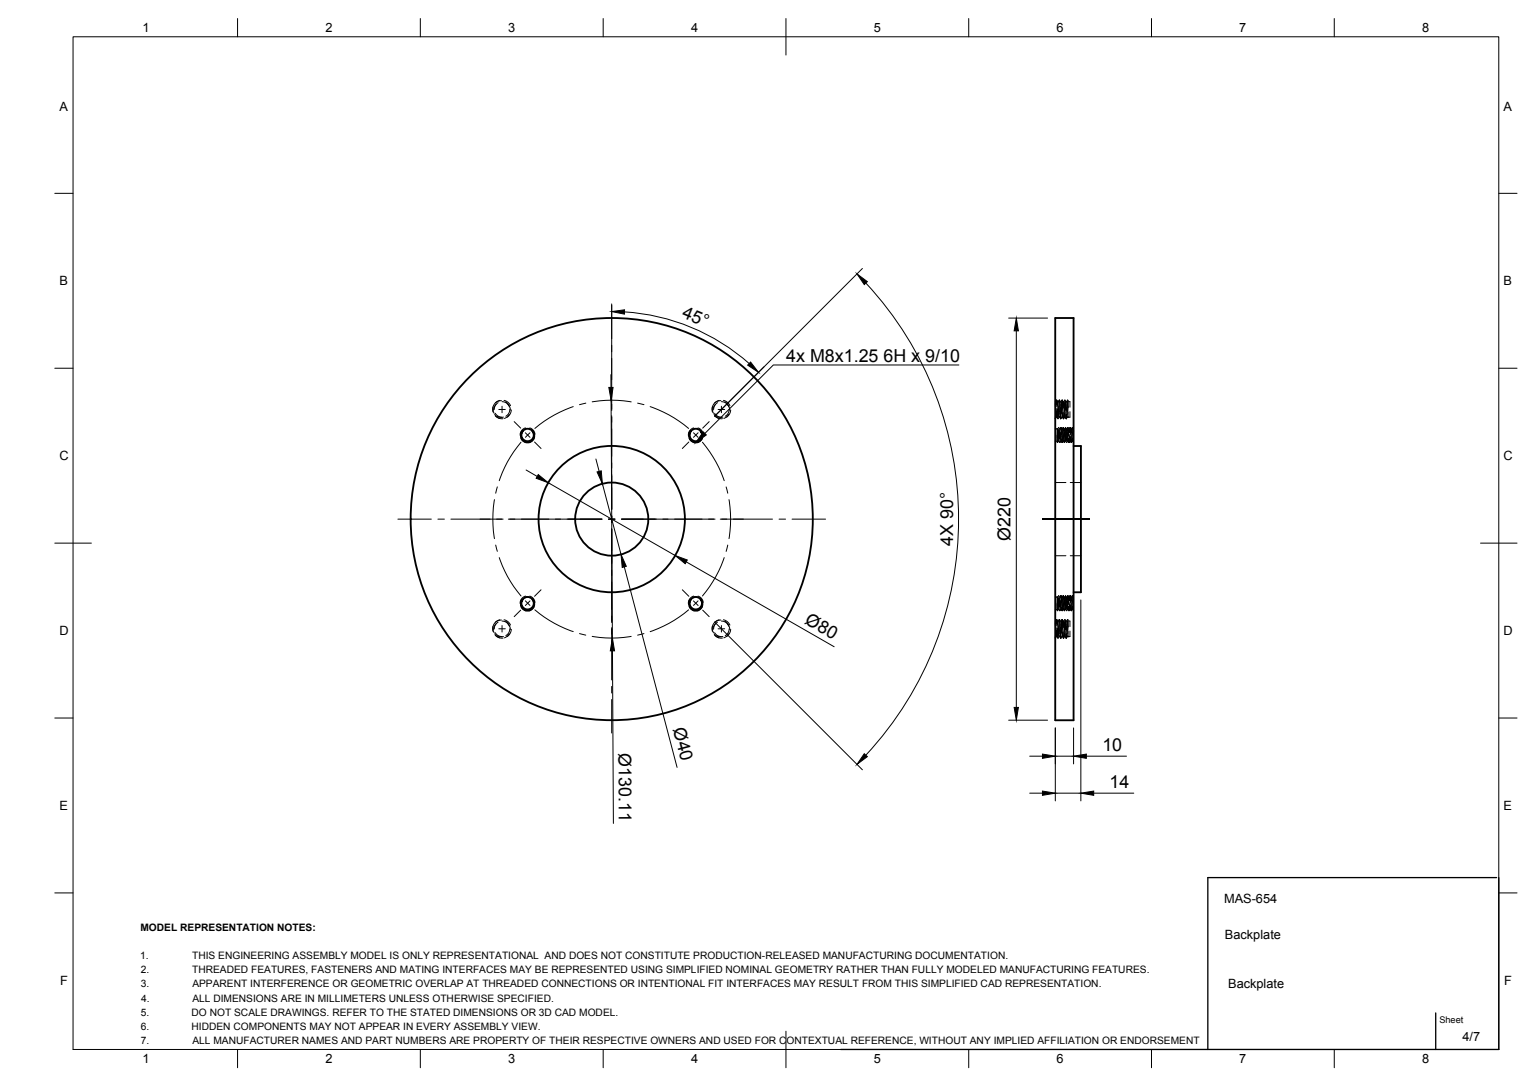
ISO-10303-21;
HEADER;
/* Generated by software containing ST-Developer
 * from STEP Tools, Inc. (www.steptools.com) 
 */

FILE_DESCRIPTION(
/* description */ ('Independent four-jaw lathe chuck,200mm body,40mm bore,36\X2\2013\X0\7
6mm nominal opposed jaw opening. Four shared machined T-jaws and model
ed partial M12x1.75 feed screws, native independent screw/slider links
, removable bolted bronze-bearing cartridges, fully captured ring/wash
er/head thrust stacks and registered bolted backplate. Custom spindle 
interface; no compatibility, speed, grip force or safety rating assign
ed.'),
/* implementation_level */ '2;1');

FILE_NAME(
/* name */ 'Backplate.step',
/* time_stamp */ '2026-11-09T20:24:54-08:00',
/* author */ (''),
/* organization */ (''),
/* preprocessor_version */ 'ST-DEVELOPER v20.2',
/* originating_system */ 'Autodesk Translation Framework v15.17.0.0',
/* authorisation */ '');

FILE_SCHEMA (('AUTOMOTIVE_DESIGN { 1 0 10303 214 3 1 1 }'));
ENDSEC;

DATA;
#10=MECHANICAL_DESIGN_GEOMETRIC_PRESENTATION_REPRESENTATION('',(#237),#69491);
#215=SHAPE_REPRESENTATION_RELATIONSHIP('SRR','None',#69572,#226);
#226=ADVANCED_BREP_SHAPE_REPRESENTATION('',(#248),#69481);
#237=STYLED_ITEM('',(#69636),#248);
#248=MANIFOLD_SOLID_BREP('Body1',#14732);
#274=B_SPLINE_SURFACE_WITH_KNOTS('',3,3,((#35745,#35746,#35747,#35748,#35749,
#35750,#35751,#35752,#35753,#35754,#35755,#35756,#35757,#35758,#35759,#35760,
#35761,#35762,#35763,#35764,#35765,#35766,#35767,#35768,#35769,#35770,#35771,
#35772,#35773,#35774,#35775,#35776,#35777,#35778,#35779,#35780,#35781,#35782,
#35783,#35784,#35785,#35786,#35787,#35788,#35789,#35790,#35791,#35792,#35793,
#35794,#35795,#35796,#35797,#35798,#35799,#35800,#35801,#35802,#35803,#35804,
#35805,#35806,#35807,#35808),(#35809,#35810,#35811,#35812,#35813,#35814,
#35815,#35816,#35817,#35818,#35819,#35820,#35821,#35822,#35823,#35824,#35825,
#35826,#35827,#35828,#35829,#35830,#35831,#35832,#35833,#35834,#35835,#35836,
#35837,#35838,#35839,#35840,#35841,#35842,#35843,#35844,#35845,#35846,#35847,
#35848,#35849,#35850,#35851,#35852,#35853,#35854,#35855,#35856,#35857,#35858,
#35859,#35860,#35861,#35862,#35863,#35864,#35865,#35866,#35867,#35868,#35869,
#35870,#35871,#35872),(#35873,#35874,#35875,#35876,#35877,#35878,#35879,
#35880,#35881,#35882,#35883,#35884,#35885,#35886,#35887,#35888,#35889,#35890,
#35891,#35892,#35893,#35894,#35895,#35896,#35897,#35898,#35899,#35900,#35901,
#35902,#35903,#35904,#35905,#35906,#35907,#35908,#35909,#35910,#35911,#35912,
#35913,#35914,#35915,#35916,#35917,#35918,#35919,#35920,#35921,#35922,#35923,
#35924,#35925,#35926,#35927,#35928,#35929,#35930,#35931,#35932,#35933,#35934,
#35935,#35936),(#35937,#35938,#35939,#35940,#35941,#35942,#35943,#35944,
#35945,#35946,#35947,#35948,#35949,#35950,#35951,#35952,#35953,#35954,#35955,
#35956,#35957,#35958,#35959,#35960,#35961,#35962,#35963,#35964,#35965,#35966,
#35967,#35968,#35969,#35970,#35971,#35972,#35973,#35974,#35975,#35976,#35977,
#35978,#35979,#35980,#35981,#35982,#35983,#35984,#35985,#35986,#35987,#35988,
#35989,#35990,#35991,#35992,#35993,#35994,#35995,#35996,#35997,#35998,#35999,
#36000)),.UNSPECIFIED.,.F.,.F.,.F.,(4,4),(4,1,1,1,1,1,1,1,1,1,1,1,1,1,1,
1,1,1,1,1,1,1,1,1,1,1,1,1,1,1,1,1,1,1,1,1,1,1,1,1,1,1,1,1,1,1,1,1,1,1,1,
1,1,1,1,1,1,1,1,1,1,4),(0.,0.0965329650085053),(11.8529428644271,12.3426821320026,
12.8324213995782,13.3221606671538,13.8118999347294,14.301639202305,14.7913784698806,
15.2811177374562,15.7708570050318,16.2605962726074,16.750335540183,17.2400748077586,
17.7298140753341,18.2195533429097,18.7092926104853,19.1990318780609,19.6887711456365,
20.1785104132121,20.6682496807877,21.1579889483633,21.6477282159389,22.1374674835145,
22.6272067510901,23.1169460186656,23.6066852862412,24.0964245538168,24.5861638213924,
25.075903088968,25.5656423565436,26.0553816241192,26.5451208916948,27.524599426846,
28.5040779619971,29.4835564971483,29.9732957647239,30.4630350322995,30.9527742998751,
31.4425135674507,31.9322528350263,32.4219921026019,32.9117313701775,33.4014706377531,
33.8912099053287,34.3809491729042,34.8706884404798,35.3604277080554,35.850166975631,
36.3399062432066,36.8296455107822,37.3193847783578,37.8091240459334,38.298863313509,
38.7886025810846,39.2783418486601,39.7680811162357,40.2578203838113,40.7475596513869,
41.2372989189625,41.7270381865381,42.2167774541137,42.7065167216893,43.1962559892649),
 .UNSPECIFIED.);
#275=B_SPLINE_SURFACE_WITH_KNOTS('',3,3,((#36150,#36151,#36152,#36153,#36154,
#36155,#36156,#36157,#36158,#36159,#36160,#36161,#36162,#36163,#36164,#36165,
#36166,#36167,#36168,#36169,#36170,#36171,#36172,#36173,#36174,#36175,#36176,
#36177,#36178,#36179,#36180,#36181,#36182,#36183,#36184,#36185,#36186,#36187,
#36188,#36189,#36190,#36191,#36192,#36193,#36194,#36195,#36196,#36197,#36198,
#36199,#36200,#36201,#36202,#36203,#36204,#36205,#36206,#36207,#36208,#36209,
#36210,#36211,#36212,#36213),(#36214,#36215,#36216,#36217,#36218,#36219,
#36220,#36221,#36222,#36223,#36224,#36225,#36226,#36227,#36228,#36229,#36230,
#36231,#36232,#36233,#36234,#36235,#36236,#36237,#36238,#36239,#36240,#36241,
#36242,#36243,#36244,#36245,#36246,#36247,#36248,#36249,#36250,#36251,#36252,
#36253,#36254,#36255,#36256,#36257,#36258,#36259,#36260,#36261,#36262,#36263,
#36264,#36265,#36266,#36267,#36268,#36269,#36270,#36271,#36272,#36273,#36274,
#36275,#36276,#36277),(#36278,#36279,#36280,#36281,#36282,#36283,#36284,
#36285,#36286,#36287,#36288,#36289,#36290,#36291,#36292,#36293,#36294,#36295,
#36296,#36297,#36298,#36299,#36300,#36301,#36302,#36303,#36304,#36305,#36306,
#36307,#36308,#36309,#36310,#36311,#36312,#36313,#36314,#36315,#36316,#36317,
#36318,#36319,#36320,#36321,#36322,#36323,#36324,#36325,#36326,#36327,#36328,
#36329,#36330,#36331,#36332,#36333,#36334,#36335,#36336,#36337,#36338,#36339,
#36340,#36341),(#36342,#36343,#36344,#36345,#36346,#36347,#36348,#36349,
#36350,#36351,#36352,#36353,#36354,#36355,#36356,#36357,#36358,#36359,#36360,
#36361,#36362,#36363,#36364,#36365,#36366,#36367,#36368,#36369,#36370,#36371,
#36372,#36373,#36374,#36375,#36376,#36377,#36378,#36379,#36380,#36381,#36382,
#36383,#36384,#36385,#36386,#36387,#36388,#36389,#36390,#36391,#36392,#36393,
#36394,#36395,#36396,#36397,#36398,#36399,#36400,#36401,#36402,#36403,#36404,
#36405)),.UNSPECIFIED.,.F.,.F.,.F.,(4,4),(4,1,1,1,1,1,1,1,1,1,1,1,1,1,1,
1,1,1,1,1,1,1,1,1,1,1,1,1,1,1,1,1,1,1,1,1,1,1,1,1,1,1,1,1,1,1,1,1,1,1,1,
1,1,1,1,1,1,1,1,1,1,4),(0.,0.0965329650085053),(14.399609326548,14.8893485941236,
15.3790878616992,15.8688271292748,16.3585663968504,16.848305664426,17.3380449320016,
17.8277841995772,18.3175234671527,18.8072627347283,19.2970020023039,19.7867412698795,
20.2764805374551,20.7662198050307,21.2559590726063,21.7456983401819,22.2354376077575,
22.7251768753331,23.2149161429087,23.7046554104842,24.1943946780598,24.6841339456354,
25.173873213211,25.6636124807866,26.1533517483622,26.6430910159378,27.1328302835134,
27.622569551089,28.1123088186646,28.6020480862402,29.0917873538157,30.0712658889669,
31.0507444241181,32.0302229592693,32.5199622268449,33.0097014944205,33.4994407619961,
33.9891800295717,34.4789192971472,34.9686585647228,35.4583978322984,35.948137099874,
36.4378763674496,36.9276156350252,37.4173549026008,37.9070941701764,38.396833437752,
38.8865727053276,39.3763119729032,39.8660512404787,40.3557905080543,40.8455297756299,
41.3352690432055,41.8250083107811,42.3147475783567,42.8044868459323,43.2942261135079,
43.7839653810835,44.2737046486591,44.7634439162347,45.2531831838103,45.7429224513858),
 .UNSPECIFIED.);
#276=B_SPLINE_SURFACE_WITH_KNOTS('',3,3,((#36810,#36811,#36812,#36813,#36814,
#36815,#36816,#36817,#36818,#36819,#36820,#36821,#36822,#36823,#36824,#36825,
#36826,#36827,#36828,#36829,#36830,#36831,#36832,#36833,#36834,#36835,#36836,
#36837,#36838,#36839,#36840,#36841,#36842,#36843,#36844,#36845,#36846,#36847,
#36848,#36849,#36850,#36851,#36852,#36853,#36854,#36855,#36856,#36857,#36858,
#36859,#36860,#36861,#36862,#36863,#36864,#36865,#36866,#36867,#36868,#36869,
#36870,#36871,#36872,#36873),(#36874,#36875,#36876,#36877,#36878,#36879,
#36880,#36881,#36882,#36883,#36884,#36885,#36886,#36887,#36888,#36889,#36890,
#36891,#36892,#36893,#36894,#36895,#36896,#36897,#36898,#36899,#36900,#36901,
#36902,#36903,#36904,#36905,#36906,#36907,#36908,#36909,#36910,#36911,#36912,
#36913,#36914,#36915,#36916,#36917,#36918,#36919,#36920,#36921,#36922,#36923,
#36924,#36925,#36926,#36927,#36928,#36929,#36930,#36931,#36932,#36933,#36934,
#36935,#36936,#36937),(#36938,#36939,#36940,#36941,#36942,#36943,#36944,
#36945,#36946,#36947,#36948,#36949,#36950,#36951,#36952,#36953,#36954,#36955,
#36956,#36957,#36958,#36959,#36960,#36961,#36962,#36963,#36964,#36965,#36966,
#36967,#36968,#36969,#36970,#36971,#36972,#36973,#36974,#36975,#36976,#36977,
#36978,#36979,#36980,#36981,#36982,#36983,#36984,#36985,#36986,#36987,#36988,
#36989,#36990,#36991,#36992,#36993,#36994,#36995,#36996,#36997,#36998,#36999,
#37000,#37001),(#37002,#37003,#37004,#37005,#37006,#37007,#37008,#37009,
#37010,#37011,#37012,#37013,#37014,#37015,#37016,#37017,#37018,#37019,#37020,
#37021,#37022,#37023,#37024,#37025,#37026,#37027,#37028,#37029,#37030,#37031,
#37032,#37033,#37034,#37035,#37036,#37037,#37038,#37039,#37040,#37041,#37042,
#37043,#37044,#37045,#37046,#37047,#37048,#37049,#37050,#37051,#37052,#37053,
#37054,#37055,#37056,#37057,#37058,#37059,#37060,#37061,#37062,#37063,#37064,
#37065)),.UNSPECIFIED.,.F.,.F.,.F.,(4,4),(4,1,1,1,1,1,1,1,1,1,1,1,1,1,1,
1,1,1,1,1,1,1,1,1,1,1,1,1,1,1,1,1,1,1,1,1,1,1,1,1,1,1,1,1,1,1,1,1,1,1,1,
1,1,1,1,1,1,1,1,1,1,4),(0.,0.0965329650085053),(11.8529428644271,12.3426821320026,
12.8324213995782,13.3221606671538,13.8118999347294,14.301639202305,14.7913784698806,
15.2811177374562,15.7708570050318,16.2605962726074,16.750335540183,17.2400748077586,
17.7298140753341,18.2195533429097,18.7092926104853,19.1990318780609,19.6887711456365,
20.1785104132121,20.6682496807877,21.1579889483633,21.6477282159389,22.1374674835145,
22.6272067510901,23.1169460186656,23.6066852862412,24.0964245538168,24.5861638213924,
25.075903088968,25.5656423565436,26.0553816241192,26.5451208916948,27.524599426846,
28.5040779619971,29.4835564971483,29.9732957647239,30.4630350322995,30.9527742998751,
31.4425135674507,31.9322528350263,32.4219921026019,32.9117313701775,33.4014706377531,
33.8912099053287,34.3809491729042,34.8706884404798,35.3604277080554,35.850166975631,
36.3399062432066,36.8296455107822,37.3193847783578,37.8091240459334,38.298863313509,
38.7886025810846,39.2783418486601,39.7680811162357,40.2578203838113,40.7475596513869,
41.2372989189625,41.7270381865381,42.2167774541137,42.7065167216893,43.1962559892649),
 .UNSPECIFIED.);
#277=B_SPLINE_SURFACE_WITH_KNOTS('',3,3,((#37215,#37216,#37217,#37218,#37219,
#37220,#37221,#37222,#37223,#37224,#37225,#37226,#37227,#37228,#37229,#37230,
#37231,#37232,#37233,#37234,#37235,#37236,#37237,#37238,#37239,#37240,#37241,
#37242,#37243,#37244,#37245,#37246,#37247,#37248,#37249,#37250,#37251,#37252,
#37253,#37254,#37255,#37256,#37257,#37258,#37259,#37260,#37261,#37262,#37263,
#37264,#37265,#37266,#37267,#37268,#37269,#37270,#37271,#37272,#37273,#37274,
#37275,#37276,#37277,#37278),(#37279,#37280,#37281,#37282,#37283,#37284,
#37285,#37286,#37287,#37288,#37289,#37290,#37291,#37292,#37293,#37294,#37295,
#37296,#37297,#37298,#37299,#37300,#37301,#37302,#37303,#37304,#37305,#37306,
#37307,#37308,#37309,#37310,#37311,#37312,#37313,#37314,#37315,#37316,#37317,
#37318,#37319,#37320,#37321,#37322,#37323,#37324,#37325,#37326,#37327,#37328,
#37329,#37330,#37331,#37332,#37333,#37334,#37335,#37336,#37337,#37338,#37339,
#37340,#37341,#37342),(#37343,#37344,#37345,#37346,#37347,#37348,#37349,
#37350,#37351,#37352,#37353,#37354,#37355,#37356,#37357,#37358,#37359,#37360,
#37361,#37362,#37363,#37364,#37365,#37366,#37367,#37368,#37369,#37370,#37371,
#37372,#37373,#37374,#37375,#37376,#37377,#37378,#37379,#37380,#37381,#37382,
#37383,#37384,#37385,#37386,#37387,#37388,#37389,#37390,#37391,#37392,#37393,
#37394,#37395,#37396,#37397,#37398,#37399,#37400,#37401,#37402,#37403,#37404,
#37405,#37406),(#37407,#37408,#37409,#37410,#37411,#37412,#37413,#37414,
#37415,#37416,#37417,#37418,#37419,#37420,#37421,#37422,#37423,#37424,#37425,
#37426,#37427,#37428,#37429,#37430,#37431,#37432,#37433,#37434,#37435,#37436,
#37437,#37438,#37439,#37440,#37441,#37442,#37443,#37444,#37445,#37446,#37447,
#37448,#37449,#37450,#37451,#37452,#37453,#37454,#37455,#37456,#37457,#37458,
#37459,#37460,#37461,#37462,#37463,#37464,#37465,#37466,#37467,#37468,#37469,
#37470)),.UNSPECIFIED.,.F.,.F.,.F.,(4,4),(4,1,1,1,1,1,1,1,1,1,1,1,1,1,1,
1,1,1,1,1,1,1,1,1,1,1,1,1,1,1,1,1,1,1,1,1,1,1,1,1,1,1,1,1,1,1,1,1,1,1,1,
1,1,1,1,1,1,1,1,1,1,4),(0.,0.0965329650085053),(14.399609326548,14.8893485941236,
15.3790878616992,15.8688271292748,16.3585663968504,16.848305664426,17.3380449320016,
17.8277841995772,18.3175234671527,18.8072627347283,19.2970020023039,19.7867412698795,
20.2764805374551,20.7662198050307,21.2559590726063,21.7456983401819,22.2354376077575,
22.7251768753331,23.2149161429087,23.7046554104842,24.1943946780598,24.6841339456354,
25.173873213211,25.6636124807866,26.1533517483622,26.6430910159378,27.1328302835134,
27.622569551089,28.1123088186646,28.6020480862402,29.0917873538157,30.0712658889669,
31.0507444241181,32.0302229592693,32.5199622268449,33.0097014944205,33.4994407619961,
33.9891800295717,34.4789192971472,34.9686585647228,35.4583978322984,35.948137099874,
36.4378763674496,36.9276156350252,37.4173549026008,37.9070941701764,38.396833437752,
38.8865727053276,39.3763119729032,39.8660512404787,40.3557905080543,40.8455297756299,
41.3352690432055,41.8250083107811,42.3147475783567,42.8044868459323,43.2942261135079,
43.7839653810835,44.2737046486591,44.7634439162347,45.2531831838103,45.7429224513858),
 .UNSPECIFIED.);
#278=B_SPLINE_SURFACE_WITH_KNOTS('',3,3,((#37875,#37876,#37877,#37878,#37879,
#37880,#37881,#37882,#37883,#37884,#37885,#37886,#37887,#37888,#37889,#37890,
#37891,#37892,#37893,#37894,#37895,#37896,#37897,#37898,#37899,#37900,#37901,
#37902,#37903,#37904,#37905,#37906,#37907,#37908,#37909,#37910,#37911,#37912,
#37913,#37914,#37915,#37916,#37917,#37918,#37919,#37920,#37921,#37922,#37923,
#37924,#37925,#37926,#37927,#37928,#37929,#37930,#37931,#37932,#37933,#37934,
#37935,#37936,#37937,#37938),(#37939,#37940,#37941,#37942,#37943,#37944,
#37945,#37946,#37947,#37948,#37949,#37950,#37951,#37952,#37953,#37954,#37955,
#37956,#37957,#37958,#37959,#37960,#37961,#37962,#37963,#37964,#37965,#37966,
#37967,#37968,#37969,#37970,#37971,#37972,#37973,#37974,#37975,#37976,#37977,
#37978,#37979,#37980,#37981,#37982,#37983,#37984,#37985,#37986,#37987,#37988,
#37989,#37990,#37991,#37992,#37993,#37994,#37995,#37996,#37997,#37998,#37999,
#38000,#38001,#38002),(#38003,#38004,#38005,#38006,#38007,#38008,#38009,
#38010,#38011,#38012,#38013,#38014,#38015,#38016,#38017,#38018,#38019,#38020,
#38021,#38022,#38023,#38024,#38025,#38026,#38027,#38028,#38029,#38030,#38031,
#38032,#38033,#38034,#38035,#38036,#38037,#38038,#38039,#38040,#38041,#38042,
#38043,#38044,#38045,#38046,#38047,#38048,#38049,#38050,#38051,#38052,#38053,
#38054,#38055,#38056,#38057,#38058,#38059,#38060,#38061,#38062,#38063,#38064,
#38065,#38066),(#38067,#38068,#38069,#38070,#38071,#38072,#38073,#38074,
#38075,#38076,#38077,#38078,#38079,#38080,#38081,#38082,#38083,#38084,#38085,
#38086,#38087,#38088,#38089,#38090,#38091,#38092,#38093,#38094,#38095,#38096,
#38097,#38098,#38099,#38100,#38101,#38102,#38103,#38104,#38105,#38106,#38107,
#38108,#38109,#38110,#38111,#38112,#38113,#38114,#38115,#38116,#38117,#38118,
#38119,#38120,#38121,#38122,#38123,#38124,#38125,#38126,#38127,#38128,#38129,
#38130)),.UNSPECIFIED.,.F.,.F.,.F.,(4,4),(4,1,1,1,1,1,1,1,1,1,1,1,1,1,1,
1,1,1,1,1,1,1,1,1,1,1,1,1,1,1,1,1,1,1,1,1,1,1,1,1,1,1,1,1,1,1,1,1,1,1,1,
1,1,1,1,1,1,1,1,1,1,4),(0.,0.0965329650085053),(11.8529428644271,12.3426821320026,
12.8324213995782,13.3221606671538,13.8118999347294,14.301639202305,14.7913784698806,
15.2811177374562,15.7708570050318,16.2605962726074,16.750335540183,17.2400748077586,
17.7298140753341,18.2195533429097,18.7092926104853,19.1990318780609,19.6887711456365,
20.1785104132121,20.6682496807877,21.1579889483633,21.6477282159389,22.1374674835145,
22.6272067510901,23.1169460186656,23.6066852862412,24.0964245538168,24.5861638213924,
25.075903088968,25.5656423565436,26.0553816241192,26.5451208916948,27.524599426846,
28.5040779619971,29.4835564971483,29.9732957647239,30.4630350322995,30.9527742998751,
31.4425135674507,31.9322528350263,32.4219921026019,32.9117313701775,33.4014706377531,
33.8912099053287,34.3809491729042,34.8706884404798,35.3604277080554,35.850166975631,
36.3399062432066,36.8296455107822,37.3193847783578,37.8091240459334,38.298863313509,
38.7886025810846,39.2783418486601,39.7680811162357,40.2578203838113,40.7475596513869,
41.2372989189625,41.7270381865381,42.2167774541137,42.7065167216893,43.1962559892649),
 .UNSPECIFIED.);
#279=B_SPLINE_SURFACE_WITH_KNOTS('',3,3,((#38280,#38281,#38282,#38283,#38284,
#38285,#38286,#38287,#38288,#38289,#38290,#38291,#38292,#38293,#38294,#38295,
#38296,#38297,#38298,#38299,#38300,#38301,#38302,#38303,#38304,#38305,#38306,
#38307,#38308,#38309,#38310,#38311,#38312,#38313,#38314,#38315,#38316,#38317,
#38318,#38319,#38320,#38321,#38322,#38323,#38324,#38325,#38326,#38327,#38328,
#38329,#38330,#38331,#38332,#38333,#38334,#38335,#38336,#38337,#38338,#38339,
#38340,#38341,#38342,#38343),(#38344,#38345,#38346,#38347,#38348,#38349,
#38350,#38351,#38352,#38353,#38354,#38355,#38356,#38357,#38358,#38359,#38360,
#38361,#38362,#38363,#38364,#38365,#38366,#38367,#38368,#38369,#38370,#38371,
#38372,#38373,#38374,#38375,#38376,#38377,#38378,#38379,#38380,#38381,#38382,
#38383,#38384,#38385,#38386,#38387,#38388,#38389,#38390,#38391,#38392,#38393,
#38394,#38395,#38396,#38397,#38398,#38399,#38400,#38401,#38402,#38403,#38404,
#38405,#38406,#38407),(#38408,#38409,#38410,#38411,#38412,#38413,#38414,
#38415,#38416,#38417,#38418,#38419,#38420,#38421,#38422,#38423,#38424,#38425,
#38426,#38427,#38428,#38429,#38430,#38431,#38432,#38433,#38434,#38435,#38436,
#38437,#38438,#38439,#38440,#38441,#38442,#38443,#38444,#38445,#38446,#38447,
#38448,#38449,#38450,#38451,#38452,#38453,#38454,#38455,#38456,#38457,#38458,
#38459,#38460,#38461,#38462,#38463,#38464,#38465,#38466,#38467,#38468,#38469,
#38470,#38471),(#38472,#38473,#38474,#38475,#38476,#38477,#38478,#38479,
#38480,#38481,#38482,#38483,#38484,#38485,#38486,#38487,#38488,#38489,#38490,
#38491,#38492,#38493,#38494,#38495,#38496,#38497,#38498,#38499,#38500,#38501,
#38502,#38503,#38504,#38505,#38506,#38507,#38508,#38509,#38510,#38511,#38512,
#38513,#38514,#38515,#38516,#38517,#38518,#38519,#38520,#38521,#38522,#38523,
#38524,#38525,#38526,#38527,#38528,#38529,#38530,#38531,#38532,#38533,#38534,
#38535)),.UNSPECIFIED.,.F.,.F.,.F.,(4,4),(4,1,1,1,1,1,1,1,1,1,1,1,1,1,1,
1,1,1,1,1,1,1,1,1,1,1,1,1,1,1,1,1,1,1,1,1,1,1,1,1,1,1,1,1,1,1,1,1,1,1,1,
1,1,1,1,1,1,1,1,1,1,4),(0.,0.0965329650085053),(14.399609326548,14.8893485941236,
15.3790878616992,15.8688271292748,16.3585663968504,16.848305664426,17.3380449320016,
17.8277841995772,18.3175234671527,18.8072627347283,19.2970020023039,19.7867412698795,
20.2764805374551,20.7662198050307,21.2559590726063,21.7456983401819,22.2354376077575,
22.7251768753331,23.2149161429087,23.7046554104842,24.1943946780598,24.6841339456354,
25.173873213211,25.6636124807866,26.1533517483622,26.6430910159378,27.1328302835134,
27.622569551089,28.1123088186646,28.6020480862402,29.0917873538157,30.0712658889669,
31.0507444241181,32.0302229592693,32.5199622268449,33.0097014944205,33.4994407619961,
33.9891800295717,34.4789192971472,34.9686585647228,35.4583978322984,35.948137099874,
36.4378763674496,36.9276156350252,37.4173549026008,37.9070941701764,38.396833437752,
38.8865727053276,39.3763119729032,39.8660512404787,40.3557905080543,40.8455297756299,
41.3352690432055,41.8250083107811,42.3147475783567,42.8044868459323,43.2942261135079,
43.7839653810835,44.2737046486591,44.7634439162347,45.2531831838103,45.7429224513858),
 .UNSPECIFIED.);
#280=B_SPLINE_SURFACE_WITH_KNOTS('',3,3,((#38940,#38941,#38942,#38943,#38944,
#38945,#38946,#38947,#38948,#38949,#38950,#38951,#38952,#38953,#38954,#38955,
#38956,#38957,#38958,#38959,#38960,#38961,#38962,#38963,#38964,#38965,#38966,
#38967,#38968,#38969,#38970,#38971,#38972,#38973,#38974,#38975,#38976,#38977,
#38978,#38979,#38980,#38981,#38982,#38983,#38984,#38985,#38986,#38987,#38988,
#38989,#38990,#38991,#38992,#38993,#38994,#38995,#38996,#38997,#38998,#38999,
#39000,#39001,#39002,#39003),(#39004,#39005,#39006,#39007,#39008,#39009,
#39010,#39011,#39012,#39013,#39014,#39015,#39016,#39017,#39018,#39019,#39020,
#39021,#39022,#39023,#39024,#39025,#39026,#39027,#39028,#39029,#39030,#39031,
#39032,#39033,#39034,#39035,#39036,#39037,#39038,#39039,#39040,#39041,#39042,
#39043,#39044,#39045,#39046,#39047,#39048,#39049,#39050,#39051,#39052,#39053,
#39054,#39055,#39056,#39057,#39058,#39059,#39060,#39061,#39062,#39063,#39064,
#39065,#39066,#39067),(#39068,#39069,#39070,#39071,#39072,#39073,#39074,
#39075,#39076,#39077,#39078,#39079,#39080,#39081,#39082,#39083,#39084,#39085,
#39086,#39087,#39088,#39089,#39090,#39091,#39092,#39093,#39094,#39095,#39096,
#39097,#39098,#39099,#39100,#39101,#39102,#39103,#39104,#39105,#39106,#39107,
#39108,#39109,#39110,#39111,#39112,#39113,#39114,#39115,#39116,#39117,#39118,
#39119,#39120,#39121,#39122,#39123,#39124,#39125,#39126,#39127,#39128,#39129,
#39130,#39131),(#39132,#39133,#39134,#39135,#39136,#39137,#39138,#39139,
#39140,#39141,#39142,#39143,#39144,#39145,#39146,#39147,#39148,#39149,#39150,
#39151,#39152,#39153,#39154,#39155,#39156,#39157,#39158,#39159,#39160,#39161,
#39162,#39163,#39164,#39165,#39166,#39167,#39168,#39169,#39170,#39171,#39172,
#39173,#39174,#39175,#39176,#39177,#39178,#39179,#39180,#39181,#39182,#39183,
#39184,#39185,#39186,#39187,#39188,#39189,#39190,#39191,#39192,#39193,#39194,
#39195)),.UNSPECIFIED.,.F.,.F.,.F.,(4,4),(4,1,1,1,1,1,1,1,1,1,1,1,1,1,1,
1,1,1,1,1,1,1,1,1,1,1,1,1,1,1,1,1,1,1,1,1,1,1,1,1,1,1,1,1,1,1,1,1,1,1,1,
1,1,1,1,1,1,1,1,1,1,4),(0.,0.0965329650085053),(11.8529428644271,12.3426821320026,
12.8324213995782,13.3221606671538,13.8118999347294,14.301639202305,14.7913784698806,
15.2811177374562,15.7708570050318,16.2605962726074,16.750335540183,17.2400748077586,
17.7298140753341,18.2195533429097,18.7092926104853,19.1990318780609,19.6887711456365,
20.1785104132121,20.6682496807877,21.1579889483633,21.6477282159389,22.1374674835145,
22.6272067510901,23.1169460186656,23.6066852862412,24.0964245538168,24.5861638213924,
25.075903088968,25.5656423565436,26.0553816241192,26.5451208916948,27.524599426846,
28.5040779619972,29.4835564971483,29.9732957647239,30.4630350322995,30.9527742998751,
31.4425135674507,31.9322528350263,32.4219921026019,32.9117313701775,33.4014706377531,
33.8912099053287,34.3809491729042,34.8706884404798,35.3604277080554,35.850166975631,
36.3399062432066,36.8296455107822,37.3193847783578,37.8091240459334,38.298863313509,
38.7886025810846,39.2783418486602,39.7680811162357,40.2578203838113,40.7475596513869,
41.2372989189625,41.7270381865381,42.2167774541137,42.7065167216893,43.1962559892649),
 .UNSPECIFIED.);
#281=B_SPLINE_SURFACE_WITH_KNOTS('',3,3,((#39345,#39346,#39347,#39348,#39349,
#39350,#39351,#39352,#39353,#39354,#39355,#39356,#39357,#39358,#39359,#39360,
#39361,#39362,#39363,#39364,#39365,#39366,#39367,#39368,#39369,#39370,#39371,
#39372,#39373,#39374,#39375,#39376,#39377,#39378,#39379,#39380,#39381,#39382,
#39383,#39384,#39385,#39386,#39387,#39388,#39389,#39390,#39391,#39392,#39393,
#39394,#39395,#39396,#39397,#39398,#39399,#39400,#39401,#39402,#39403,#39404,
#39405,#39406,#39407,#39408),(#39409,#39410,#39411,#39412,#39413,#39414,
#39415,#39416,#39417,#39418,#39419,#39420,#39421,#39422,#39423,#39424,#39425,
#39426,#39427,#39428,#39429,#39430,#39431,#39432,#39433,#39434,#39435,#39436,
#39437,#39438,#39439,#39440,#39441,#39442,#39443,#39444,#39445,#39446,#39447,
#39448,#39449,#39450,#39451,#39452,#39453,#39454,#39455,#39456,#39457,#39458,
#39459,#39460,#39461,#39462,#39463,#39464,#39465,#39466,#39467,#39468,#39469,
#39470,#39471,#39472),(#39473,#39474,#39475,#39476,#39477,#39478,#39479,
#39480,#39481,#39482,#39483,#39484,#39485,#39486,#39487,#39488,#39489,#39490,
#39491,#39492,#39493,#39494,#39495,#39496,#39497,#39498,#39499,#39500,#39501,
#39502,#39503,#39504,#39505,#39506,#39507,#39508,#39509,#39510,#39511,#39512,
#39513,#39514,#39515,#39516,#39517,#39518,#39519,#39520,#39521,#39522,#39523,
#39524,#39525,#39526,#39527,#39528,#39529,#39530,#39531,#39532,#39533,#39534,
#39535,#39536),(#39537,#39538,#39539,#39540,#39541,#39542,#39543,#39544,
#39545,#39546,#39547,#39548,#39549,#39550,#39551,#39552,#39553,#39554,#39555,
#39556,#39557,#39558,#39559,#39560,#39561,#39562,#39563,#39564,#39565,#39566,
#39567,#39568,#39569,#39570,#39571,#39572,#39573,#39574,#39575,#39576,#39577,
#39578,#39579,#39580,#39581,#39582,#39583,#39584,#39585,#39586,#39587,#39588,
#39589,#39590,#39591,#39592,#39593,#39594,#39595,#39596,#39597,#39598,#39599,
#39600)),.UNSPECIFIED.,.F.,.F.,.F.,(4,4),(4,1,1,1,1,1,1,1,1,1,1,1,1,1,1,
1,1,1,1,1,1,1,1,1,1,1,1,1,1,1,1,1,1,1,1,1,1,1,1,1,1,1,1,1,1,1,1,1,1,1,1,
1,1,1,1,1,1,1,1,1,1,4),(0.,0.0965329650085053),(14.399609326548,14.8893485941236,
15.3790878616992,15.8688271292748,16.3585663968504,16.848305664426,17.3380449320016,
17.8277841995772,18.3175234671527,18.8072627347283,19.2970020023039,19.7867412698795,
20.2764805374551,20.7662198050307,21.2559590726063,21.7456983401819,22.2354376077575,
22.7251768753331,23.2149161429087,23.7046554104842,24.1943946780598,24.6841339456354,
25.173873213211,25.6636124807866,26.1533517483622,26.6430910159378,27.1328302835134,
27.622569551089,28.1123088186646,28.6020480862402,29.0917873538157,30.0712658889669,
31.0507444241181,32.0302229592693,32.5199622268449,33.0097014944205,33.4994407619961,
33.9891800295717,34.4789192971472,34.9686585647228,35.4583978322984,35.948137099874,
36.4378763674496,36.9276156350252,37.4173549026008,37.9070941701764,38.396833437752,
38.8865727053276,39.3763119729032,39.8660512404787,40.3557905080543,40.8455297756299,
41.3352690432055,41.8250083107811,42.3147475783567,42.8044868459323,43.2942261135079,
43.7839653810835,44.2737046486591,44.7634439162347,45.2531831838103,45.7429224513858),
 .UNSPECIFIED.);
#282=B_SPLINE_SURFACE_WITH_KNOTS('',3,3,((#39975,#39976,#39977,#39978,#39979,
#39980,#39981,#39982,#39983,#39984,#39985,#39986,#39987,#39988,#39989,#39990,
#39991,#39992,#39993,#39994,#39995,#39996,#39997,#39998,#39999,#40000,#40001,
#40002,#40003,#40004,#40005,#40006,#40007,#40008,#40009,#40010,#40011,#40012,
#40013,#40014,#40015,#40016,#40017,#40018,#40019,#40020,#40021,#40022,#40023,
#40024,#40025),(#40026,#40027,#40028,#40029,#40030,#40031,#40032,#40033,
#40034,#40035,#40036,#40037,#40038,#40039,#40040,#40041,#40042,#40043,#40044,
#40045,#40046,#40047,#40048,#40049,#40050,#40051,#40052,#40053,#40054,#40055,
#40056,#40057,#40058,#40059,#40060,#40061,#40062,#40063,#40064,#40065,#40066,
#40067,#40068,#40069,#40070,#40071,#40072,#40073,#40074,#40075,#40076),
(#40077,#40078,#40079,#40080,#40081,#40082,#40083,#40084,#40085,#40086,
#40087,#40088,#40089,#40090,#40091,#40092,#40093,#40094,#40095,#40096,#40097,
#40098,#40099,#40100,#40101,#40102,#40103,#40104,#40105,#40106,#40107,#40108,
#40109,#40110,#40111,#40112,#40113,#40114,#40115,#40116,#40117,#40118,#40119,
#40120,#40121,#40122,#40123,#40124,#40125,#40126,#40127),(#40128,#40129,
#40130,#40131,#40132,#40133,#40134,#40135,#40136,#40137,#40138,#40139,#40140,
#40141,#40142,#40143,#40144,#40145,#40146,#40147,#40148,#40149,#40150,#40151,
#40152,#40153,#40154,#40155,#40156,#40157,#40158,#40159,#40160,#40161,#40162,
#40163,#40164,#40165,#40166,#40167,#40168,#40169,#40170,#40171,#40172,#40173,
#40174,#40175,#40176,#40177,#40178)),.UNSPECIFIED.,.F.,.F.,.F.,(4,4),(4,
1,1,1,1,1,1,1,1,1,1,1,1,1,1,1,1,1,1,1,1,1,1,1,1,1,1,1,1,1,1,1,1,1,1,1,1,
1,1,1,1,1,1,1,1,1,1,1,4),(0.,0.0802805549308171),(11.8575378228164,12.8420504191595,
13.8265630155026,14.8110756118456,15.7955882081887,16.7801008045318,17.7646134008748,
18.7491259972179,19.733638593561,20.718151189904,21.7026637862471,22.6871763825902,
23.6716889789332,24.6562015752763,25.6407141716194,26.6252267679624,27.6097393643055,
28.5942519606485,29.5787645569916,30.5632771533347,31.5477897496777,32.5323023460208,
33.5168149423639,34.5013275387069,35.48584013505,36.4703527313931,37.4548653277361,
38.4393779240792,39.4238905204223,40.4084031167653,41.3929157131084,42.3774283094515,
43.3619409057945,44.3464535021376,45.3309660984807,46.3154786948237,47.2999912911668,
48.2845038875099,49.2690164838529,50.253529080196,51.2380416765391,52.2225542728821,
53.2070668692252,54.1915794655683,55.1760920619113,56.1606046582544,57.1451172545975,
58.1296298509405,59.1141424472836),.UNSPECIFIED.);
#283=B_SPLINE_SURFACE_WITH_KNOTS('',3,3,((#40298,#40299,#40300,#40301,#40302,
#40303,#40304,#40305,#40306,#40307,#40308,#40309,#40310,#40311,#40312,#40313,
#40314,#40315,#40316,#40317,#40318,#40319,#40320,#40321,#40322,#40323,#40324,
#40325,#40326,#40327,#40328,#40329,#40330,#40331,#40332,#40333,#40334,#40335,
#40336,#40337,#40338,#40339,#40340,#40341,#40342,#40343,#40344,#40345,#40346,
#40347,#40348),(#40349,#40350,#40351,#40352,#40353,#40354,#40355,#40356,
#40357,#40358,#40359,#40360,#40361,#40362,#40363,#40364,#40365,#40366,#40367,
#40368,#40369,#40370,#40371,#40372,#40373,#40374,#40375,#40376,#40377,#40378,
#40379,#40380,#40381,#40382,#40383,#40384,#40385,#40386,#40387,#40388,#40389,
#40390,#40391,#40392,#40393,#40394,#40395,#40396,#40397,#40398,#40399),
(#40400,#40401,#40402,#40403,#40404,#40405,#40406,#40407,#40408,#40409,
#40410,#40411,#40412,#40413,#40414,#40415,#40416,#40417,#40418,#40419,#40420,
#40421,#40422,#40423,#40424,#40425,#40426,#40427,#40428,#40429,#40430,#40431,
#40432,#40433,#40434,#40435,#40436,#40437,#40438,#40439,#40440,#40441,#40442,
#40443,#40444,#40445,#40446,#40447,#40448,#40449,#40450),(#40451,#40452,
#40453,#40454,#40455,#40456,#40457,#40458,#40459,#40460,#40461,#40462,#40463,
#40464,#40465,#40466,#40467,#40468,#40469,#40470,#40471,#40472,#40473,#40474,
#40475,#40476,#40477,#40478,#40479,#40480,#40481,#40482,#40483,#40484,#40485,
#40486,#40487,#40488,#40489,#40490,#40491,#40492,#40493,#40494,#40495,#40496,
#40497,#40498,#40499,#40500,#40501)),.UNSPECIFIED.,.F.,.F.,.F.,(4,4),(4,
1,1,1,1,1,1,1,1,1,1,1,1,1,1,1,1,1,1,1,1,1,1,1,1,1,1,1,1,1,1,1,1,1,1,1,1,
1,1,1,1,1,1,1,1,1,1,1,4),(0.,0.0802805549308171),(14.3991256467175,15.3836382430606,
16.3681508394037,17.3526634357467,18.3371760320898,19.3216886284329,20.3062012247759,
21.290713821119,22.2752264174621,23.2597390138051,24.2442516101482,25.2287642064913,
26.2132768028343,27.1977893991774,28.1823019955205,29.1668145918635,30.1513271882066,
31.1358397845497,32.1203523808927,33.1048649772358,34.0893775735789,35.0738901699219,
36.058402766265,37.0429153626081,38.0274279589511,39.0119405552942,39.9964531516373,
40.9809657479803,41.9654783443234,42.9499909406665,43.9345035370095,44.9190161333526,
45.9035287296957,46.8880413260387,47.8725539223818,48.8570665187248,49.8415791150679,
50.826091711411,51.810604307754,52.7951169040971,53.7796295004402,54.7641420967832,
55.7486546931263,56.7331672894694,57.7176798858124,58.7021924821555,59.6867050784986,
60.6712176748416,61.6557302711847),.UNSPECIFIED.);
#284=B_SPLINE_SURFACE_WITH_KNOTS('',3,3,((#40848,#40849,#40850,#40851,#40852,
#40853,#40854,#40855,#40856,#40857,#40858,#40859,#40860,#40861,#40862,#40863,
#40864,#40865,#40866,#40867,#40868,#40869,#40870,#40871,#40872,#40873,#40874,
#40875,#40876,#40877,#40878,#40879,#40880,#40881,#40882,#40883,#40884,#40885,
#40886,#40887,#40888,#40889,#40890,#40891,#40892,#40893,#40894,#40895,#40896,
#40897,#40898),(#40899,#40900,#40901,#40902,#40903,#40904,#40905,#40906,
#40907,#40908,#40909,#40910,#40911,#40912,#40913,#40914,#40915,#40916,#40917,
#40918,#40919,#40920,#40921,#40922,#40923,#40924,#40925,#40926,#40927,#40928,
#40929,#40930,#40931,#40932,#40933,#40934,#40935,#40936,#40937,#40938,#40939,
#40940,#40941,#40942,#40943,#40944,#40945,#40946,#40947,#40948,#40949),
(#40950,#40951,#40952,#40953,#40954,#40955,#40956,#40957,#40958,#40959,
#40960,#40961,#40962,#40963,#40964,#40965,#40966,#40967,#40968,#40969,#40970,
#40971,#40972,#40973,#40974,#40975,#40976,#40977,#40978,#40979,#40980,#40981,
#40982,#40983,#40984,#40985,#40986,#40987,#40988,#40989,#40990,#40991,#40992,
#40993,#40994,#40995,#40996,#40997,#40998,#40999,#41000),(#41001,#41002,
#41003,#41004,#41005,#41006,#41007,#41008,#41009,#41010,#41011,#41012,#41013,
#41014,#41015,#41016,#41017,#41018,#41019,#41020,#41021,#41022,#41023,#41024,
#41025,#41026,#41027,#41028,#41029,#41030,#41031,#41032,#41033,#41034,#41035,
#41036,#41037,#41038,#41039,#41040,#41041,#41042,#41043,#41044,#41045,#41046,
#41047,#41048,#41049,#41050,#41051)),.UNSPECIFIED.,.F.,.F.,.F.,(4,4),(4,
1,1,1,1,1,1,1,1,1,1,1,1,1,1,1,1,1,1,1,1,1,1,1,1,1,1,1,1,1,1,1,1,1,1,1,1,
1,1,1,1,1,1,1,1,1,1,1,4),(0.,0.0802805549308171),(11.8575378228164,12.8420504191595,
13.8265630155026,14.8110756118456,15.7955882081887,16.7801008045318,17.7646134008748,
18.7491259972179,19.733638593561,20.718151189904,21.7026637862471,22.6871763825901,
23.6716889789332,24.6562015752763,25.6407141716193,26.6252267679624,27.6097393643055,
28.5942519606485,29.5787645569916,30.5632771533347,31.5477897496777,32.5323023460208,
33.5168149423639,34.5013275387069,35.48584013505,36.4703527313931,37.4548653277361,
38.4393779240792,39.4238905204223,40.4084031167653,41.3929157131084,42.3774283094515,
43.3619409057945,44.3464535021376,45.3309660984807,46.3154786948237,47.2999912911668,
48.2845038875099,49.2690164838529,50.253529080196,51.2380416765391,52.2225542728821,
53.2070668692252,54.1915794655683,55.1760920619113,56.1606046582544,57.1451172545975,
58.1296298509405,59.1141424472836),.UNSPECIFIED.);
#285=B_SPLINE_SURFACE_WITH_KNOTS('',3,3,((#41171,#41172,#41173,#41174,#41175,
#41176,#41177,#41178,#41179,#41180,#41181,#41182,#41183,#41184,#41185,#41186,
#41187,#41188,#41189,#41190,#41191,#41192,#41193,#41194,#41195,#41196,#41197,
#41198,#41199,#41200,#41201,#41202,#41203,#41204,#41205,#41206,#41207,#41208,
#41209,#41210,#41211,#41212,#41213,#41214,#41215,#41216,#41217,#41218,#41219,
#41220,#41221),(#41222,#41223,#41224,#41225,#41226,#41227,#41228,#41229,
#41230,#41231,#41232,#41233,#41234,#41235,#41236,#41237,#41238,#41239,#41240,
#41241,#41242,#41243,#41244,#41245,#41246,#41247,#41248,#41249,#41250,#41251,
#41252,#41253,#41254,#41255,#41256,#41257,#41258,#41259,#41260,#41261,#41262,
#41263,#41264,#41265,#41266,#41267,#41268,#41269,#41270,#41271,#41272),
(#41273,#41274,#41275,#41276,#41277,#41278,#41279,#41280,#41281,#41282,
#41283,#41284,#41285,#41286,#41287,#41288,#41289,#41290,#41291,#41292,#41293,
#41294,#41295,#41296,#41297,#41298,#41299,#41300,#41301,#41302,#41303,#41304,
#41305,#41306,#41307,#41308,#41309,#41310,#41311,#41312,#41313,#41314,#41315,
#41316,#41317,#41318,#41319,#41320,#41321,#41322,#41323),(#41324,#41325,
#41326,#41327,#41328,#41329,#41330,#41331,#41332,#41333,#41334,#41335,#41336,
#41337,#41338,#41339,#41340,#41341,#41342,#41343,#41344,#41345,#41346,#41347,
#41348,#41349,#41350,#41351,#41352,#41353,#41354,#41355,#41356,#41357,#41358,
#41359,#41360,#41361,#41362,#41363,#41364,#41365,#41366,#41367,#41368,#41369,
#41370,#41371,#41372,#41373,#41374)),.UNSPECIFIED.,.F.,.F.,.F.,(4,4),(4,
1,1,1,1,1,1,1,1,1,1,1,1,1,1,1,1,1,1,1,1,1,1,1,1,1,1,1,1,1,1,1,1,1,1,1,1,
1,1,1,1,1,1,1,1,1,1,1,4),(0.,0.0802805549308171),(14.3991256467175,15.3836382430606,
16.3681508394037,17.3526634357467,18.3371760320898,19.3216886284329,20.3062012247759,
21.290713821119,22.2752264174621,23.2597390138051,24.2442516101482,25.2287642064913,
26.2132768028343,27.1977893991774,28.1823019955205,29.1668145918635,30.1513271882066,
31.1358397845497,32.1203523808927,33.1048649772358,34.0893775735789,35.0738901699219,
36.058402766265,37.0429153626081,38.0274279589511,39.0119405552942,39.9964531516373,
40.9809657479803,41.9654783443234,42.9499909406665,43.9345035370095,44.9190161333526,
45.9035287296957,46.8880413260387,47.8725539223818,48.8570665187248,49.8415791150679,
50.826091711411,51.810604307754,52.7951169040971,53.7796295004402,54.7641420967832,
55.7486546931263,56.7331672894694,57.7176798858124,58.7021924821555,59.6867050784986,
60.6712176748416,61.6557302711847),.UNSPECIFIED.);
#286=B_SPLINE_SURFACE_WITH_KNOTS('',3,3,((#41721,#41722,#41723,#41724,#41725,
#41726,#41727,#41728,#41729,#41730,#41731,#41732,#41733,#41734,#41735,#41736,
#41737,#41738,#41739,#41740,#41741,#41742,#41743,#41744,#41745,#41746,#41747,
#41748,#41749,#41750,#41751,#41752,#41753,#41754,#41755,#41756,#41757,#41758,
#41759,#41760,#41761,#41762,#41763,#41764,#41765,#41766,#41767,#41768,#41769,
#41770,#41771),(#41772,#41773,#41774,#41775,#41776,#41777,#41778,#41779,
#41780,#41781,#41782,#41783,#41784,#41785,#41786,#41787,#41788,#41789,#41790,
#41791,#41792,#41793,#41794,#41795,#41796,#41797,#41798,#41799,#41800,#41801,
#41802,#41803,#41804,#41805,#41806,#41807,#41808,#41809,#41810,#41811,#41812,
#41813,#41814,#41815,#41816,#41817,#41818,#41819,#41820,#41821,#41822),
(#41823,#41824,#41825,#41826,#41827,#41828,#41829,#41830,#41831,#41832,
#41833,#41834,#41835,#41836,#41837,#41838,#41839,#41840,#41841,#41842,#41843,
#41844,#41845,#41846,#41847,#41848,#41849,#41850,#41851,#41852,#41853,#41854,
#41855,#41856,#41857,#41858,#41859,#41860,#41861,#41862,#41863,#41864,#41865,
#41866,#41867,#41868,#41869,#41870,#41871,#41872,#41873),(#41874,#41875,
#41876,#41877,#41878,#41879,#41880,#41881,#41882,#41883,#41884,#41885,#41886,
#41887,#41888,#41889,#41890,#41891,#41892,#41893,#41894,#41895,#41896,#41897,
#41898,#41899,#41900,#41901,#41902,#41903,#41904,#41905,#41906,#41907,#41908,
#41909,#41910,#41911,#41912,#41913,#41914,#41915,#41916,#41917,#41918,#41919,
#41920,#41921,#41922,#41923,#41924)),.UNSPECIFIED.,.F.,.F.,.F.,(4,4),(4,
1,1,1,1,1,1,1,1,1,1,1,1,1,1,1,1,1,1,1,1,1,1,1,1,1,1,1,1,1,1,1,1,1,1,1,1,
1,1,1,1,1,1,1,1,1,1,1,4),(0.,0.0802805549308171),(11.8575378228164,12.8420504191595,
13.8265630155026,14.8110756118456,15.7955882081887,16.7801008045318,17.7646134008748,
18.7491259972179,19.733638593561,20.718151189904,21.7026637862471,22.6871763825901,
23.6716889789332,24.6562015752763,25.6407141716193,26.6252267679624,27.6097393643055,
28.5942519606485,29.5787645569916,30.5632771533347,31.5477897496777,32.5323023460208,
33.5168149423639,34.5013275387069,35.48584013505,36.4703527313931,37.4548653277361,
38.4393779240792,39.4238905204223,40.4084031167653,41.3929157131084,42.3774283094515,
43.3619409057945,44.3464535021376,45.3309660984807,46.3154786948237,47.2999912911668,
48.2845038875099,49.2690164838529,50.253529080196,51.2380416765391,52.2225542728821,
53.2070668692252,54.1915794655683,55.1760920619113,56.1606046582544,57.1451172545975,
58.1296298509405,59.1141424472836),.UNSPECIFIED.);
#287=B_SPLINE_SURFACE_WITH_KNOTS('',3,3,((#42044,#42045,#42046,#42047,#42048,
#42049,#42050,#42051,#42052,#42053,#42054,#42055,#42056,#42057,#42058,#42059,
#42060,#42061,#42062,#42063,#42064,#42065,#42066,#42067,#42068,#42069,#42070,
#42071,#42072,#42073,#42074,#42075,#42076,#42077,#42078,#42079,#42080,#42081,
#42082,#42083,#42084,#42085,#42086,#42087,#42088,#42089,#42090,#42091,#42092,
#42093,#42094),(#42095,#42096,#42097,#42098,#42099,#42100,#42101,#42102,
#42103,#42104,#42105,#42106,#42107,#42108,#42109,#42110,#42111,#42112,#42113,
#42114,#42115,#42116,#42117,#42118,#42119,#42120,#42121,#42122,#42123,#42124,
#42125,#42126,#42127,#42128,#42129,#42130,#42131,#42132,#42133,#42134,#42135,
#42136,#42137,#42138,#42139,#42140,#42141,#42142,#42143,#42144,#42145),
(#42146,#42147,#42148,#42149,#42150,#42151,#42152,#42153,#42154,#42155,
#42156,#42157,#42158,#42159,#42160,#42161,#42162,#42163,#42164,#42165,#42166,
#42167,#42168,#42169,#42170,#42171,#42172,#42173,#42174,#42175,#42176,#42177,
#42178,#42179,#42180,#42181,#42182,#42183,#42184,#42185,#42186,#42187,#42188,
#42189,#42190,#42191,#42192,#42193,#42194,#42195,#42196),(#42197,#42198,
#42199,#42200,#42201,#42202,#42203,#42204,#42205,#42206,#42207,#42208,#42209,
#42210,#42211,#42212,#42213,#42214,#42215,#42216,#42217,#42218,#42219,#42220,
#42221,#42222,#42223,#42224,#42225,#42226,#42227,#42228,#42229,#42230,#42231,
#42232,#42233,#42234,#42235,#42236,#42237,#42238,#42239,#42240,#42241,#42242,
#42243,#42244,#42245,#42246,#42247)),.UNSPECIFIED.,.F.,.F.,.F.,(4,4),(4,
1,1,1,1,1,1,1,1,1,1,1,1,1,1,1,1,1,1,1,1,1,1,1,1,1,1,1,1,1,1,1,1,1,1,1,1,
1,1,1,1,1,1,1,1,1,1,1,4),(0.,0.0802805549308171),(14.3991256467175,15.3836382430606,
16.3681508394037,17.3526634357467,18.3371760320898,19.3216886284329,20.3062012247759,
21.290713821119,22.2752264174621,23.2597390138051,24.2442516101482,25.2287642064913,
26.2132768028343,27.1977893991774,28.1823019955205,29.1668145918635,30.1513271882066,
31.1358397845496,32.1203523808927,33.1048649772358,34.0893775735788,35.0738901699219,
36.058402766265,37.042915362608,38.0274279589511,39.0119405552942,39.9964531516372,
40.9809657479803,41.9654783443234,42.9499909406664,43.9345035370095,44.9190161333526,
45.9035287296956,46.8880413260387,47.8725539223818,48.8570665187248,49.8415791150679,
50.826091711411,51.810604307754,52.7951169040971,53.7796295004402,54.7641420967832,
55.7486546931263,56.7331672894694,57.7176798858124,58.7021924821555,59.6867050784986,
60.6712176748416,61.6557302711847),.UNSPECIFIED.);
#288=B_SPLINE_SURFACE_WITH_KNOTS('',3,3,((#42594,#42595,#42596,#42597,#42598,
#42599,#42600,#42601,#42602,#42603,#42604,#42605,#42606,#42607,#42608,#42609,
#42610,#42611,#42612,#42613,#42614,#42615,#42616,#42617,#42618,#42619,#42620,
#42621,#42622,#42623,#42624,#42625,#42626,#42627,#42628,#42629,#42630,#42631,
#42632,#42633,#42634,#42635,#42636,#42637,#42638,#42639,#42640,#42641,#42642,
#42643,#42644),(#42645,#42646,#42647,#42648,#42649,#42650,#42651,#42652,
#42653,#42654,#42655,#42656,#42657,#42658,#42659,#42660,#42661,#42662,#42663,
#42664,#42665,#42666,#42667,#42668,#42669,#42670,#42671,#42672,#42673,#42674,
#42675,#42676,#42677,#42678,#42679,#42680,#42681,#42682,#42683,#42684,#42685,
#42686,#42687,#42688,#42689,#42690,#42691,#42692,#42693,#42694,#42695),
(#42696,#42697,#42698,#42699,#42700,#42701,#42702,#42703,#42704,#42705,
#42706,#42707,#42708,#42709,#42710,#42711,#42712,#42713,#42714,#42715,#42716,
#42717,#42718,#42719,#42720,#42721,#42722,#42723,#42724,#42725,#42726,#42727,
#42728,#42729,#42730,#42731,#42732,#42733,#42734,#42735,#42736,#42737,#42738,
#42739,#42740,#42741,#42742,#42743,#42744,#42745,#42746),(#42747,#42748,
#42749,#42750,#42751,#42752,#42753,#42754,#42755,#42756,#42757,#42758,#42759,
#42760,#42761,#42762,#42763,#42764,#42765,#42766,#42767,#42768,#42769,#42770,
#42771,#42772,#42773,#42774,#42775,#42776,#42777,#42778,#42779,#42780,#42781,
#42782,#42783,#42784,#42785,#42786,#42787,#42788,#42789,#42790,#42791,#42792,
#42793,#42794,#42795,#42796,#42797)),.UNSPECIFIED.,.F.,.F.,.F.,(4,4),(4,
1,1,1,1,1,1,1,1,1,1,1,1,1,1,1,1,1,1,1,1,1,1,1,1,1,1,1,1,1,1,1,1,1,1,1,1,
1,1,1,1,1,1,1,1,1,1,1,4),(0.,0.0802805549308171),(11.8575378228164,12.8420504191595,
13.8265630155026,14.8110756118456,15.7955882081887,16.7801008045318,17.7646134008748,
18.7491259972179,19.733638593561,20.718151189904,21.7026637862471,22.6871763825901,
23.6716889789332,24.6562015752763,25.6407141716193,26.6252267679624,27.6097393643055,
28.5942519606485,29.5787645569916,30.5632771533347,31.5477897496777,32.5323023460208,
33.5168149423639,34.5013275387069,35.48584013505,36.4703527313931,37.4548653277361,
38.4393779240792,39.4238905204223,40.4084031167653,41.3929157131084,42.3774283094515,
43.3619409057945,44.3464535021376,45.3309660984807,46.3154786948237,47.2999912911668,
48.2845038875099,49.2690164838529,50.253529080196,51.2380416765391,52.2225542728821,
53.2070668692252,54.1915794655683,55.1760920619113,56.1606046582544,57.1451172545975,
58.1296298509405,59.1141424472836),.UNSPECIFIED.);
#289=B_SPLINE_SURFACE_WITH_KNOTS('',3,3,((#42917,#42918,#42919,#42920,#42921,
#42922,#42923,#42924,#42925,#42926,#42927,#42928,#42929,#42930,#42931,#42932,
#42933,#42934,#42935,#42936,#42937,#42938,#42939,#42940,#42941,#42942,#42943,
#42944,#42945,#42946,#42947,#42948,#42949,#42950,#42951,#42952,#42953,#42954,
#42955,#42956,#42957,#42958,#42959,#42960,#42961,#42962,#42963,#42964,#42965,
#42966,#42967),(#42968,#42969,#42970,#42971,#42972,#42973,#42974,#42975,
#42976,#42977,#42978,#42979,#42980,#42981,#42982,#42983,#42984,#42985,#42986,
#42987,#42988,#42989,#42990,#42991,#42992,#42993,#42994,#42995,#42996,#42997,
#42998,#42999,#43000,#43001,#43002,#43003,#43004,#43005,#43006,#43007,#43008,
#43009,#43010,#43011,#43012,#43013,#43014,#43015,#43016,#43017,#43018),
(#43019,#43020,#43021,#43022,#43023,#43024,#43025,#43026,#43027,#43028,
#43029,#43030,#43031,#43032,#43033,#43034,#43035,#43036,#43037,#43038,#43039,
#43040,#43041,#43042,#43043,#43044,#43045,#43046,#43047,#43048,#43049,#43050,
#43051,#43052,#43053,#43054,#43055,#43056,#43057,#43058,#43059,#43060,#43061,
#43062,#43063,#43064,#43065,#43066,#43067,#43068,#43069),(#43070,#43071,
#43072,#43073,#43074,#43075,#43076,#43077,#43078,#43079,#43080,#43081,#43082,
#43083,#43084,#43085,#43086,#43087,#43088,#43089,#43090,#43091,#43092,#43093,
#43094,#43095,#43096,#43097,#43098,#43099,#43100,#43101,#43102,#43103,#43104,
#43105,#43106,#43107,#43108,#43109,#43110,#43111,#43112,#43113,#43114,#43115,
#43116,#43117,#43118,#43119,#43120)),.UNSPECIFIED.,.F.,.F.,.F.,(4,4),(4,
1,1,1,1,1,1,1,1,1,1,1,1,1,1,1,1,1,1,1,1,1,1,1,1,1,1,1,1,1,1,1,1,1,1,1,1,
1,1,1,1,1,1,1,1,1,1,1,4),(0.,0.0802805549308171),(14.3991256467175,15.3836382430606,
16.3681508394037,17.3526634357467,18.3371760320898,19.3216886284329,20.3062012247759,
21.290713821119,22.2752264174621,23.2597390138051,24.2442516101482,25.2287642064913,
26.2132768028343,27.1977893991774,28.1823019955205,29.1668145918635,30.1513271882066,
31.1358397845497,32.1203523808927,33.1048649772358,34.0893775735789,35.0738901699219,
36.058402766265,37.0429153626081,38.0274279589511,39.0119405552942,39.9964531516373,
40.9809657479803,41.9654783443234,42.9499909406665,43.9345035370095,44.9190161333526,
45.9035287296957,46.8880413260387,47.8725539223818,48.8570665187248,49.8415791150679,
50.826091711411,51.810604307754,52.7951169040971,53.7796295004402,54.7641420967832,
55.7486546931263,56.7331672894694,57.7176798858124,58.7021924821555,59.6867050784986,
60.6712176748416,61.6557302711847),.UNSPECIFIED.);
#328=FACE_BOUND('',#1728,.T.);
#329=FACE_BOUND('',#1732,.T.);
#330=FACE_BOUND('',#1733,.T.);
#331=FACE_BOUND('',#1734,.T.);
#332=FACE_BOUND('',#1735,.T.);
#333=FACE_BOUND('',#1736,.T.);
#334=FACE_BOUND('',#1738,.T.);
#335=FACE_BOUND('',#1739,.T.);
#336=FACE_BOUND('',#1740,.T.);
#337=FACE_BOUND('',#1741,.T.);
#338=FACE_BOUND('',#1742,.T.);
#339=FACE_BOUND('',#1743,.T.);
#340=FACE_BOUND('',#1744,.T.);
#341=FACE_BOUND('',#1745,.T.);
#342=FACE_BOUND('',#1746,.T.);
#435=PLANE('',#15330);
#436=PLANE('',#15333);
#437=PLANE('',#15336);
#438=PLANE('',#15339);
#439=PLANE('',#15342);
#440=PLANE('',#15343);
#441=PLANE('',#15344);
#442=PLANE('',#15345);
#443=PLANE('',#15346);
#444=PLANE('',#15349);
#445=PLANE('',#15352);
#446=PLANE('',#15355);
#447=PLANE('',#15361);
#448=PLANE('',#15368);
#449=PLANE('',#15369);
#779=FACE_OUTER_BOUND('',#1590,.T.);
#780=FACE_OUTER_BOUND('',#1591,.T.);
#781=FACE_OUTER_BOUND('',#1592,.T.);
#782=FACE_OUTER_BOUND('',#1593,.T.);
#783=FACE_OUTER_BOUND('',#1594,.T.);
#784=FACE_OUTER_BOUND('',#1595,.T.);
#785=FACE_OUTER_BOUND('',#1596,.T.);
#786=FACE_OUTER_BOUND('',#1597,.T.);
#787=FACE_OUTER_BOUND('',#1598,.T.);
#788=FACE_OUTER_BOUND('',#1599,.T.);
#789=FACE_OUTER_BOUND('',#1600,.T.);
#790=FACE_OUTER_BOUND('',#1601,.T.);
#791=FACE_OUTER_BOUND('',#1602,.T.);
#792=FACE_OUTER_BOUND('',#1603,.T.);
#793=FACE_OUTER_BOUND('',#1604,.T.);
#794=FACE_OUTER_BOUND('',#1605,.T.);
#795=FACE_OUTER_BOUND('',#1606,.T.);
#796=FACE_OUTER_BOUND('',#1607,.T.);
#797=FACE_OUTER_BOUND('',#1608,.T.);
#798=FACE_OUTER_BOUND('',#1609,.T.);
#799=FACE_OUTER_BOUND('',#1610,.T.);
#800=FACE_OUTER_BOUND('',#1611,.T.);
#801=FACE_OUTER_BOUND('',#1612,.T.);
#802=FACE_OUTER_BOUND('',#1613,.T.);
#803=FACE_OUTER_BOUND('',#1614,.T.);
#804=FACE_OUTER_BOUND('',#1615,.T.);
#805=FACE_OUTER_BOUND('',#1616,.T.);
#806=FACE_OUTER_BOUND('',#1617,.T.);
#807=FACE_OUTER_BOUND('',#1618,.T.);
#808=FACE_OUTER_BOUND('',#1619,.T.);
#809=FACE_OUTER_BOUND('',#1620,.T.);
#810=FACE_OUTER_BOUND('',#1621,.T.);
#811=FACE_OUTER_BOUND('',#1622,.T.);
#812=FACE_OUTER_BOUND('',#1623,.T.);
#813=FACE_OUTER_BOUND('',#1624,.T.);
#814=FACE_OUTER_BOUND('',#1625,.T.);
#815=FACE_OUTER_BOUND('',#1626,.T.);
#816=FACE_OUTER_BOUND('',#1627,.T.);
#817=FACE_OUTER_BOUND('',#1628,.T.);
#818=FACE_OUTER_BOUND('',#1629,.T.);
#819=FACE_OUTER_BOUND('',#1630,.T.);
#820=FACE_OUTER_BOUND('',#1631,.T.);
#821=FACE_OUTER_BOUND('',#1632,.T.);
#822=FACE_OUTER_BOUND('',#1633,.T.);
#823=FACE_OUTER_BOUND('',#1634,.T.);
#824=FACE_OUTER_BOUND('',#1635,.T.);
#825=FACE_OUTER_BOUND('',#1636,.T.);
#826=FACE_OUTER_BOUND('',#1637,.T.);
#827=FACE_OUTER_BOUND('',#1638,.T.);
#828=FACE_OUTER_BOUND('',#1639,.T.);
#829=FACE_OUTER_BOUND('',#1640,.T.);
#830=FACE_OUTER_BOUND('',#1641,.T.);
#831=FACE_OUTER_BOUND('',#1642,.T.);
#832=FACE_OUTER_BOUND('',#1643,.T.);
#833=FACE_OUTER_BOUND('',#1644,.T.);
#834=FACE_OUTER_BOUND('',#1645,.T.);
#835=FACE_OUTER_BOUND('',#1646,.T.);
#836=FACE_OUTER_BOUND('',#1647,.T.);
#837=FACE_OUTER_BOUND('',#1648,.T.);
#838=FACE_OUTER_BOUND('',#1649,.T.);
#839=FACE_OUTER_BOUND('',#1650,.T.);
#840=FACE_OUTER_BOUND('',#1651,.T.);
#841=FACE_OUTER_BOUND('',#1652,.T.);
#842=FACE_OUTER_BOUND('',#1653,.T.);
#843=FACE_OUTER_BOUND('',#1654,.T.);
#844=FACE_OUTER_BOUND('',#1655,.T.);
#845=FACE_OUTER_BOUND('',#1656,.T.);
#846=FACE_OUTER_BOUND('',#1657,.T.);
#847=FACE_OUTER_BOUND('',#1658,.T.);
#848=FACE_OUTER_BOUND('',#1659,.T.);
#849=FACE_OUTER_BOUND('',#1660,.T.);
#850=FACE_OUTER_BOUND('',#1661,.T.);
#851=FACE_OUTER_BOUND('',#1662,.T.);
#852=FACE_OUTER_BOUND('',#1663,.T.);
#853=FACE_OUTER_BOUND('',#1664,.T.);
#854=FACE_OUTER_BOUND('',#1665,.T.);
#855=FACE_OUTER_BOUND('',#1666,.T.);
#856=FACE_OUTER_BOUND('',#1667,.T.);
#857=FACE_OUTER_BOUND('',#1668,.T.);
#858=FACE_OUTER_BOUND('',#1669,.T.);
#859=FACE_OUTER_BOUND('',#1670,.T.);
#860=FACE_OUTER_BOUND('',#1671,.T.);
#861=FACE_OUTER_BOUND('',#1672,.T.);
#862=FACE_OUTER_BOUND('',#1673,.T.);
#863=FACE_OUTER_BOUND('',#1674,.T.);
#864=FACE_OUTER_BOUND('',#1675,.T.);
#865=FACE_OUTER_BOUND('',#1676,.T.);
#866=FACE_OUTER_BOUND('',#1677,.T.);
#867=FACE_OUTER_BOUND('',#1678,.T.);
#868=FACE_OUTER_BOUND('',#1679,.T.);
#869=FACE_OUTER_BOUND('',#1680,.T.);
#870=FACE_OUTER_BOUND('',#1681,.T.);
#871=FACE_OUTER_BOUND('',#1682,.T.);
#872=FACE_OUTER_BOUND('',#1683,.T.);
#873=FACE_OUTER_BOUND('',#1684,.T.);
#874=FACE_OUTER_BOUND('',#1685,.T.);
#875=FACE_OUTER_BOUND('',#1686,.T.);
#876=FACE_OUTER_BOUND('',#1687,.T.);
#877=FACE_OUTER_BOUND('',#1688,.T.);
#878=FACE_OUTER_BOUND('',#1689,.T.);
#879=FACE_OUTER_BOUND('',#1690,.T.);
#880=FACE_OUTER_BOUND('',#1691,.T.);
#881=FACE_OUTER_BOUND('',#1692,.T.);
#882=FACE_OUTER_BOUND('',#1693,.T.);
#883=FACE_OUTER_BOUND('',#1694,.T.);
#884=FACE_OUTER_BOUND('',#1695,.T.);
#885=FACE_OUTER_BOUND('',#1696,.T.);
#886=FACE_OUTER_BOUND('',#1697,.T.);
#887=FACE_OUTER_BOUND('',#1698,.T.);
#888=FACE_OUTER_BOUND('',#1699,.T.);
#889=FACE_OUTER_BOUND('',#1700,.T.);
#890=FACE_OUTER_BOUND('',#1701,.T.);
#891=FACE_OUTER_BOUND('',#1702,.T.);
#892=FACE_OUTER_BOUND('',#1703,.T.);
#893=FACE_OUTER_BOUND('',#1704,.T.);
#894=FACE_OUTER_BOUND('',#1705,.T.);
#895=FACE_OUTER_BOUND('',#1706,.T.);
#896=FACE_OUTER_BOUND('',#1707,.T.);
#897=FACE_OUTER_BOUND('',#1708,.T.);
#898=FACE_OUTER_BOUND('',#1709,.T.);
#899=FACE_OUTER_BOUND('',#1710,.T.);
#900=FACE_OUTER_BOUND('',#1711,.T.);
#901=FACE_OUTER_BOUND('',#1712,.T.);
#902=FACE_OUTER_BOUND('',#1713,.T.);
#903=FACE_OUTER_BOUND('',#1714,.T.);
#904=FACE_OUTER_BOUND('',#1715,.T.);
#905=FACE_OUTER_BOUND('',#1716,.T.);
#906=FACE_OUTER_BOUND('',#1717,.T.);
#907=FACE_OUTER_BOUND('',#1718,.T.);
#908=FACE_OUTER_BOUND('',#1719,.T.);
#909=FACE_OUTER_BOUND('',#1720,.T.);
#910=FACE_OUTER_BOUND('',#1721,.T.);
#911=FACE_OUTER_BOUND('',#1722,.T.);
#912=FACE_OUTER_BOUND('',#1723,.T.);
#913=FACE_OUTER_BOUND('',#1724,.T.);
#914=FACE_OUTER_BOUND('',#1725,.T.);
#915=FACE_OUTER_BOUND('',#1726,.T.);
#916=FACE_OUTER_BOUND('',#1727,.T.);
#917=FACE_OUTER_BOUND('',#1729,.T.);
#918=FACE_OUTER_BOUND('',#1730,.T.);
#919=FACE_OUTER_BOUND('',#1731,.T.);
#920=FACE_OUTER_BOUND('',#1737,.T.);
#1590=EDGE_LOOP('',(#10427,#10428,#10429,#10430,#10431,#10432,#10433,#10434));
#1591=EDGE_LOOP('',(#10435,#10436,#10437,#10438));
#1592=EDGE_LOOP('',(#10439,#10440,#10441,#10442));
#1593=EDGE_LOOP('',(#10443,#10444,#10445,#10446));
#1594=EDGE_LOOP('',(#10447,#10448,#10449,#10450));
#1595=EDGE_LOOP('',(#10451,#10452,#10453,#10454));
#1596=EDGE_LOOP('',(#10455,#10456,#10457,#10458));
#1597=EDGE_LOOP('',(#10459,#10460,#10461,#10462));
#1598=EDGE_LOOP('',(#10463,#10464,#10465,#10466));
#1599=EDGE_LOOP('',(#10467,#10468,#10469,#10470));
#1600=EDGE_LOOP('',(#10471,#10472,#10473,#10474));
#1601=EDGE_LOOP('',(#10475,#10476,#10477,#10478));
#1602=EDGE_LOOP('',(#10479,#10480,#10481,#10482));
#1603=EDGE_LOOP('',(#10483,#10484,#10485,#10486));
#1604=EDGE_LOOP('',(#10487,#10488,#10489,#10490,#10491,#10492,#10493,#10494));
#1605=EDGE_LOOP('',(#10495,#10496,#10497,#10498));
#1606=EDGE_LOOP('',(#10499,#10500,#10501,#10502));
#1607=EDGE_LOOP('',(#10503,#10504,#10505,#10506));
#1608=EDGE_LOOP('',(#10507,#10508,#10509,#10510));
#1609=EDGE_LOOP('',(#10511,#10512,#10513,#10514));
#1610=EDGE_LOOP('',(#10515,#10516,#10517,#10518));
#1611=EDGE_LOOP('',(#10519,#10520,#10521,#10522));
#1612=EDGE_LOOP('',(#10523,#10524,#10525,#10526));
#1613=EDGE_LOOP('',(#10527,#10528,#10529,#10530));
#1614=EDGE_LOOP('',(#10531,#10532,#10533,#10534));
#1615=EDGE_LOOP('',(#10535,#10536,#10537,#10538));
#1616=EDGE_LOOP('',(#10539,#10540,#10541,#10542));
#1617=EDGE_LOOP('',(#10543,#10544,#10545,#10546));
#1618=EDGE_LOOP('',(#10547,#10548,#10549,#10550,#10551,#10552,#10553,#10554));
#1619=EDGE_LOOP('',(#10555,#10556,#10557,#10558));
#1620=EDGE_LOOP('',(#10559,#10560,#10561,#10562));
#1621=EDGE_LOOP('',(#10563,#10564,#10565,#10566));
#1622=EDGE_LOOP('',(#10567,#10568,#10569,#10570));
#1623=EDGE_LOOP('',(#10571,#10572,#10573,#10574));
#1624=EDGE_LOOP('',(#10575,#10576,#10577,#10578));
#1625=EDGE_LOOP('',(#10579,#10580,#10581,#10582));
#1626=EDGE_LOOP('',(#10583,#10584,#10585,#10586));
#1627=EDGE_LOOP('',(#10587,#10588,#10589,#10590));
#1628=EDGE_LOOP('',(#10591,#10592,#10593,#10594));
#1629=EDGE_LOOP('',(#10595,#10596,#10597,#10598));
#1630=EDGE_LOOP('',(#10599,#10600,#10601,#10602));
#1631=EDGE_LOOP('',(#10603,#10604,#10605,#10606));
#1632=EDGE_LOOP('',(#10607,#10608,#10609,#10610,#10611,#10612,#10613,#10614));
#1633=EDGE_LOOP('',(#10615,#10616,#10617,#10618));
#1634=EDGE_LOOP('',(#10619,#10620,#10621,#10622));
#1635=EDGE_LOOP('',(#10623,#10624,#10625,#10626));
#1636=EDGE_LOOP('',(#10627,#10628,#10629,#10630));
#1637=EDGE_LOOP('',(#10631,#10632,#10633,#10634));
#1638=EDGE_LOOP('',(#10635,#10636,#10637,#10638));
#1639=EDGE_LOOP('',(#10639,#10640,#10641,#10642));
#1640=EDGE_LOOP('',(#10643,#10644,#10645,#10646));
#1641=EDGE_LOOP('',(#10647,#10648,#10649,#10650));
#1642=EDGE_LOOP('',(#10651,#10652,#10653,#10654));
#1643=EDGE_LOOP('',(#10655,#10656,#10657,#10658));
#1644=EDGE_LOOP('',(#10659,#10660,#10661,#10662));
#1645=EDGE_LOOP('',(#10663,#10664,#10665,#10666));
#1646=EDGE_LOOP('',(#10667,#10668,#10669,#10670,#10671,#10672,#10673,#10674));
#1647=EDGE_LOOP('',(#10675,#10676,#10677,#10678));
#1648=EDGE_LOOP('',(#10679,#10680,#10681,#10682));
#1649=EDGE_LOOP('',(#10683,#10684,#10685,#10686));
#1650=EDGE_LOOP('',(#10687,#10688,#10689,#10690));
#1651=EDGE_LOOP('',(#10691,#10692,#10693,#10694));
#1652=EDGE_LOOP('',(#10695,#10696,#10697,#10698));
#1653=EDGE_LOOP('',(#10699,#10700,#10701,#10702));
#1654=EDGE_LOOP('',(#10703,#10704,#10705,#10706));
#1655=EDGE_LOOP('',(#10707,#10708,#10709,#10710,#10711,#10712,#10713,#10714));
#1656=EDGE_LOOP('',(#10715,#10716,#10717,#10718));
#1657=EDGE_LOOP('',(#10719,#10720,#10721,#10722));
#1658=EDGE_LOOP('',(#10723,#10724,#10725,#10726));
#1659=EDGE_LOOP('',(#10727,#10728,#10729,#10730));
#1660=EDGE_LOOP('',(#10731,#10732,#10733,#10734));
#1661=EDGE_LOOP('',(#10735,#10736,#10737,#10738));
#1662=EDGE_LOOP('',(#10739,#10740,#10741,#10742));
#1663=EDGE_LOOP('',(#10743,#10744,#10745,#10746));
#1664=EDGE_LOOP('',(#10747,#10748,#10749,#10750,#10751,#10752,#10753,#10754));
#1665=EDGE_LOOP('',(#10755,#10756,#10757,#10758));
#1666=EDGE_LOOP('',(#10759,#10760,#10761,#10762));
#1667=EDGE_LOOP('',(#10763,#10764,#10765,#10766));
#1668=EDGE_LOOP('',(#10767,#10768,#10769,#10770));
#1669=EDGE_LOOP('',(#10771,#10772,#10773,#10774));
#1670=EDGE_LOOP('',(#10775,#10776,#10777,#10778));
#1671=EDGE_LOOP('',(#10779,#10780,#10781,#10782));
#1672=EDGE_LOOP('',(#10783,#10784,#10785,#10786));
#1673=EDGE_LOOP('',(#10787,#10788,#10789,#10790,#10791,#10792,#10793,#10794));
#1674=EDGE_LOOP('',(#10795,#10796,#10797,#10798));
#1675=EDGE_LOOP('',(#10799,#10800,#10801,#10802));
#1676=EDGE_LOOP('',(#10803,#10804,#10805,#10806));
#1677=EDGE_LOOP('',(#10807,#10808,#10809,#10810));
#1678=EDGE_LOOP('',(#10811,#10812,#10813,#10814));
#1679=EDGE_LOOP('',(#10815,#10816,#10817,#10818));
#1680=EDGE_LOOP('',(#10819,#10820,#10821,#10822));
#1681=EDGE_LOOP('',(#10823,#10824,#10825,#10826));
#1682=EDGE_LOOP('',(#10827,#10828,#10829,#10830));
#1683=EDGE_LOOP('',(#10831,#10832,#10833,#10834));
#1684=EDGE_LOOP('',(#10835,#10836,#10837,#10838,#10839,#10840,#10841,#10842,
#10843,#10844,#10845,#10846,#10847,#10848));
#1685=EDGE_LOOP('',(#10849,#10850,#10851,#10852,#10853,#10854,#10855,#10856,
#10857,#10858,#10859,#10860,#10861));
#1686=EDGE_LOOP('',(#10862,#10863,#10864,#10865));
#1687=EDGE_LOOP('',(#10866,#10867,#10868,#10869));
#1688=EDGE_LOOP('',(#10870,#10871,#10872,#10873));
#1689=EDGE_LOOP('',(#10874,#10875,#10876,#10877,#10878,#10879,#10880,#10881,
#10882,#10883,#10884,#10885,#10886,#10887));
#1690=EDGE_LOOP('',(#10888,#10889,#10890,#10891,#10892,#10893,#10894,#10895,
#10896,#10897,#10898,#10899,#10900));
#1691=EDGE_LOOP('',(#10901,#10902,#10903,#10904));
#1692=EDGE_LOOP('',(#10905,#10906,#10907,#10908));
#1693=EDGE_LOOP('',(#10909,#10910,#10911,#10912));
#1694=EDGE_LOOP('',(#10913,#10914,#10915,#10916,#10917,#10918,#10919,#10920,
#10921,#10922,#10923,#10924,#10925,#10926));
#1695=EDGE_LOOP('',(#10927,#10928,#10929,#10930,#10931,#10932,#10933,#10934,
#10935,#10936,#10937,#10938,#10939));
#1696=EDGE_LOOP('',(#10940,#10941,#10942,#10943));
#1697=EDGE_LOOP('',(#10944,#10945,#10946,#10947));
#1698=EDGE_LOOP('',(#10948,#10949,#10950,#10951));
#1699=EDGE_LOOP('',(#10952,#10953,#10954,#10955,#10956,#10957,#10958,#10959,
#10960,#10961,#10962,#10963,#10964,#10965));
#1700=EDGE_LOOP('',(#10966,#10967,#10968,#10969,#10970,#10971,#10972,#10973,
#10974,#10975,#10976,#10977,#10978));
#1701=EDGE_LOOP('',(#10979,#10980,#10981,#10982));
#1702=EDGE_LOOP('',(#10983));
#1703=EDGE_LOOP('',(#10984));
#1704=EDGE_LOOP('',(#10985));
#1705=EDGE_LOOP('',(#10986));
#1706=EDGE_LOOP('',(#10987,#10988,#10989,#10990,#10991));
#1707=EDGE_LOOP('',(#10992,#10993,#10994,#10995));
#1708=EDGE_LOOP('',(#10996,#10997,#10998,#10999,#11000,#11001,#11002,#11003,
#11004,#11005,#11006,#11007,#11008,#11009,#11010,#11011,#11012,#11013));
#1709=EDGE_LOOP('',(#11014,#11015,#11016,#11017,#11018,#11019,#11020,#11021,
#11022,#11023,#11024,#11025,#11026,#11027,#11028,#11029,#11030,#11031));
#1710=EDGE_LOOP('',(#11032,#11033,#11034,#11035));
#1711=EDGE_LOOP('',(#11036,#11037,#11038,#11039,#11040));
#1712=EDGE_LOOP('',(#11041,#11042,#11043,#11044));
#1713=EDGE_LOOP('',(#11045,#11046,#11047,#11048,#11049,#11050,#11051,#11052,
#11053,#11054,#11055,#11056,#11057,#11058,#11059,#11060,#11061,#11062));
#1714=EDGE_LOOP('',(#11063,#11064,#11065,#11066,#11067,#11068,#11069,#11070,
#11071,#11072,#11073,#11074,#11075,#11076,#11077,#11078,#11079,#11080));
#1715=EDGE_LOOP('',(#11081,#11082,#11083,#11084));
#1716=EDGE_LOOP('',(#11085,#11086,#11087,#11088,#11089));
#1717=EDGE_LOOP('',(#11090,#11091,#11092,#11093));
#1718=EDGE_LOOP('',(#11094,#11095,#11096,#11097,#11098,#11099,#11100,#11101,
#11102,#11103,#11104,#11105,#11106,#11107,#11108,#11109,#11110,#11111));
#1719=EDGE_LOOP('',(#11112,#11113,#11114,#11115,#11116,#11117,#11118,#11119,
#11120,#11121,#11122,#11123,#11124,#11125,#11126,#11127,#11128,#11129));
#1720=EDGE_LOOP('',(#11130,#11131,#11132,#11133));
#1721=EDGE_LOOP('',(#11134,#11135,#11136,#11137,#11138));
#1722=EDGE_LOOP('',(#11139,#11140,#11141,#11142));
#1723=EDGE_LOOP('',(#11143,#11144,#11145,#11146,#11147,#11148,#11149,#11150,
#11151,#11152,#11153,#11154,#11155,#11156,#11157,#11158,#11159,#11160));
#1724=EDGE_LOOP('',(#11161,#11162,#11163,#11164,#11165,#11166,#11167,#11168,
#11169,#11170,#11171,#11172,#11173,#11174,#11175,#11176,#11177,#11178));
#1725=EDGE_LOOP('',(#11179,#11180,#11181,#11182));
#1726=EDGE_LOOP('',(#11183,#11184,#11185,#11186));
#1727=EDGE_LOOP('',(#11187));
#1728=EDGE_LOOP('',(#11188));
#1729=EDGE_LOOP('',(#11189,#11190,#11191,#11192));
#1730=EDGE_LOOP('',(#11193,#11194,#11195,#11196));
#1731=EDGE_LOOP('',(#11197));
#1732=EDGE_LOOP('',(#11198,#11199,#11200,#11201));
#1733=EDGE_LOOP('',(#11202,#11203,#11204,#11205));
#1734=EDGE_LOOP('',(#11206,#11207,#11208,#11209));
#1735=EDGE_LOOP('',(#11210,#11211,#11212,#11213));
#1736=EDGE_LOOP('',(#11214));
#1737=EDGE_LOOP('',(#11215));
#1738=EDGE_LOOP('',(#11216,#11217,#11218,#11219));
#1739=EDGE_LOOP('',(#11220,#11221,#11222,#11223));
#1740=EDGE_LOOP('',(#11224));
#1741=EDGE_LOOP('',(#11225));
#1742=EDGE_LOOP('',(#11226));
#1743=EDGE_LOOP('',(#11227));
#1744=EDGE_LOOP('',(#11228));
#1745=EDGE_LOOP('',(#11229,#11230,#11231,#11232));
#1746=EDGE_LOOP('',(#11233,#11234,#11235,#11236));
#2237=CIRCLE('',#15195,3.38975);
#2238=CIRCLE('',#15196,3.38975);
#2239=CIRCLE('',#15197,3.38975);
#2240=CIRCLE('',#15204,3.38975);
#2241=CIRCLE('',#15206,4.085);
#2242=CIRCLE('',#15213,4.085);
#2243=CIRCLE('',#15215,3.38975);
#2244=CIRCLE('',#15216,3.38975);
#2245=CIRCLE('',#15217,3.38975);
#2246=CIRCLE('',#15224,3.38975);
#2247=CIRCLE('',#15226,4.085);
#2248=CIRCLE('',#15233,4.085);
#2249=CIRCLE('',#15235,3.38975);
#2250=CIRCLE('',#15236,3.38975);
#2251=CIRCLE('',#15237,3.38975);
#2252=CIRCLE('',#15244,3.38975);
#2253=CIRCLE('',#15246,4.085);
#2254=CIRCLE('',#15253,4.085);
#2255=CIRCLE('',#15255,3.38975);
#2256=CIRCLE('',#15256,3.38975);
#2257=CIRCLE('',#15257,3.38975);
#2258=CIRCLE('',#15264,3.38975);
#2259=CIRCLE('',#15266,4.085);
#2260=CIRCLE('',#15273,4.085);
#2261=CIRCLE('',#15275,4.263);
#2262=CIRCLE('',#15276,4.263);
#2263=CIRCLE('',#15280,4.263);
#2264=CIRCLE('',#15282,5.099);
#2265=CIRCLE('',#15287,5.099);
#2266=CIRCLE('',#15289,4.263);
#2267=CIRCLE('',#15290,4.263);
#2268=CIRCLE('',#15294,4.263);
#2269=CIRCLE('',#15296,5.099);
#2270=CIRCLE('',#15301,5.099);
#2271=CIRCLE('',#15303,4.263);
#2272=CIRCLE('',#15304,4.263);
#2273=CIRCLE('',#15308,4.263);
#2274=CIRCLE('',#15310,5.099);
#2275=CIRCLE('',#15315,5.099);
#2276=CIRCLE('',#15317,4.263);
#2277=CIRCLE('',#15318,4.263);
#2278=CIRCLE('',#15322,4.263);
#2279=CIRCLE('',#15324,5.099);
#2280=CIRCLE('',#15329,5.099);
#2281=CIRCLE('',#15359,40.);
#2282=CIRCLE('',#15360,40.);
#2283=CIRCLE('',#15362,20.);
#2284=CIRCLE('',#15364,20.);
#2285=CIRCLE('',#15366,110.);
#2286=CIRCLE('',#15367,110.);
#2699=B_SPLINE_CURVE_WITH_KNOTS('',3,(#31645,#31646,#31647,#31648,#31649,
#31650,#31651),.UNSPECIFIED.,.F.,.F.,(4,3,4),(45.2911347714885,46.2720920281241,
47.2566046244672),.UNSPECIFIED.);
#2700=B_SPLINE_CURVE_WITH_KNOTS('',3,(#31659,#31660,#31661,#31662,#31663,
#31664,#31665,#31666,#31667,#31668,#31669,#31670,#31671),.UNSPECIFIED.,
 .F.,.F.,(4,3,3,3,4),(-45.238934211693,-44.303066835438,-43.3185542390949,
-42.3340416427518,-41.5495372882101),.UNSPECIFIED.);
#2701=B_SPLINE_CURVE_WITH_KNOTS('',3,(#31676,#31677,#31678,#31679,#31680,
#31681,#31682,#31683,#31684,#31685,#31686,#31687,#31688,#31689,#31690,#31691,
#31692,#31693,#31694,#31695,#31696,#31697,#31698,#31699,#31700),
 .UNSPECIFIED.,.F.,.F.,(4,3,3,3,3,3,3,3,4),(39.0079494643089,39.3805038537227,
40.3650164500657,41.3495290464088,42.3340416427518,43.3185542390949,44.303066835438,
45.287579431781,45.2911347714885),.UNSPECIFIED.);
#2702=B_SPLINE_CURVE_WITH_KNOTS('',3,(#31701,#31702,#31703,#31704,#31705,
#31706,#31707,#31708,#31709,#31710,#31711,#31712,#31713,#31714,#31715,#31716,
#31717,#31718,#31719,#31720,#31721,#31722,#31723,#31724,#31725),
 .UNSPECIFIED.,.F.,.F.,(4,3,3,3,3,3,3,3,4),(-41.5495372882101,-41.3495290464088,
-40.3650164500657,-39.3805038537227,-38.3959912573796,-37.4114786610365,
-36.4269660646935,-35.4424534683504,-35.2663519810305),.UNSPECIFIED.);
#2703=B_SPLINE_CURVE_WITH_KNOTS('',3,(#31730,#31731,#31732,#31733,#31734,
#31735,#31736,#31737,#31738,#31739,#31740,#31741,#31742,#31743,#31744,#31745,
#31746,#31747,#31748,#31749,#31750,#31751),.UNSPECIFIED.,.F.,.F.,(4,3,3,
3,3,3,3,4),(32.7247641571293,33.4734282756643,34.4579408720073,35.4424534683504,
36.4269660646935,37.4114786610365,38.3959912573796,39.0079494643089),
 .UNSPECIFIED.);
#2704=B_SPLINE_CURVE_WITH_KNOTS('',3,(#31752,#31753,#31754,#31755,#31756,
#31757,#31758,#31759,#31760,#31761,#31762,#31763,#31764,#31765,#31766,#31767,
#31768,#31769,#31770,#31771,#31772,#31773),.UNSPECIFIED.,.F.,.F.,(4,3,3,
3,3,3,3,4),(-35.2663519810305,-34.4579408720073,-33.4734282756643,-32.4889156793212,
-31.5044030829781,-30.5198904866351,-29.535377890292,-28.9831666738509),
 .UNSPECIFIED.);
#2705=B_SPLINE_CURVE_WITH_KNOTS('',3,(#31778,#31779,#31780,#31781,#31782,
#31783,#31784,#31785,#31786,#31787,#31788,#31789,#31790,#31791,#31792,#31793,
#31794,#31795,#31796,#31797,#31798,#31799,#31800,#31801,#31802),
 .UNSPECIFIED.,.F.,.F.,(4,3,3,3,3,3,3,3,4),(26.4415788499498,26.5818401012628,
27.5663526976059,28.5508652939489,29.535377890292,30.5198904866351,31.5044030829781,
32.4889156793212,32.7247641571293),.UNSPECIFIED.);
#2706=B_SPLINE_CURVE_WITH_KNOTS('',3,(#31803,#31804,#31805,#31806,#31807,
#31808,#31809,#31810,#31811,#31812,#31813,#31814,#31815,#31816,#31817,#31818,
#31819,#31820,#31821,#31822,#31823,#31824),.UNSPECIFIED.,.F.,.F.,(4,3,3,
3,3,3,3,4),(-28.9831666738509,-28.5508652939489,-27.5663526976059,-26.5818401012628,
-25.5973275049197,-24.6128149085767,-23.6283023122336,-22.6999813666713),
 .UNSPECIFIED.);
#2707=B_SPLINE_CURVE_WITH_KNOTS('',3,(#31829,#31830,#31831,#31832,#31833,
#31834,#31835,#31836,#31837,#31838,#31839,#31840,#31841,#31842,#31843,#31844,
#31845,#31846,#31847,#31848,#31849,#31850),.UNSPECIFIED.,.F.,.F.,(4,3,3,
3,3,3,3,4),(20.1583935427702,20.6747645232044,21.6592771195475,22.6437897158905,
23.6283023122336,24.6128149085767,25.5973275049197,26.4415788499498),
 .UNSPECIFIED.);
#2708=B_SPLINE_CURVE_WITH_KNOTS('',3,(#31851,#31852,#31853,#31854,#31855,
#31856,#31857,#31858,#31859,#31860,#31861,#31862,#31863,#31864,#31865,#31866,
#31867,#31868,#31869,#31870,#31871,#31872,#31873,#31874,#31875),
 .UNSPECIFIED.,.F.,.F.,(4,3,3,3,3,3,3,3,4),(-22.6999813666713,-22.6437897158905,
-21.6592771195475,-20.6747645232044,-19.6902519268613,-18.7057393305183,
-17.7212267341752,-16.7367141378321,-16.4167960594917),.UNSPECIFIED.);
#2709=B_SPLINE_CURVE_WITH_KNOTS('',3,(#31880,#31881,#31882,#31883,#31884,
#31885,#31886,#31887,#31888,#31889,#31890,#31891,#31892,#31893,#31894,#31895,
#31896,#31897,#31898,#31899,#31900,#31901),.UNSPECIFIED.,.F.,.F.,(4,3,3,
3,3,3,3,4),(13.8752082355906,14.767688945146,15.7522015414891,16.7367141378321,
17.7212267341752,18.7057393305183,19.6902519268613,20.1583935427702),
 .UNSPECIFIED.);
#2710=B_SPLINE_CURVE_WITH_KNOTS('',3,(#31902,#31903,#31904,#31905,#31906,
#31907,#31908,#31909,#31910,#31911,#31912,#31913,#31914,#31915,#31916,#31917,
#31918,#31919,#31920,#31921,#31922,#31923),.UNSPECIFIED.,.F.,.F.,(4,3,3,
3,3,3,3,4),(-16.4167960594917,-15.7522015414891,-14.767688945146,-13.7831763488029,
-12.7986637524599,-11.8141511561168,-10.8296385597737,-10.1336107523121),
 .UNSPECIFIED.);
#2711=B_SPLINE_CURVE_WITH_KNOTS('',3,(#31929,#31930,#31931,#31932,#31933,
#31934,#31935,#31936,#31937,#31938,#31939,#31940,#31941),.UNSPECIFIED.,
 .F.,.F.,(4,3,3,3,4),(-3.85042544513253,-2.9535377890292,-1.96902519268613,
-0.984512596343067,0.),.UNSPECIFIED.);
#2712=B_SPLINE_CURVE_WITH_KNOTS('',3,(#31944,#31945,#31946,#31947,#31948,
#31949,#31950,#31951,#31952,#31953,#31954,#31955,#31956,#31957,#31958,#31959,
#31960,#31961,#31962),.UNSPECIFIED.,.F.,.F.,(4,3,3,3,3,3,4),(2.01767041277416,
2.9535377890292,3.93805038537227,4.92256298171533,5.9070755780584,6.89158817440147,
7.592022928411),.UNSPECIFIED.);
#2713=B_SPLINE_CURVE_WITH_KNOTS('',3,(#31968,#31969,#31970,#31971,#31972,
#31973,#31974,#31975,#31976),.UNSPECIFIED.,.F.,.F.,(4,1,1,1,1,1,4),(53.4070751110265,
54.1915794655683,55.1760920619113,56.1606046582544,57.1451172545975,58.1296298509405,
59.1141424472836),.UNSPECIFIED.);
#2714=B_SPLINE_CURVE_WITH_KNOTS('',3,(#31979,#31980,#31981,#31982,#31983,
#31984,#31985,#31986,#31987,#31988),.UNSPECIFIED.,.F.,.F.,(4,1,1,1,1,1,
1,4),(53.4070751110265,53.7796295004402,54.7641420967832,55.7486546931263,
56.7331672894694,57.7176798858124,58.7021924821555,59.6380598584106),
 .UNSPECIFIED.);
#2715=B_SPLINE_CURVE_WITH_KNOTS('',3,(#31993,#31994,#31995,#31996,#31997,
#31998,#31999,#32000,#32001,#32002,#32003),.UNSPECIFIED.,.F.,.F.,(4,1,1,
1,1,1,1,1,4),(47.1238898038469,47.2999912911668,48.2845038875099,49.2690164838529,
50.253529080196,51.2380416765391,52.2225542728821,53.2070668692252,53.4070751110265),
 .UNSPECIFIED.);
#2716=B_SPLINE_CURVE_WITH_KNOTS('',3,(#32004,#32005,#32006,#32007,#32008,
#32009,#32010,#32011,#32012,#32013),.UNSPECIFIED.,.F.,.F.,(4,1,1,1,1,1,
1,4),(47.1238898038469,47.8725539223818,48.8570665187248,49.8415791150679,
50.826091711411,51.810604307754,52.7951169040971,53.4070751110265),
 .UNSPECIFIED.);
#2717=B_SPLINE_CURVE_WITH_KNOTS('',3,(#32018,#32019,#32020,#32021,#32022,
#32023,#32024,#32025,#32026,#32027),.UNSPECIFIED.,.F.,.F.,(4,1,1,1,1,1,
1,4),(40.8407044966673,41.3929157131084,42.3774283094515,43.3619409057945,
44.3464535021376,45.3309660984807,46.3154786948237,47.1238898038469),
 .UNSPECIFIED.);
#2718=B_SPLINE_CURVE_WITH_KNOTS('',3,(#32028,#32029,#32030,#32031,#32032,
#32033,#32034,#32035,#32036,#32037,#32038),.UNSPECIFIED.,.F.,.F.,(4,1,1,
1,1,1,1,1,4),(40.8407044966673,40.9809657479803,41.9654783443234,42.9499909406665,
43.9345035370095,44.9190161333526,45.9035287296957,46.8880413260387,47.1238898038469),
 .UNSPECIFIED.);
#2719=B_SPLINE_CURVE_WITH_KNOTS('',3,(#32043,#32044,#32045,#32046,#32047,
#32048,#32049,#32050,#32051,#32052),.UNSPECIFIED.,.F.,.F.,(4,1,1,1,1,1,
1,4),(34.5575191894877,35.48584013505,36.4703527313931,37.4548653277361,
38.4393779240792,39.4238905204223,40.4084031167653,40.8407044966673),
 .UNSPECIFIED.);
#2720=B_SPLINE_CURVE_WITH_KNOTS('',3,(#32053,#32054,#32055,#32056,#32057,
#32058,#32059,#32060,#32061,#32062),.UNSPECIFIED.,.F.,.F.,(4,1,1,1,1,1,
1,4),(34.5575191894877,35.0738901699219,36.058402766265,37.0429153626081,
38.0274279589511,39.0119405552942,39.9964531516373,40.8407044966673),
 .UNSPECIFIED.);
#2721=B_SPLINE_CURVE_WITH_KNOTS('',3,(#32067,#32068,#32069,#32070,#32071,
#32072,#32073,#32074,#32075,#32076,#32077),.UNSPECIFIED.,.F.,.F.,(4,1,1,
1,1,1,1,1,4),(28.2743338823081,28.5942519606485,29.5787645569916,30.5632771533347,
31.5477897496777,32.5323023460208,33.5168149423639,34.5013275387069,34.5575191894877),
 .UNSPECIFIED.);
#2722=B_SPLINE_CURVE_WITH_KNOTS('',3,(#32078,#32079,#32080,#32081,#32082,
#32083,#32084,#32085,#32086,#32087),.UNSPECIFIED.,.F.,.F.,(4,1,1,1,1,1,
1,4),(28.2743338823081,29.1668145918635,30.1513271882066,31.1358397845497,
32.1203523808927,33.1048649772358,34.0893775735789,34.5575191894877),
 .UNSPECIFIED.);
#2723=B_SPLINE_CURVE_WITH_KNOTS('',3,(#32092,#32093,#32094,#32095,#32096,
#32097,#32098,#32099,#32100,#32101),.UNSPECIFIED.,.F.,.F.,(4,1,1,1,1,1,
1,4),(21.9911485751285,22.6871763825901,23.6716889789332,24.6562015752763,
25.6407141716193,26.6252267679624,27.6097393643055,28.2743338823081),
 .UNSPECIFIED.);
#2724=B_SPLINE_CURVE_WITH_KNOTS('',3,(#32102,#32103,#32104,#32105,#32106,
#32107,#32108,#32109,#32110,#32111,#32112),.UNSPECIFIED.,.F.,.F.,(4,1,1,
1,1,1,1,1,4),(21.9911485751285,22.2752264174621,23.2597390138051,24.2442516101482,
25.2287642064913,26.2132768028343,27.1977893991774,28.1823019955205,28.2743338823081),
 .UNSPECIFIED.);
#2725=B_SPLINE_CURVE_WITH_KNOTS('',3,(#32118,#32119,#32120,#32121,#32122),
 .UNSPECIFIED.,.F.,.F.,(4,1,4),(14.3991256467175,15.3836382430606,15.7079632679489),
 .UNSPECIFIED.);
#2726=B_SPLINE_CURVE_WITH_KNOTS('',3,(#32125,#32126,#32127,#32128,#32129),
 .UNSPECIFIED.,.F.,.F.,(4,1,4),(13.8752082355906,14.8110756118456,15.7079632679489),
 .UNSPECIFIED.);
#2727=B_SPLINE_CURVE_WITH_KNOTS('',3,(#32135,#32136,#32137,#32138,#32139,
#32140,#32141),.UNSPECIFIED.,.F.,.F.,(4,3,4),(45.2911347714885,46.2720920281241,
47.2566046244672),.UNSPECIFIED.);
#2728=B_SPLINE_CURVE_WITH_KNOTS('',3,(#32149,#32150,#32151,#32152,#32153,
#32154,#32155,#32156,#32157,#32158,#32159,#32160,#32161),.UNSPECIFIED.,
 .F.,.F.,(4,3,3,3,4),(-45.238934211693,-44.303066835438,-43.3185542390949,
-42.3340416427519,-41.54953728821),.UNSPECIFIED.);
#2729=B_SPLINE_CURVE_WITH_KNOTS('',3,(#32166,#32167,#32168,#32169,#32170,
#32171,#32172,#32173,#32174,#32175,#32176,#32177,#32178,#32179,#32180,#32181,
#32182,#32183,#32184,#32185,#32186,#32187,#32188,#32189,#32190),
 .UNSPECIFIED.,.F.,.F.,(4,3,3,3,3,3,3,3,4),(39.0079494643089,39.3805038537226,
40.3650164500657,41.3495290464088,42.3340416427518,43.3185542390949,44.303066835438,
45.287579431781,45.2911347714885),.UNSPECIFIED.);
#2730=B_SPLINE_CURVE_WITH_KNOTS('',3,(#32191,#32192,#32193,#32194,#32195,
#32196,#32197,#32198,#32199,#32200,#32201,#32202,#32203,#32204,#32205,#32206,
#32207,#32208,#32209,#32210,#32211,#32212,#32213,#32214,#32215),
 .UNSPECIFIED.,.F.,.F.,(4,3,3,3,3,3,3,3,4),(-41.54953728821,-41.3495290464088,
-40.3650164500657,-39.3805038537227,-38.3959912573796,-37.4114786610365,
-36.4269660646935,-35.4424534683504,-35.2663519810305),.UNSPECIFIED.);
#2731=B_SPLINE_CURVE_WITH_KNOTS('',3,(#32220,#32221,#32222,#32223,#32224,
#32225,#32226,#32227,#32228,#32229,#32230,#32231,#32232,#32233,#32234,#32235,
#32236,#32237,#32238,#32239,#32240,#32241),.UNSPECIFIED.,.F.,.F.,(4,3,3,
3,3,3,3,4),(32.7247641571293,33.4734282756642,34.4579408720073,35.4424534683504,
36.4269660646934,37.4114786610365,38.3959912573796,39.0079494643089),
 .UNSPECIFIED.);
#2732=B_SPLINE_CURVE_WITH_KNOTS('',3,(#32242,#32243,#32244,#32245,#32246,
#32247,#32248,#32249,#32250,#32251,#32252,#32253,#32254,#32255,#32256,#32257,
#32258,#32259,#32260,#32261,#32262,#32263),.UNSPECIFIED.,.F.,.F.,(4,3,3,
3,3,3,3,4),(-35.2663519810305,-34.4579408720073,-33.4734282756642,-32.4889156793212,
-31.5044030829781,-30.5198904866351,-29.535377890292,-28.9831666738509),
 .UNSPECIFIED.);
#2733=B_SPLINE_CURVE_WITH_KNOTS('',3,(#32268,#32269,#32270,#32271,#32272,
#32273,#32274,#32275,#32276,#32277,#32278,#32279,#32280,#32281,#32282,#32283,
#32284,#32285,#32286,#32287,#32288,#32289,#32290,#32291,#32292),
 .UNSPECIFIED.,.F.,.F.,(4,3,3,3,3,3,3,3,4),(26.4415788499498,26.5818401012628,
27.5663526976058,28.5508652939489,29.535377890292,30.519890486635,31.5044030829781,
32.4889156793212,32.7247641571293),.UNSPECIFIED.);
#2734=B_SPLINE_CURVE_WITH_KNOTS('',3,(#32293,#32294,#32295,#32296,#32297,
#32298,#32299,#32300,#32301,#32302,#32303,#32304,#32305,#32306,#32307,#32308,
#32309,#32310,#32311,#32312,#32313,#32314),.UNSPECIFIED.,.F.,.F.,(4,3,3,
3,3,3,3,4),(-28.9831666738509,-28.5508652939489,-27.5663526976059,-26.5818401012628,
-25.5973275049197,-24.6128149085767,-23.6283023122336,-22.6999813666713),
 .UNSPECIFIED.);
#2735=B_SPLINE_CURVE_WITH_KNOTS('',3,(#32319,#32320,#32321,#32322,#32323,
#32324,#32325,#32326,#32327,#32328,#32329,#32330,#32331,#32332,#32333,#32334,
#32335,#32336,#32337,#32338,#32339,#32340),.UNSPECIFIED.,.F.,.F.,(4,3,3,
3,3,3,3,4),(20.1583935427702,20.6747645232044,21.6592771195474,22.6437897158905,
23.6283023122336,24.6128149085766,25.5973275049197,26.4415788499498),
 .UNSPECIFIED.);
#2736=B_SPLINE_CURVE_WITH_KNOTS('',3,(#32341,#32342,#32343,#32344,#32345,
#32346,#32347,#32348,#32349,#32350,#32351,#32352,#32353,#32354,#32355,#32356,
#32357,#32358,#32359,#32360,#32361,#32362,#32363,#32364,#32365),
 .UNSPECIFIED.,.F.,.F.,(4,3,3,3,3,3,3,3,4),(-22.6999813666713,-22.6437897158905,
-21.6592771195475,-20.6747645232044,-19.6902519268613,-18.7057393305183,
-17.7212267341752,-16.7367141378321,-16.4167960594917),.UNSPECIFIED.);
#2737=B_SPLINE_CURVE_WITH_KNOTS('',3,(#32370,#32371,#32372,#32373,#32374,
#32375,#32376,#32377,#32378,#32379,#32380,#32381,#32382,#32383,#32384,#32385,
#32386,#32387,#32388,#32389,#32390,#32391),.UNSPECIFIED.,.F.,.F.,(4,3,3,
3,3,3,3,4),(13.8752082355906,14.767688945146,15.7522015414891,16.7367141378321,
17.7212267341752,18.7057393305182,19.6902519268613,20.1583935427702),
 .UNSPECIFIED.);
#2738=B_SPLINE_CURVE_WITH_KNOTS('',3,(#32392,#32393,#32394,#32395,#32396,
#32397,#32398,#32399,#32400,#32401,#32402,#32403,#32404,#32405,#32406,#32407,
#32408,#32409,#32410,#32411,#32412,#32413),.UNSPECIFIED.,.F.,.F.,(4,3,3,
3,3,3,3,4),(-16.4167960594917,-15.7522015414891,-14.767688945146,-13.7831763488029,
-12.7986637524599,-11.8141511561168,-10.8296385597737,-10.1336107523121),
 .UNSPECIFIED.);
#2739=B_SPLINE_CURVE_WITH_KNOTS('',3,(#32419,#32420,#32421,#32422,#32423,
#32424,#32425,#32426,#32427,#32428,#32429,#32430,#32431),.UNSPECIFIED.,
 .F.,.F.,(4,3,3,3,4),(-3.85042544513253,-2.9535377890292,-1.96902519268613,
-0.984512596343066,0.),.UNSPECIFIED.);
#2740=B_SPLINE_CURVE_WITH_KNOTS('',3,(#32434,#32435,#32436,#32437,#32438,
#32439,#32440,#32441,#32442,#32443,#32444,#32445,#32446,#32447,#32448,#32449,
#32450,#32451,#32452),.UNSPECIFIED.,.F.,.F.,(4,3,3,3,3,3,4),(2.01767041277416,
2.9535377890292,3.93805038537227,4.92256298171533,5.9070755780584,6.89158817440146,
7.592022928411),.UNSPECIFIED.);
#2741=B_SPLINE_CURVE_WITH_KNOTS('',3,(#32458,#32459,#32460,#32461,#32462,
#32463,#32464,#32465,#32466),.UNSPECIFIED.,.F.,.F.,(4,1,1,1,1,1,4),(53.4070751110265,
54.1915794655683,55.1760920619113,56.1606046582544,57.1451172545975,58.1296298509405,
59.1141424472836),.UNSPECIFIED.);
#2742=B_SPLINE_CURVE_WITH_KNOTS('',3,(#32469,#32470,#32471,#32472,#32473,
#32474,#32475,#32476,#32477,#32478),.UNSPECIFIED.,.F.,.F.,(4,1,1,1,1,1,
1,4),(53.4070751110265,53.7796295004402,54.7641420967832,55.7486546931263,
56.7331672894694,57.7176798858124,58.7021924821555,59.6380598584105),
 .UNSPECIFIED.);
#2743=B_SPLINE_CURVE_WITH_KNOTS('',3,(#32483,#32484,#32485,#32486,#32487,
#32488,#32489,#32490,#32491,#32492,#32493),.UNSPECIFIED.,.F.,.F.,(4,1,1,
1,1,1,1,1,4),(47.1238898038469,47.2999912911668,48.2845038875099,49.2690164838529,
50.253529080196,51.2380416765391,52.2225542728821,53.2070668692252,53.4070751110265),
 .UNSPECIFIED.);
#2744=B_SPLINE_CURVE_WITH_KNOTS('',3,(#32494,#32495,#32496,#32497,#32498,
#32499,#32500,#32501,#32502,#32503),.UNSPECIFIED.,.F.,.F.,(4,1,1,1,1,1,
1,4),(47.1238898038469,47.8725539223818,48.8570665187248,49.8415791150679,
50.826091711411,51.810604307754,52.7951169040971,53.4070751110265),
 .UNSPECIFIED.);
#2745=B_SPLINE_CURVE_WITH_KNOTS('',3,(#32508,#32509,#32510,#32511,#32512,
#32513,#32514,#32515,#32516,#32517),.UNSPECIFIED.,.F.,.F.,(4,1,1,1,1,1,
1,4),(40.8407044966673,41.3929157131084,42.3774283094515,43.3619409057945,
44.3464535021376,45.3309660984807,46.3154786948237,47.1238898038469),
 .UNSPECIFIED.);
#2746=B_SPLINE_CURVE_WITH_KNOTS('',3,(#32518,#32519,#32520,#32521,#32522,
#32523,#32524,#32525,#32526,#32527,#32528),.UNSPECIFIED.,.F.,.F.,(4,1,1,
1,1,1,1,1,4),(40.8407044966673,40.9809657479803,41.9654783443234,42.9499909406664,
43.9345035370095,44.9190161333526,45.9035287296956,46.8880413260387,47.1238898038469),
 .UNSPECIFIED.);
#2747=B_SPLINE_CURVE_WITH_KNOTS('',3,(#32533,#32534,#32535,#32536,#32537,
#32538,#32539,#32540,#32541,#32542),.UNSPECIFIED.,.F.,.F.,(4,1,1,1,1,1,
1,4),(34.5575191894877,35.48584013505,36.4703527313931,37.4548653277361,
38.4393779240792,39.4238905204223,40.4084031167653,40.8407044966673),
 .UNSPECIFIED.);
#2748=B_SPLINE_CURVE_WITH_KNOTS('',3,(#32543,#32544,#32545,#32546,#32547,
#32548,#32549,#32550,#32551,#32552),.UNSPECIFIED.,.F.,.F.,(4,1,1,1,1,1,
1,4),(34.5575191894877,35.0738901699219,36.058402766265,37.042915362608,
38.0274279589511,39.0119405552942,39.9964531516372,40.8407044966673),
 .UNSPECIFIED.);
#2749=B_SPLINE_CURVE_WITH_KNOTS('',3,(#32557,#32558,#32559,#32560,#32561,
#32562,#32563,#32564,#32565,#32566,#32567),.UNSPECIFIED.,.F.,.F.,(4,1,1,
1,1,1,1,1,4),(28.2743338823081,28.5942519606485,29.5787645569916,30.5632771533347,
31.5477897496777,32.5323023460208,33.5168149423639,34.5013275387069,34.5575191894877),
 .UNSPECIFIED.);
#2750=B_SPLINE_CURVE_WITH_KNOTS('',3,(#32568,#32569,#32570,#32571,#32572,
#32573,#32574,#32575,#32576,#32577),.UNSPECIFIED.,.F.,.F.,(4,1,1,1,1,1,
1,4),(28.2743338823081,29.1668145918635,30.1513271882066,31.1358397845496,
32.1203523808927,33.1048649772358,34.0893775735788,34.5575191894877),
 .UNSPECIFIED.);
#2751=B_SPLINE_CURVE_WITH_KNOTS('',3,(#32582,#32583,#32584,#32585,#32586,
#32587,#32588,#32589,#32590,#32591),.UNSPECIFIED.,.F.,.F.,(4,1,1,1,1,1,
1,4),(21.9911485751285,22.6871763825901,23.6716889789332,24.6562015752763,
25.6407141716193,26.6252267679624,27.6097393643055,28.2743338823081),
 .UNSPECIFIED.);
#2752=B_SPLINE_CURVE_WITH_KNOTS('',3,(#32592,#32593,#32594,#32595,#32596,
#32597,#32598,#32599,#32600,#32601,#32602),.UNSPECIFIED.,.F.,.F.,(4,1,1,
1,1,1,1,1,4),(21.9911485751285,22.2752264174621,23.2597390138051,24.2442516101482,
25.2287642064913,26.2132768028343,27.1977893991774,28.1823019955205,28.2743338823081),
 .UNSPECIFIED.);
#2753=B_SPLINE_CURVE_WITH_KNOTS('',3,(#32608,#32609,#32610,#32611,#32612),
 .UNSPECIFIED.,.F.,.F.,(4,1,4),(14.3991256467175,15.3836382430606,15.7079632679489),
 .UNSPECIFIED.);
#2754=B_SPLINE_CURVE_WITH_KNOTS('',3,(#32615,#32616,#32617,#32618,#32619),
 .UNSPECIFIED.,.F.,.F.,(4,1,4),(13.8752082355906,14.8110756118456,15.7079632679489),
 .UNSPECIFIED.);
#2755=B_SPLINE_CURVE_WITH_KNOTS('',3,(#32625,#32626,#32627,#32628,#32629,
#32630,#32631),.UNSPECIFIED.,.F.,.F.,(4,3,4),(45.2911347714885,46.2720920281241,
47.2566046244672),.UNSPECIFIED.);
#2756=B_SPLINE_CURVE_WITH_KNOTS('',3,(#32639,#32640,#32641,#32642,#32643,
#32644,#32645,#32646,#32647,#32648,#32649,#32650,#32651),.UNSPECIFIED.,
 .F.,.F.,(4,3,3,3,4),(-45.238934211693,-44.303066835438,-43.3185542390949,
-42.3340416427518,-41.5495372882101),.UNSPECIFIED.);
#2757=B_SPLINE_CURVE_WITH_KNOTS('',3,(#32656,#32657,#32658,#32659,#32660,
#32661,#32662,#32663,#32664,#32665,#32666,#32667,#32668,#32669,#32670,#32671,
#32672,#32673,#32674,#32675,#32676,#32677,#32678,#32679,#32680),
 .UNSPECIFIED.,.F.,.F.,(4,3,3,3,3,3,3,3,4),(39.0079494643089,39.3805038537227,
40.3650164500657,41.3495290464088,42.3340416427518,43.3185542390949,44.303066835438,
45.287579431781,45.2911347714885),.UNSPECIFIED.);
#2758=B_SPLINE_CURVE_WITH_KNOTS('',3,(#32681,#32682,#32683,#32684,#32685,
#32686,#32687,#32688,#32689,#32690,#32691,#32692,#32693,#32694,#32695,#32696,
#32697,#32698,#32699,#32700,#32701,#32702,#32703,#32704,#32705),
 .UNSPECIFIED.,.F.,.F.,(4,3,3,3,3,3,3,3,4),(-41.5495372882101,-41.3495290464088,
-40.3650164500657,-39.3805038537227,-38.3959912573796,-37.4114786610365,
-36.4269660646935,-35.4424534683504,-35.2663519810305),.UNSPECIFIED.);
#2759=B_SPLINE_CURVE_WITH_KNOTS('',3,(#32710,#32711,#32712,#32713,#32714,
#32715,#32716,#32717,#32718,#32719,#32720,#32721,#32722,#32723,#32724,#32725,
#32726,#32727,#32728,#32729,#32730,#32731),.UNSPECIFIED.,.F.,.F.,(4,3,3,
3,3,3,3,4),(32.7247641571293,33.4734282756643,34.4579408720073,35.4424534683504,
36.4269660646935,37.4114786610365,38.3959912573796,39.0079494643089),
 .UNSPECIFIED.);
#2760=B_SPLINE_CURVE_WITH_KNOTS('',3,(#32732,#32733,#32734,#32735,#32736,
#32737,#32738,#32739,#32740,#32741,#32742,#32743,#32744,#32745,#32746,#32747,
#32748,#32749,#32750,#32751,#32752,#32753),.UNSPECIFIED.,.F.,.F.,(4,3,3,
3,3,3,3,4),(-35.2663519810305,-34.4579408720073,-33.4734282756643,-32.4889156793212,
-31.5044030829781,-30.5198904866351,-29.535377890292,-28.9831666738509),
 .UNSPECIFIED.);
#2761=B_SPLINE_CURVE_WITH_KNOTS('',3,(#32758,#32759,#32760,#32761,#32762,
#32763,#32764,#32765,#32766,#32767,#32768,#32769,#32770,#32771,#32772,#32773,
#32774,#32775,#32776,#32777,#32778,#32779,#32780,#32781,#32782),
 .UNSPECIFIED.,.F.,.F.,(4,3,3,3,3,3,3,3,4),(26.4415788499498,26.5818401012628,
27.5663526976059,28.5508652939489,29.535377890292,30.5198904866351,31.5044030829781,
32.4889156793212,32.7247641571293),.UNSPECIFIED.);
#2762=B_SPLINE_CURVE_WITH_KNOTS('',3,(#32783,#32784,#32785,#32786,#32787,
#32788,#32789,#32790,#32791,#32792,#32793,#32794,#32795,#32796,#32797,#32798,
#32799,#32800,#32801,#32802,#32803,#32804),.UNSPECIFIED.,.F.,.F.,(4,3,3,
3,3,3,3,4),(-28.9831666738509,-28.5508652939489,-27.5663526976059,-26.5818401012628,
-25.5973275049197,-24.6128149085767,-23.6283023122336,-22.6999813666713),
 .UNSPECIFIED.);
#2763=B_SPLINE_CURVE_WITH_KNOTS('',3,(#32809,#32810,#32811,#32812,#32813,
#32814,#32815,#32816,#32817,#32818,#32819,#32820,#32821,#32822,#32823,#32824,
#32825,#32826,#32827,#32828,#32829,#32830),.UNSPECIFIED.,.F.,.F.,(4,3,3,
3,3,3,3,4),(20.1583935427702,20.6747645232044,21.6592771195475,22.6437897158905,
23.6283023122336,24.6128149085767,25.5973275049197,26.4415788499498),
 .UNSPECIFIED.);
#2764=B_SPLINE_CURVE_WITH_KNOTS('',3,(#32831,#32832,#32833,#32834,#32835,
#32836,#32837,#32838,#32839,#32840,#32841,#32842,#32843,#32844,#32845,#32846,
#32847,#32848,#32849,#32850,#32851,#32852,#32853,#32854,#32855),
 .UNSPECIFIED.,.F.,.F.,(4,3,3,3,3,3,3,3,4),(-22.6999813666713,-22.6437897158905,
-21.6592771195475,-20.6747645232044,-19.6902519268613,-18.7057393305183,
-17.7212267341752,-16.7367141378321,-16.4167960594917),.UNSPECIFIED.);
#2765=B_SPLINE_CURVE_WITH_KNOTS('',3,(#32860,#32861,#32862,#32863,#32864,
#32865,#32866,#32867,#32868,#32869,#32870,#32871,#32872,#32873,#32874,#32875,
#32876,#32877,#32878,#32879,#32880,#32881),.UNSPECIFIED.,.F.,.F.,(4,3,3,
3,3,3,3,4),(13.8752082355906,14.767688945146,15.7522015414891,16.7367141378321,
17.7212267341752,18.7057393305183,19.6902519268613,20.1583935427702),
 .UNSPECIFIED.);
#2766=B_SPLINE_CURVE_WITH_KNOTS('',3,(#32882,#32883,#32884,#32885,#32886,
#32887,#32888,#32889,#32890,#32891,#32892,#32893,#32894,#32895,#32896,#32897,
#32898,#32899,#32900,#32901,#32902,#32903),.UNSPECIFIED.,.F.,.F.,(4,3,3,
3,3,3,3,4),(-16.4167960594917,-15.7522015414891,-14.767688945146,-13.7831763488029,
-12.7986637524599,-11.8141511561168,-10.8296385597737,-10.1336107523121),
 .UNSPECIFIED.);
#2767=B_SPLINE_CURVE_WITH_KNOTS('',3,(#32909,#32910,#32911,#32912,#32913,
#32914,#32915,#32916,#32917,#32918,#32919,#32920,#32921),.UNSPECIFIED.,
 .F.,.F.,(4,3,3,3,4),(-3.85042544513253,-2.9535377890292,-1.96902519268613,
-0.984512596343067,0.),.UNSPECIFIED.);
#2768=B_SPLINE_CURVE_WITH_KNOTS('',3,(#32924,#32925,#32926,#32927,#32928,
#32929,#32930,#32931,#32932,#32933,#32934,#32935,#32936,#32937,#32938,#32939,
#32940,#32941,#32942),.UNSPECIFIED.,.F.,.F.,(4,3,3,3,3,3,4),(2.01767041277416,
2.9535377890292,3.93805038537227,4.92256298171533,5.9070755780584,6.89158817440147,
7.592022928411),.UNSPECIFIED.);
#2769=B_SPLINE_CURVE_WITH_KNOTS('',3,(#32948,#32949,#32950,#32951,#32952,
#32953,#32954,#32955,#32956),.UNSPECIFIED.,.F.,.F.,(4,1,1,1,1,1,4),(53.4070751110265,
54.1915794655683,55.1760920619113,56.1606046582544,57.1451172545975,58.1296298509405,
59.1141424472836),.UNSPECIFIED.);
#2770=B_SPLINE_CURVE_WITH_KNOTS('',3,(#32959,#32960,#32961,#32962,#32963,
#32964,#32965,#32966,#32967,#32968),.UNSPECIFIED.,.F.,.F.,(4,1,1,1,1,1,
1,4),(53.4070751110265,53.7796295004402,54.7641420967832,55.7486546931263,
56.7331672894694,57.7176798858124,58.7021924821555,59.6380598584106),
 .UNSPECIFIED.);
#2771=B_SPLINE_CURVE_WITH_KNOTS('',3,(#32973,#32974,#32975,#32976,#32977,
#32978,#32979,#32980,#32981,#32982,#32983),.UNSPECIFIED.,.F.,.F.,(4,1,1,
1,1,1,1,1,4),(47.1238898038469,47.2999912911668,48.2845038875099,49.2690164838529,
50.253529080196,51.2380416765391,52.2225542728821,53.2070668692252,53.4070751110265),
 .UNSPECIFIED.);
#2772=B_SPLINE_CURVE_WITH_KNOTS('',3,(#32984,#32985,#32986,#32987,#32988,
#32989,#32990,#32991,#32992,#32993),.UNSPECIFIED.,.F.,.F.,(4,1,1,1,1,1,
1,4),(47.1238898038469,47.8725539223818,48.8570665187248,49.8415791150679,
50.826091711411,51.810604307754,52.7951169040971,53.4070751110265),
 .UNSPECIFIED.);
#2773=B_SPLINE_CURVE_WITH_KNOTS('',3,(#32998,#32999,#33000,#33001,#33002,
#33003,#33004,#33005,#33006,#33007),.UNSPECIFIED.,.F.,.F.,(4,1,1,1,1,1,
1,4),(40.8407044966673,41.3929157131084,42.3774283094515,43.3619409057945,
44.3464535021376,45.3309660984807,46.3154786948237,47.1238898038469),
 .UNSPECIFIED.);
#2774=B_SPLINE_CURVE_WITH_KNOTS('',3,(#33008,#33009,#33010,#33011,#33012,
#33013,#33014,#33015,#33016,#33017,#33018),.UNSPECIFIED.,.F.,.F.,(4,1,1,
1,1,1,1,1,4),(40.8407044966673,40.9809657479803,41.9654783443234,42.9499909406665,
43.9345035370095,44.9190161333526,45.9035287296957,46.8880413260387,47.1238898038469),
 .UNSPECIFIED.);
#2775=B_SPLINE_CURVE_WITH_KNOTS('',3,(#33023,#33024,#33025,#33026,#33027,
#33028,#33029,#33030,#33031,#33032),.UNSPECIFIED.,.F.,.F.,(4,1,1,1,1,1,
1,4),(34.5575191894877,35.48584013505,36.4703527313931,37.4548653277361,
38.4393779240792,39.4238905204223,40.4084031167653,40.8407044966673),
 .UNSPECIFIED.);
#2776=B_SPLINE_CURVE_WITH_KNOTS('',3,(#33033,#33034,#33035,#33036,#33037,
#33038,#33039,#33040,#33041,#33042),.UNSPECIFIED.,.F.,.F.,(4,1,1,1,1,1,
1,4),(34.5575191894877,35.0738901699219,36.058402766265,37.0429153626081,
38.0274279589511,39.0119405552942,39.9964531516373,40.8407044966673),
 .UNSPECIFIED.);
#2777=B_SPLINE_CURVE_WITH_KNOTS('',3,(#33047,#33048,#33049,#33050,#33051,
#33052,#33053,#33054,#33055,#33056,#33057),.UNSPECIFIED.,.F.,.F.,(4,1,1,
1,1,1,1,1,4),(28.2743338823081,28.5942519606485,29.5787645569916,30.5632771533347,
31.5477897496777,32.5323023460208,33.5168149423639,34.5013275387069,34.5575191894877),
 .UNSPECIFIED.);
#2778=B_SPLINE_CURVE_WITH_KNOTS('',3,(#33058,#33059,#33060,#33061,#33062,
#33063,#33064,#33065,#33066,#33067),.UNSPECIFIED.,.F.,.F.,(4,1,1,1,1,1,
1,4),(28.2743338823081,29.1668145918635,30.1513271882066,31.1358397845497,
32.1203523808927,33.1048649772358,34.0893775735789,34.5575191894877),
 .UNSPECIFIED.);
#2779=B_SPLINE_CURVE_WITH_KNOTS('',3,(#33072,#33073,#33074,#33075,#33076,
#33077,#33078,#33079,#33080,#33081),.UNSPECIFIED.,.F.,.F.,(4,1,1,1,1,1,
1,4),(21.9911485751285,22.6871763825901,23.6716889789332,24.6562015752763,
25.6407141716193,26.6252267679624,27.6097393643055,28.2743338823081),
 .UNSPECIFIED.);
#2780=B_SPLINE_CURVE_WITH_KNOTS('',3,(#33082,#33083,#33084,#33085,#33086,
#33087,#33088,#33089,#33090,#33091,#33092),.UNSPECIFIED.,.F.,.F.,(4,1,1,
1,1,1,1,1,4),(21.9911485751285,22.2752264174621,23.2597390138051,24.2442516101482,
25.2287642064913,26.2132768028343,27.1977893991774,28.1823019955205,28.2743338823081),
 .UNSPECIFIED.);
#2781=B_SPLINE_CURVE_WITH_KNOTS('',3,(#33098,#33099,#33100,#33101,#33102),
 .UNSPECIFIED.,.F.,.F.,(4,1,4),(14.3991256467175,15.3836382430606,15.7079632679489),
 .UNSPECIFIED.);
#2782=B_SPLINE_CURVE_WITH_KNOTS('',3,(#33105,#33106,#33107,#33108,#33109),
 .UNSPECIFIED.,.F.,.F.,(4,1,4),(13.8752082355906,14.8110756118456,15.7079632679489),
 .UNSPECIFIED.);
#2783=B_SPLINE_CURVE_WITH_KNOTS('',3,(#33115,#33116,#33117,#33118,#33119,
#33120,#33121),.UNSPECIFIED.,.F.,.F.,(4,3,4),(45.2911347714885,46.2720920281241,
47.2566046244672),.UNSPECIFIED.);
#2784=B_SPLINE_CURVE_WITH_KNOTS('',3,(#33129,#33130,#33131,#33132,#33133,
#33134,#33135,#33136,#33137,#33138,#33139,#33140,#33141),.UNSPECIFIED.,
 .F.,.F.,(4,3,3,3,4),(-45.238934211693,-44.303066835438,-43.3185542390949,
-42.3340416427518,-41.54953728821),.UNSPECIFIED.);
#2785=B_SPLINE_CURVE_WITH_KNOTS('',3,(#33146,#33147,#33148,#33149,#33150,
#33151,#33152,#33153,#33154,#33155,#33156,#33157,#33158,#33159,#33160,#33161,
#33162,#33163,#33164,#33165,#33166,#33167,#33168,#33169,#33170),
 .UNSPECIFIED.,.F.,.F.,(4,3,3,3,3,3,3,3,4),(39.0079494643089,39.3805038537226,
40.3650164500657,41.3495290464088,42.3340416427518,43.3185542390949,44.303066835438,
45.287579431781,45.2911347714885),.UNSPECIFIED.);
#2786=B_SPLINE_CURVE_WITH_KNOTS('',3,(#33171,#33172,#33173,#33174,#33175,
#33176,#33177,#33178,#33179,#33180,#33181,#33182,#33183,#33184,#33185,#33186,
#33187,#33188,#33189,#33190,#33191,#33192,#33193,#33194,#33195),
 .UNSPECIFIED.,.F.,.F.,(4,3,3,3,3,3,3,3,4),(-41.54953728821,-41.3495290464088,
-40.3650164500657,-39.3805038537226,-38.3959912573796,-37.4114786610365,
-36.4269660646934,-35.4424534683504,-35.2663519810305),.UNSPECIFIED.);
#2787=B_SPLINE_CURVE_WITH_KNOTS('',3,(#33200,#33201,#33202,#33203,#33204,
#33205,#33206,#33207,#33208,#33209,#33210,#33211,#33212,#33213,#33214,#33215,
#33216,#33217,#33218,#33219,#33220,#33221),.UNSPECIFIED.,.F.,.F.,(4,3,3,
3,3,3,3,4),(32.7247641571293,33.4734282756642,34.4579408720073,35.4424534683504,
36.4269660646934,37.4114786610365,38.3959912573796,39.0079494643089),
 .UNSPECIFIED.);
#2788=B_SPLINE_CURVE_WITH_KNOTS('',3,(#33222,#33223,#33224,#33225,#33226,
#33227,#33228,#33229,#33230,#33231,#33232,#33233,#33234,#33235,#33236,#33237,
#33238,#33239,#33240,#33241,#33242,#33243),.UNSPECIFIED.,.F.,.F.,(4,3,3,
3,3,3,3,4),(-35.2663519810305,-34.4579408720073,-33.4734282756642,-32.4889156793212,
-31.5044030829781,-30.519890486635,-29.535377890292,-28.9831666738509),
 .UNSPECIFIED.);
#2789=B_SPLINE_CURVE_WITH_KNOTS('',3,(#33248,#33249,#33250,#33251,#33252,
#33253,#33254,#33255,#33256,#33257,#33258,#33259,#33260,#33261,#33262,#33263,
#33264,#33265,#33266,#33267,#33268,#33269,#33270,#33271,#33272),
 .UNSPECIFIED.,.F.,.F.,(4,3,3,3,3,3,3,3,4),(26.4415788499497,26.5818401012628,
27.5663526976059,28.5508652939489,29.535377890292,30.519890486635,31.5044030829781,
32.4889156793212,32.7247641571293),.UNSPECIFIED.);
#2790=B_SPLINE_CURVE_WITH_KNOTS('',3,(#33273,#33274,#33275,#33276,#33277,
#33278,#33279,#33280,#33281,#33282,#33283,#33284,#33285,#33286,#33287,#33288,
#33289,#33290,#33291,#33292,#33293,#33294),.UNSPECIFIED.,.F.,.F.,(4,3,3,
3,3,3,3,4),(-28.9831666738509,-28.5508652939489,-27.5663526976059,-26.5818401012628,
-25.5973275049197,-24.6128149085767,-23.6283023122336,-22.6999813666713),
 .UNSPECIFIED.);
#2791=B_SPLINE_CURVE_WITH_KNOTS('',3,(#33299,#33300,#33301,#33302,#33303,
#33304,#33305,#33306,#33307,#33308,#33309,#33310,#33311,#33312,#33313,#33314,
#33315,#33316,#33317,#33318,#33319,#33320),.UNSPECIFIED.,.F.,.F.,(4,3,3,
3,3,3,3,4),(20.1583935427702,20.6747645232044,21.6592771195474,22.6437897158905,
23.6283023122336,24.6128149085766,25.5973275049197,26.4415788499497),
 .UNSPECIFIED.);
#2792=B_SPLINE_CURVE_WITH_KNOTS('',3,(#33321,#33322,#33323,#33324,#33325,
#33326,#33327,#33328,#33329,#33330,#33331,#33332,#33333,#33334,#33335,#33336,
#33337,#33338,#33339,#33340,#33341,#33342,#33343,#33344,#33345),
 .UNSPECIFIED.,.F.,.F.,(4,3,3,3,3,3,3,3,4),(-22.6999813666713,-22.6437897158905,
-21.6592771195475,-20.6747645232044,-19.6902519268613,-18.7057393305183,
-17.7212267341752,-16.7367141378321,-16.4167960594917),.UNSPECIFIED.);
#2793=B_SPLINE_CURVE_WITH_KNOTS('',3,(#33350,#33351,#33352,#33353,#33354,
#33355,#33356,#33357,#33358,#33359,#33360,#33361,#33362,#33363,#33364,#33365,
#33366,#33367,#33368,#33369,#33370,#33371),.UNSPECIFIED.,.F.,.F.,(4,3,3,
3,3,3,3,4),(13.8752082355906,14.767688945146,15.7522015414891,16.7367141378321,
17.7212267341752,18.7057393305182,19.6902519268613,20.1583935427702),
 .UNSPECIFIED.);
#2794=B_SPLINE_CURVE_WITH_KNOTS('',3,(#33372,#33373,#33374,#33375,#33376,
#33377,#33378,#33379,#33380,#33381,#33382,#33383,#33384,#33385,#33386,#33387,
#33388,#33389,#33390,#33391,#33392,#33393),.UNSPECIFIED.,.F.,.F.,(4,3,3,
3,3,3,3,4),(-16.4167960594917,-15.7522015414891,-14.767688945146,-13.7831763488029,
-12.7986637524599,-11.8141511561168,-10.8296385597737,-10.1336107523121),
 .UNSPECIFIED.);
#2795=B_SPLINE_CURVE_WITH_KNOTS('',3,(#33399,#33400,#33401,#33402,#33403,
#33404,#33405,#33406,#33407,#33408,#33409,#33410,#33411),.UNSPECIFIED.,
 .F.,.F.,(4,3,3,3,4),(-3.85042544513252,-2.9535377890292,-1.96902519268613,
-0.984512596343066,0.),.UNSPECIFIED.);
#2796=B_SPLINE_CURVE_WITH_KNOTS('',3,(#33414,#33415,#33416,#33417,#33418,
#33419,#33420,#33421,#33422,#33423,#33424,#33425,#33426,#33427,#33428,#33429,
#33430,#33431,#33432),.UNSPECIFIED.,.F.,.F.,(4,3,3,3,3,3,4),(2.01767041277416,
2.9535377890292,3.93805038537226,4.92256298171533,5.90707557805839,6.89158817440146,
7.59202292841098),.UNSPECIFIED.);
#2797=B_SPLINE_CURVE_WITH_KNOTS('',3,(#33438,#33439,#33440,#33441,#33442,
#33443,#33444,#33445,#33446),.UNSPECIFIED.,.F.,.F.,(4,1,1,1,1,1,4),(53.4070751110265,
54.1915794655683,55.1760920619113,56.1606046582544,57.1451172545975,58.1296298509405,
59.1141424472836),.UNSPECIFIED.);
#2798=B_SPLINE_CURVE_WITH_KNOTS('',3,(#33449,#33450,#33451,#33452,#33453,
#33454,#33455,#33456,#33457,#33458),.UNSPECIFIED.,.F.,.F.,(4,1,1,1,1,1,
1,4),(53.4070751110265,53.7796295004402,54.7641420967832,55.7486546931263,
56.7331672894694,57.7176798858124,58.7021924821555,59.6380598584106),
 .UNSPECIFIED.);
#2799=B_SPLINE_CURVE_WITH_KNOTS('',3,(#33463,#33464,#33465,#33466,#33467,
#33468,#33469,#33470,#33471,#33472,#33473),.UNSPECIFIED.,.F.,.F.,(4,1,1,
1,1,1,1,1,4),(47.1238898038469,47.2999912911668,48.2845038875099,49.2690164838529,
50.253529080196,51.2380416765391,52.2225542728821,53.2070668692252,53.4070751110265),
 .UNSPECIFIED.);
#2800=B_SPLINE_CURVE_WITH_KNOTS('',3,(#33474,#33475,#33476,#33477,#33478,
#33479,#33480,#33481,#33482,#33483),.UNSPECIFIED.,.F.,.F.,(4,1,1,1,1,1,
1,4),(47.1238898038469,47.8725539223818,48.8570665187248,49.8415791150679,
50.826091711411,51.810604307754,52.7951169040971,53.4070751110265),
 .UNSPECIFIED.);
#2801=B_SPLINE_CURVE_WITH_KNOTS('',3,(#33488,#33489,#33490,#33491,#33492,
#33493,#33494,#33495,#33496,#33497),.UNSPECIFIED.,.F.,.F.,(4,1,1,1,1,1,
1,4),(40.8407044966673,41.3929157131084,42.3774283094515,43.3619409057945,
44.3464535021376,45.3309660984807,46.3154786948237,47.1238898038469),
 .UNSPECIFIED.);
#2802=B_SPLINE_CURVE_WITH_KNOTS('',3,(#33498,#33499,#33500,#33501,#33502,
#33503,#33504,#33505,#33506,#33507,#33508),.UNSPECIFIED.,.F.,.F.,(4,1,1,
1,1,1,1,1,4),(40.8407044966673,40.9809657479803,41.9654783443234,42.9499909406665,
43.9345035370095,44.9190161333526,45.9035287296957,46.8880413260387,47.1238898038469),
 .UNSPECIFIED.);
#2803=B_SPLINE_CURVE_WITH_KNOTS('',3,(#33513,#33514,#33515,#33516,#33517,
#33518,#33519,#33520,#33521,#33522),.UNSPECIFIED.,.F.,.F.,(4,1,1,1,1,1,
1,4),(34.5575191894877,35.48584013505,36.4703527313931,37.4548653277361,
38.4393779240792,39.4238905204223,40.4084031167653,40.8407044966673),
 .UNSPECIFIED.);
#2804=B_SPLINE_CURVE_WITH_KNOTS('',3,(#33523,#33524,#33525,#33526,#33527,
#33528,#33529,#33530,#33531,#33532),.UNSPECIFIED.,.F.,.F.,(4,1,1,1,1,1,
1,4),(34.5575191894877,35.0738901699219,36.058402766265,37.0429153626081,
38.0274279589511,39.0119405552942,39.9964531516373,40.8407044966673),
 .UNSPECIFIED.);
#2805=B_SPLINE_CURVE_WITH_KNOTS('',3,(#33537,#33538,#33539,#33540,#33541,
#33542,#33543,#33544,#33545,#33546,#33547),.UNSPECIFIED.,.F.,.F.,(4,1,1,
1,1,1,1,1,4),(28.2743338823081,28.5942519606485,29.5787645569916,30.5632771533347,
31.5477897496777,32.5323023460208,33.5168149423639,34.5013275387069,34.5575191894877),
 .UNSPECIFIED.);
#2806=B_SPLINE_CURVE_WITH_KNOTS('',3,(#33548,#33549,#33550,#33551,#33552,
#33553,#33554,#33555,#33556,#33557),.UNSPECIFIED.,.F.,.F.,(4,1,1,1,1,1,
1,4),(28.2743338823081,29.1668145918635,30.1513271882066,31.1358397845497,
32.1203523808927,33.1048649772358,34.0893775735789,34.5575191894877),
 .UNSPECIFIED.);
#2807=B_SPLINE_CURVE_WITH_KNOTS('',3,(#33562,#33563,#33564,#33565,#33566,
#33567,#33568,#33569,#33570,#33571),.UNSPECIFIED.,.F.,.F.,(4,1,1,1,1,1,
1,4),(21.9911485751285,22.6871763825902,23.6716889789332,24.6562015752763,
25.6407141716194,26.6252267679624,27.6097393643055,28.2743338823081),
 .UNSPECIFIED.);
#2808=B_SPLINE_CURVE_WITH_KNOTS('',3,(#33572,#33573,#33574,#33575,#33576,
#33577,#33578,#33579,#33580,#33581,#33582),.UNSPECIFIED.,.F.,.F.,(4,1,1,
1,1,1,1,1,4),(21.9911485751285,22.2752264174621,23.2597390138051,24.2442516101482,
25.2287642064913,26.2132768028343,27.1977893991774,28.1823019955205,28.2743338823081),
 .UNSPECIFIED.);
#2809=B_SPLINE_CURVE_WITH_KNOTS('',3,(#33588,#33589,#33590,#33591,#33592),
 .UNSPECIFIED.,.F.,.F.,(4,1,4),(14.3991256467175,15.3836382430606,15.7079632679489),
 .UNSPECIFIED.);
#2810=B_SPLINE_CURVE_WITH_KNOTS('',3,(#33595,#33596,#33597,#33598,#33599),
 .UNSPECIFIED.,.F.,.F.,(4,1,4),(13.8752082355906,14.8110756118456,15.7079632679489),
 .UNSPECIFIED.);
#2811=B_SPLINE_CURVE_WITH_KNOTS('',3,(#33605,#33606,#33607,#33608,#33609,
#33610,#33611,#33612,#33613,#33614,#33615,#33616,#33617,#33618,#33619,#33620,
#33621,#33622,#33623,#33624,#33625,#33626,#33627,#33628,#33629,#33630,#33631,
#33632,#33633,#33634,#33635,#33636,#33637,#33638),.UNSPECIFIED.,.F.,.F.,
(4,3,3,3,3,3,3,3,3,3,3,4),(26.4410951701193,26.4459204490819,26.9356597166575,
27.4253989842331,27.9151382518087,28.4048775193843,28.8946167869599,29.3843560545355,
29.874095322111,30.3638345896866,30.8535738572622,31.3433131248378),
 .UNSPECIFIED.);
#2812=B_SPLINE_CURVE_WITH_KNOTS('',3,(#33642,#33643,#33644,#33645),
 .UNSPECIFIED.,.F.,.F.,(4,4),(-29.3215314335047,-28.9877616322403),
 .UNSPECIFIED.);
#2813=B_SPLINE_CURVE_WITH_KNOTS('',3,(#33649,#33650,#33651,#33652,#33653,
#33654,#33655,#33656,#33657,#33658,#33659,#33660,#33661,#33662,#33663,#33664,
#33665,#33666,#33667,#33668,#33669,#33670,#33671,#33672,#33673,#33674,#33675,
#33676,#33677,#33678,#33679,#33680,#33681,#33682,#33683,#33684,#33685,#33686,
#33687,#33688,#33689,#33690,#33691),.UNSPECIFIED.,.F.,.F.,(4,3,3,3,3,3,
3,3,3,3,3,3,3,3,4),(-28.9877616322403,-28.8946167869599,-28.4048775193843,
-27.9151382518087,-27.4253989842331,-26.9356597166575,-26.4459204490819,
-25.9561811815063,-25.4664419139307,-24.9767026463552,-24.4869633787796,
-23.997224111204,-23.5074848436284,-23.0177455760528,-22.7045763250607),
 .UNSPECIFIED.);
#2814=B_SPLINE_CURVE_WITH_KNOTS('',3,(#33696,#33697,#33698,#33699,#33700,
#33701,#33702,#33703,#33704,#33705,#33706,#33707,#33708,#33709,#33710,#33711,
#33712,#33713,#33714,#33715,#33716,#33717,#33718,#33719,#33720,#33721,#33722,
#33723,#33724,#33725,#33726,#33727,#33728,#33729,#33730,#33731,#33732,#33733,
#33734,#33735),.UNSPECIFIED.,.F.,.F.,(4,3,3,3,3,3,3,3,3,3,3,3,3,4),(20.1579098629397,
20.5690492381748,21.0587885057504,21.548527773326,22.0382670409016,22.5280063084772,
23.0177455760528,23.5074848436284,23.997224111204,24.4869633787796,24.9767026463551,
25.4664419139307,25.9561811815063,26.4410951701193),.UNSPECIFIED.);
#2815=B_SPLINE_CURVE_WITH_KNOTS('',3,(#33736,#33737,#33738,#33739,#33740,
#33741,#33742,#33743,#33744,#33745,#33746,#33747,#33748,#33749,#33750,#33751,
#33752,#33753,#33754,#33755,#33756,#33757,#33758,#33759,#33760,#33761,#33762,
#33763,#33764,#33765,#33766,#33767,#33768,#33769,#33770,#33771,#33772,#33773,
#33774,#33775),.UNSPECIFIED.,.F.,.F.,(4,3,3,3,3,3,3,3,3,3,3,3,3,4),(-22.7045763250607,
-22.5280063084772,-22.0382670409016,-21.548527773326,-21.0587885057504,
-20.5690492381748,-20.0793099705992,-19.5895707030236,-19.0998314354481,
-18.6100921678725,-18.1203529002969,-17.6306136327213,-16.6511350975701,
-16.4213910178811),.UNSPECIFIED.);
#2816=B_SPLINE_CURVE_WITH_KNOTS('',3,(#33780,#33781,#33782,#33783,#33784,
#33785,#33786,#33787,#33788,#33789,#33790,#33791,#33792,#33793,#33794,#33795,
#33796,#33797,#33798,#33799,#33800,#33801,#33802,#33803,#33804,#33805,#33806,
#33807,#33808,#33809,#33810,#33811,#33812,#33813),.UNSPECIFIED.,.F.,.F.,
(4,3,3,3,3,3,3,3,3,3,3,4),(13.8747245557601,14.2024387596921,14.6921780272677,
15.6716565624189,16.6511350975701,17.6306136327213,18.1203529002969,18.6100921678725,
19.099831435448,19.5895707030236,20.0793099705992,20.1579098629397),
 .UNSPECIFIED.);
#2817=B_SPLINE_CURVE_WITH_KNOTS('',3,(#33814,#33815,#33816,#33817,#33818,
#33819,#33820,#33821,#33822,#33823,#33824,#33825,#33826,#33827,#33828,#33829,
#33830,#33831,#33832,#33833,#33834,#33835,#33836,#33837,#33838,#33839,#33840,
#33841,#33842,#33843,#33844,#33845,#33846,#33847,#33848,#33849,#33850),
 .UNSPECIFIED.,.F.,.F.,(4,3,3,3,3,3,3,3,3,3,3,3,4),(-16.4213910178811,-15.6716565624189,
-14.6921780272677,-14.2024387596921,-13.7126994921166,-13.222960224541,
-12.7332209569654,-12.2434816893898,-11.7537424218142,-11.2640031542386,
-10.774263886663,-10.2845246190874,-10.1382057107015),.UNSPECIFIED.);
#2818=B_SPLINE_CURVE_WITH_KNOTS('',3,(#33856,#33857,#33858,#33859,#33860,
#33861,#33862,#33863,#33864,#33865,#33866,#33867,#33868,#33869,#33870,#33871,
#33872,#33873,#33874,#33875,#33876,#33877,#33878,#33879,#33880),
 .UNSPECIFIED.,.F.,.F.,(4,3,3,3,3,3,3,3,4),(-3.85502040352192,-3.42817487302914,
-2.93843560545355,-2.44869633787796,-1.95895707030237,-1.46921780272678,
-0.979478535151181,-0.489739267575591,0.),.UNSPECIFIED.);
#2819=B_SPLINE_CURVE_WITH_KNOTS('',3,(#33883,#33884,#33885,#33886,#33887,
#33888,#33889,#33890,#33891,#33892,#33893,#33894,#33895,#33896,#33897,#33898,
#33899,#33900,#33901,#33902,#33903,#33904,#33905,#33906,#33907,#33908,#33909,
#33910,#33911,#33912,#33913,#33914,#33915,#33916,#33917,#33918,#33919),
 .UNSPECIFIED.,.F.,.F.,(4,3,3,3,3,3,3,3,3,3,3,3,4),(2.02178169133308,2.44869633787796,
2.93843560545355,3.42817487302914,3.91791414060473,4.40765340818032,4.89739267575591,
5.3871319433315,5.87687121090709,6.36661047848268,6.85634974605827,7.34608901363386,
7.59153924858054),.UNSPECIFIED.);
#2820=B_SPLINE_CURVE_WITH_KNOTS('',3,(#33925,#33926,#33927,#33928,#33929,
#33930,#33931,#33932),.UNSPECIFIED.,.F.,.F.,(4,1,1,1,1,4),(40.8407044966673,
41.2372989189625,41.7270381865381,42.2167774541137,42.7065167216893,43.1962559892649),
 .UNSPECIFIED.);
#2821=B_SPLINE_CURVE_WITH_KNOTS('',3,(#33935,#33936,#33937,#33938,#33939,
#33940,#33941,#33942,#33943,#33944),.UNSPECIFIED.,.F.,.F.,(4,1,1,1,1,1,
1,4),(40.8407044966673,40.8455297756299,41.3352690432055,41.8250083107811,
42.3147475783567,42.8044868459323,43.2942261135079,43.7211407600527),
 .UNSPECIFIED.);
#2822=B_SPLINE_CURVE_WITH_KNOTS('',3,(#33949,#33950,#33951,#33952,#33953,
#33954,#33955,#33956,#33957,#33958,#33959,#33960,#33961,#33962,#33963,#33964,
#33965),.UNSPECIFIED.,.F.,.F.,(4,1,1,1,1,1,1,1,1,1,1,1,1,1,4),(34.5575191894877,
34.8706884404798,35.3604277080554,35.850166975631,36.3399062432066,36.8296455107822,
37.3193847783578,37.8091240459334,38.298863313509,38.7886025810846,39.2783418486602,
39.7680811162357,40.2578203838113,40.7475596513869,40.8407044966673),
 .UNSPECIFIED.);
#2823=B_SPLINE_CURVE_WITH_KNOTS('',3,(#33966,#33967,#33968,#33969,#33970,
#33971,#33972,#33973,#33974,#33975,#33976,#33977,#33978,#33979,#33980,#33981),
 .UNSPECIFIED.,.F.,.F.,(4,1,1,1,1,1,1,1,1,1,1,1,1,4),(34.5575191894877,
34.9686585647228,35.4583978322984,35.948137099874,36.4378763674496,36.9276156350252,
37.4173549026008,37.9070941701764,38.396833437752,38.8865727053276,39.3763119729032,
39.8660512404787,40.3557905080543,40.8407044966673),.UNSPECIFIED.);
#2824=B_SPLINE_CURVE_WITH_KNOTS('',3,(#33986,#33987,#33988,#33989,#33990,
#33991,#33992,#33993,#33994,#33995,#33996,#33997,#33998,#33999,#34000,#34001),
 .UNSPECIFIED.,.F.,.F.,(4,1,1,1,1,1,1,1,1,1,1,1,1,4),(28.2743338823081,
28.5040779619972,29.4835564971483,29.9732957647239,30.4630350322995,30.9527742998751,
31.4425135674507,31.9322528350263,32.4219921026019,32.9117313701775,33.4014706377531,
33.8912099053287,34.3809491729042,34.5575191894877),.UNSPECIFIED.);
#2825=B_SPLINE_CURVE_WITH_KNOTS('',3,(#34002,#34003,#34004,#34005,#34006,
#34007,#34008,#34009,#34010,#34011,#34012,#34013,#34014,#34015),
 .UNSPECIFIED.,.F.,.F.,(4,1,1,1,1,1,1,1,1,1,1,4),(28.2743338823081,28.6020480862402,
29.0917873538157,30.0712658889669,31.0507444241181,32.0302229592693,32.5199622268449,
33.0097014944205,33.4994407619961,33.9891800295717,34.4789192971472,34.5575191894877),
 .UNSPECIFIED.);
#2826=B_SPLINE_CURVE_WITH_KNOTS('',3,(#34020,#34021,#34022,#34023,#34024,
#34025,#34026,#34027,#34028,#34029,#34030,#34031,#34032,#34033,#34034),
 .UNSPECIFIED.,.F.,.F.,(4,1,1,1,1,1,1,1,1,1,1,1,4),(21.9911485751285,22.1374674835145,
22.6272067510901,23.1169460186656,23.6066852862412,24.0964245538168,24.5861638213924,
25.075903088968,25.5656423565436,26.0553816241192,26.5451208916948,27.524599426846,
28.2743338823081),.UNSPECIFIED.);
#2827=B_SPLINE_CURVE_WITH_KNOTS('',3,(#34035,#34036,#34037,#34038,#34039,
#34040,#34041,#34042,#34043,#34044,#34045,#34046,#34047,#34048,#34049,#34050,
#34051),.UNSPECIFIED.,.F.,.F.,(4,1,1,1,1,1,1,1,1,1,1,1,1,1,4),(21.9911485751285,
22.2354376077575,22.7251768753331,23.2149161429087,23.7046554104842,24.1943946780598,
24.6841339456354,25.173873213211,25.6636124807866,26.1533517483622,26.6430910159378,
27.1328302835134,27.622569551089,28.1123088186646,28.2743338823081),
 .UNSPECIFIED.);
#2828=B_SPLINE_CURVE_WITH_KNOTS('',3,(#34057,#34058,#34059,#34060,#34061,
#34062),.UNSPECIFIED.,.F.,.F.,(4,1,1,4),(14.399609326548,14.8893485941236,
15.3790878616992,15.707963267949),.UNSPECIFIED.);
#2829=B_SPLINE_CURVE_WITH_KNOTS('',3,(#34065,#34066,#34067,#34068,#34069,
#34070,#34071),.UNSPECIFIED.,.F.,.F.,(4,1,1,1,4),(13.8747245557601,14.301639202305,
14.7913784698806,15.2811177374562,15.707963267949),.UNSPECIFIED.);
#2830=B_SPLINE_CURVE_WITH_KNOTS('',3,(#34077,#34078,#34079,#34080,#34081,
#34082,#34083,#34084,#34085,#34086,#34087,#34088,#34089,#34090,#34091,#34092,
#34093,#34094,#34095,#34096,#34097,#34098,#34099,#34100,#34101,#34102,#34103,
#34104,#34105,#34106,#34107,#34108,#34109,#34110),.UNSPECIFIED.,.F.,.F.,
(4,3,3,3,3,3,3,3,3,3,3,4),(26.4410951701193,26.4459204490819,26.9356597166575,
27.4253989842331,27.9151382518087,28.4048775193843,28.8946167869599,29.3843560545355,
29.8740953221111,30.3638345896866,30.8535738572622,31.3433131248378),
 .UNSPECIFIED.);
#2831=B_SPLINE_CURVE_WITH_KNOTS('',3,(#34114,#34115,#34116,#34117),
 .UNSPECIFIED.,.F.,.F.,(4,4),(-29.3215314335047,-28.9877616322403),
 .UNSPECIFIED.);
#2832=B_SPLINE_CURVE_WITH_KNOTS('',3,(#34121,#34122,#34123,#34124,#34125,
#34126,#34127,#34128,#34129,#34130,#34131,#34132,#34133,#34134,#34135,#34136,
#34137,#34138,#34139,#34140,#34141,#34142,#34143,#34144,#34145,#34146,#34147,
#34148,#34149,#34150,#34151,#34152,#34153,#34154,#34155,#34156,#34157,#34158,
#34159,#34160,#34161,#34162,#34163),.UNSPECIFIED.,.F.,.F.,(4,3,3,3,3,3,
3,3,3,3,3,3,3,3,4),(-28.9877616322403,-28.8946167869599,-28.4048775193843,
-27.9151382518087,-27.4253989842331,-26.9356597166575,-26.4459204490819,
-25.9561811815063,-25.4664419139307,-24.9767026463551,-24.4869633787795,
-23.997224111204,-23.5074848436284,-23.0177455760528,-22.7045763250607),
 .UNSPECIFIED.);
#2833=B_SPLINE_CURVE_WITH_KNOTS('',3,(#34168,#34169,#34170,#34171,#34172,
#34173,#34174,#34175,#34176,#34177,#34178,#34179,#34180,#34181,#34182,#34183,
#34184,#34185,#34186,#34187,#34188,#34189,#34190,#34191,#34192,#34193,#34194,
#34195,#34196,#34197,#34198,#34199,#34200,#34201,#34202,#34203,#34204,#34205,
#34206,#34207),.UNSPECIFIED.,.F.,.F.,(4,3,3,3,3,3,3,3,3,3,3,3,3,4),(20.1579098629397,
20.5690492381748,21.0587885057504,21.548527773326,22.0382670409016,22.5280063084772,
23.0177455760528,23.5074848436284,23.997224111204,24.4869633787795,24.9767026463551,
25.4664419139307,25.9561811815063,26.4410951701193),.UNSPECIFIED.);
#2834=B_SPLINE_CURVE_WITH_KNOTS('',3,(#34208,#34209,#34210,#34211,#34212,
#34213,#34214,#34215,#34216,#34217,#34218,#34219,#34220,#34221,#34222,#34223,
#34224,#34225,#34226,#34227,#34228,#34229,#34230,#34231,#34232,#34233,#34234,
#34235,#34236,#34237,#34238,#34239,#34240,#34241,#34242,#34243,#34244,#34245,
#34246,#34247),.UNSPECIFIED.,.F.,.F.,(4,3,3,3,3,3,3,3,3,3,3,3,3,4),(-22.7045763250607,
-22.5280063084772,-22.0382670409016,-21.548527773326,-21.0587885057504,
-20.5690492381748,-20.0793099705992,-19.5895707030236,-19.099831435448,
-18.6100921678725,-18.1203529002969,-17.6306136327213,-16.6511350975701,
-16.4213910178811),.UNSPECIFIED.);
#2835=B_SPLINE_CURVE_WITH_KNOTS('',3,(#34252,#34253,#34254,#34255,#34256,
#34257,#34258,#34259,#34260,#34261,#34262,#34263,#34264,#34265,#34266,#34267,
#34268,#34269,#34270,#34271,#34272,#34273,#34274,#34275,#34276,#34277,#34278,
#34279,#34280,#34281,#34282,#34283,#34284,#34285),.UNSPECIFIED.,.F.,.F.,
(4,3,3,3,3,3,3,3,3,3,3,4),(13.8747245557601,14.2024387596921,14.6921780272677,
15.6716565624189,16.6511350975701,17.6306136327213,18.1203529002969,18.6100921678725,
19.099831435448,19.5895707030236,20.0793099705992,20.1579098629397),
 .UNSPECIFIED.);
#2836=B_SPLINE_CURVE_WITH_KNOTS('',3,(#34286,#34287,#34288,#34289,#34290,
#34291,#34292,#34293,#34294,#34295,#34296,#34297,#34298,#34299,#34300,#34301,
#34302,#34303,#34304,#34305,#34306,#34307,#34308,#34309,#34310,#34311,#34312,
#34313,#34314,#34315,#34316,#34317,#34318,#34319,#34320,#34321,#34322),
 .UNSPECIFIED.,.F.,.F.,(4,3,3,3,3,3,3,3,3,3,3,3,4),(-16.4213910178811,-15.6716565624189,
-14.6921780272677,-14.2024387596921,-13.7126994921165,-13.222960224541,
-12.7332209569654,-12.2434816893898,-11.7537424218142,-11.2640031542386,
-10.774263886663,-10.2845246190874,-10.1382057107015),.UNSPECIFIED.);
#2837=B_SPLINE_CURVE_WITH_KNOTS('',3,(#34328,#34329,#34330,#34331,#34332,
#34333,#34334,#34335,#34336,#34337,#34338,#34339,#34340,#34341,#34342,#34343,
#34344,#34345,#34346,#34347,#34348,#34349,#34350,#34351,#34352),
 .UNSPECIFIED.,.F.,.F.,(4,3,3,3,3,3,3,3,4),(-3.85502040352192,-3.42817487302914,
-2.93843560545354,-2.44869633787795,-1.95895707030236,-1.46921780272677,
-0.979478535151182,-0.489739267575592,0.),.UNSPECIFIED.);
#2838=B_SPLINE_CURVE_WITH_KNOTS('',3,(#34355,#34356,#34357,#34358,#34359,
#34360,#34361,#34362,#34363,#34364,#34365,#34366,#34367,#34368,#34369,#34370,
#34371,#34372,#34373,#34374,#34375,#34376,#34377,#34378,#34379,#34380,#34381,
#34382,#34383,#34384,#34385,#34386,#34387,#34388,#34389,#34390,#34391),
 .UNSPECIFIED.,.F.,.F.,(4,3,3,3,3,3,3,3,3,3,3,3,4),(2.02178169133309,2.44869633787795,
2.93843560545354,3.42817487302914,3.91791414060473,4.40765340818032,4.89739267575591,
5.3871319433315,5.87687121090709,6.36661047848268,6.85634974605827,7.34608901363386,
7.59153924858054),.UNSPECIFIED.);
#2839=B_SPLINE_CURVE_WITH_KNOTS('',3,(#34397,#34398,#34399,#34400,#34401,
#34402,#34403,#34404),.UNSPECIFIED.,.F.,.F.,(4,1,1,1,1,4),(40.8407044966673,
41.2372989189625,41.7270381865381,42.2167774541137,42.7065167216893,43.1962559892649),
 .UNSPECIFIED.);
#2840=B_SPLINE_CURVE_WITH_KNOTS('',3,(#34407,#34408,#34409,#34410,#34411,
#34412,#34413,#34414,#34415,#34416),.UNSPECIFIED.,.F.,.F.,(4,1,1,1,1,1,
1,4),(40.8407044966673,40.8455297756299,41.3352690432055,41.8250083107811,
42.3147475783567,42.8044868459323,43.2942261135079,43.7211407600527),
 .UNSPECIFIED.);
#2841=B_SPLINE_CURVE_WITH_KNOTS('',3,(#34421,#34422,#34423,#34424,#34425,
#34426,#34427,#34428,#34429,#34430,#34431,#34432,#34433,#34434,#34435,#34436,
#34437),.UNSPECIFIED.,.F.,.F.,(4,1,1,1,1,1,1,1,1,1,1,1,1,1,4),(34.5575191894877,
34.8706884404798,35.3604277080554,35.850166975631,36.3399062432066,36.8296455107822,
37.3193847783578,37.8091240459334,38.298863313509,38.7886025810846,39.2783418486601,
39.7680811162357,40.2578203838113,40.7475596513869,40.8407044966673),
 .UNSPECIFIED.);
#2842=B_SPLINE_CURVE_WITH_KNOTS('',3,(#34438,#34439,#34440,#34441,#34442,
#34443,#34444,#34445,#34446,#34447,#34448,#34449,#34450,#34451,#34452,#34453),
 .UNSPECIFIED.,.F.,.F.,(4,1,1,1,1,1,1,1,1,1,1,1,1,4),(34.5575191894877,
34.9686585647228,35.4583978322984,35.948137099874,36.4378763674496,36.9276156350252,
37.4173549026008,37.9070941701764,38.396833437752,38.8865727053276,39.3763119729032,
39.8660512404787,40.3557905080543,40.8407044966673),.UNSPECIFIED.);
#2843=B_SPLINE_CURVE_WITH_KNOTS('',3,(#34458,#34459,#34460,#34461,#34462,
#34463,#34464,#34465,#34466,#34467,#34468,#34469,#34470,#34471,#34472,#34473),
 .UNSPECIFIED.,.F.,.F.,(4,1,1,1,1,1,1,1,1,1,1,1,1,4),(28.2743338823081,
28.5040779619971,29.4835564971483,29.9732957647239,30.4630350322995,30.9527742998751,
31.4425135674507,31.9322528350263,32.4219921026019,32.9117313701775,33.4014706377531,
33.8912099053287,34.3809491729042,34.5575191894877),.UNSPECIFIED.);
#2844=B_SPLINE_CURVE_WITH_KNOTS('',3,(#34474,#34475,#34476,#34477,#34478,
#34479,#34480,#34481,#34482,#34483,#34484,#34485,#34486,#34487),
 .UNSPECIFIED.,.F.,.F.,(4,1,1,1,1,1,1,1,1,1,1,4),(28.2743338823081,28.6020480862402,
29.0917873538157,30.0712658889669,31.0507444241181,32.0302229592693,32.5199622268449,
33.0097014944205,33.4994407619961,33.9891800295717,34.4789192971472,34.5575191894877),
 .UNSPECIFIED.);
#2845=B_SPLINE_CURVE_WITH_KNOTS('',3,(#34492,#34493,#34494,#34495,#34496,
#34497,#34498,#34499,#34500,#34501,#34502,#34503,#34504,#34505,#34506),
 .UNSPECIFIED.,.F.,.F.,(4,1,1,1,1,1,1,1,1,1,1,1,4),(21.9911485751285,22.1374674835145,
22.6272067510901,23.1169460186656,23.6066852862412,24.0964245538168,24.5861638213924,
25.075903088968,25.5656423565436,26.0553816241192,26.5451208916948,27.524599426846,
28.2743338823081),.UNSPECIFIED.);
#2846=B_SPLINE_CURVE_WITH_KNOTS('',3,(#34507,#34508,#34509,#34510,#34511,
#34512,#34513,#34514,#34515,#34516,#34517,#34518,#34519,#34520,#34521,#34522,
#34523),.UNSPECIFIED.,.F.,.F.,(4,1,1,1,1,1,1,1,1,1,1,1,1,1,4),(21.9911485751285,
22.2354376077575,22.7251768753331,23.2149161429087,23.7046554104842,24.1943946780598,
24.6841339456354,25.173873213211,25.6636124807866,26.1533517483622,26.6430910159378,
27.1328302835134,27.622569551089,28.1123088186646,28.2743338823081),
 .UNSPECIFIED.);
#2847=B_SPLINE_CURVE_WITH_KNOTS('',3,(#34529,#34530,#34531,#34532,#34533,
#34534),.UNSPECIFIED.,.F.,.F.,(4,1,1,4),(14.399609326548,14.8893485941236,
15.3790878616992,15.707963267949),.UNSPECIFIED.);
#2848=B_SPLINE_CURVE_WITH_KNOTS('',3,(#34537,#34538,#34539,#34540,#34541,
#34542,#34543),.UNSPECIFIED.,.F.,.F.,(4,1,1,1,4),(13.8747245557601,14.301639202305,
14.7913784698806,15.2811177374562,15.707963267949),.UNSPECIFIED.);
#2849=B_SPLINE_CURVE_WITH_KNOTS('',3,(#34549,#34550,#34551,#34552,#34553,
#34554,#34555,#34556,#34557,#34558,#34559,#34560,#34561,#34562,#34563,#34564,
#34565,#34566,#34567,#34568,#34569,#34570,#34571,#34572,#34573,#34574,#34575,
#34576,#34577,#34578,#34579,#34580,#34581,#34582),.UNSPECIFIED.,.F.,.F.,
(4,3,3,3,3,3,3,3,3,3,3,4),(26.4410951701193,26.4459204490819,26.9356597166575,
27.4253989842331,27.9151382518087,28.4048775193843,28.8946167869599,29.3843560545355,
29.874095322111,30.3638345896866,30.8535738572622,31.3433131248378),
 .UNSPECIFIED.);
#2850=B_SPLINE_CURVE_WITH_KNOTS('',3,(#34586,#34587,#34588,#34589),
 .UNSPECIFIED.,.F.,.F.,(4,4),(-29.3215314335047,-28.9877616322403),
 .UNSPECIFIED.);
#2851=B_SPLINE_CURVE_WITH_KNOTS('',3,(#34593,#34594,#34595,#34596,#34597,
#34598,#34599,#34600,#34601,#34602,#34603,#34604,#34605,#34606,#34607,#34608,
#34609,#34610,#34611,#34612,#34613,#34614,#34615,#34616,#34617,#34618,#34619,
#34620,#34621,#34622,#34623,#34624,#34625,#34626,#34627,#34628,#34629,#34630,
#34631,#34632,#34633,#34634,#34635),.UNSPECIFIED.,.F.,.F.,(4,3,3,3,3,3,
3,3,3,3,3,3,3,3,4),(-28.9877616322403,-28.8946167869599,-28.4048775193843,
-27.9151382518087,-27.4253989842331,-26.9356597166575,-26.4459204490819,
-25.9561811815063,-25.4664419139307,-24.9767026463552,-24.4869633787796,
-23.997224111204,-23.5074848436284,-23.0177455760528,-22.7045763250607),
 .UNSPECIFIED.);
#2852=B_SPLINE_CURVE_WITH_KNOTS('',3,(#34640,#34641,#34642,#34643,#34644,
#34645,#34646,#34647,#34648,#34649,#34650,#34651,#34652,#34653,#34654,#34655,
#34656,#34657,#34658,#34659,#34660,#34661,#34662,#34663,#34664,#34665,#34666,
#34667,#34668,#34669,#34670,#34671,#34672,#34673,#34674,#34675,#34676,#34677,
#34678,#34679),.UNSPECIFIED.,.F.,.F.,(4,3,3,3,3,3,3,3,3,3,3,3,3,4),(20.1579098629397,
20.5690492381748,21.0587885057504,21.548527773326,22.0382670409016,22.5280063084772,
23.0177455760528,23.5074848436284,23.997224111204,24.4869633787795,24.9767026463551,
25.4664419139307,25.9561811815063,26.4410951701193),.UNSPECIFIED.);
#2853=B_SPLINE_CURVE_WITH_KNOTS('',3,(#34680,#34681,#34682,#34683,#34684,
#34685,#34686,#34687,#34688,#34689,#34690,#34691,#34692,#34693,#34694,#34695,
#34696,#34697,#34698,#34699,#34700,#34701,#34702,#34703,#34704,#34705,#34706,
#34707,#34708,#34709,#34710,#34711,#34712,#34713,#34714,#34715,#34716,#34717,
#34718,#34719),.UNSPECIFIED.,.F.,.F.,(4,3,3,3,3,3,3,3,3,3,3,3,3,4),(-22.7045763250607,
-22.5280063084772,-22.0382670409016,-21.548527773326,-21.0587885057504,
-20.5690492381748,-20.0793099705992,-19.5895707030236,-19.0998314354481,
-18.6100921678725,-18.1203529002969,-17.6306136327213,-16.6511350975701,
-16.4213910178811),.UNSPECIFIED.);
#2854=B_SPLINE_CURVE_WITH_KNOTS('',3,(#34724,#34725,#34726,#34727,#34728,
#34729,#34730,#34731,#34732,#34733,#34734,#34735,#34736,#34737,#34738,#34739,
#34740,#34741,#34742,#34743,#34744,#34745,#34746,#34747,#34748,#34749,#34750,
#34751,#34752,#34753,#34754,#34755,#34756,#34757),.UNSPECIFIED.,.F.,.F.,
(4,3,3,3,3,3,3,3,3,3,3,4),(13.8747245557601,14.2024387596921,14.6921780272677,
15.6716565624189,16.6511350975701,17.6306136327213,18.1203529002969,18.6100921678725,
19.0998314354481,19.5895707030236,20.0793099705992,20.1579098629397),
 .UNSPECIFIED.);
#2855=B_SPLINE_CURVE_WITH_KNOTS('',3,(#34758,#34759,#34760,#34761,#34762,
#34763,#34764,#34765,#34766,#34767,#34768,#34769,#34770,#34771,#34772,#34773,
#34774,#34775,#34776,#34777,#34778,#34779,#34780,#34781,#34782,#34783,#34784,
#34785,#34786,#34787,#34788,#34789,#34790,#34791,#34792,#34793,#34794),
 .UNSPECIFIED.,.F.,.F.,(4,3,3,3,3,3,3,3,3,3,3,3,4),(-16.4213910178811,-15.6716565624189,
-14.6921780272677,-14.2024387596921,-13.7126994921165,-13.222960224541,
-12.7332209569654,-12.2434816893898,-11.7537424218142,-11.2640031542386,
-10.774263886663,-10.2845246190874,-10.1382057107015),.UNSPECIFIED.);
#2856=B_SPLINE_CURVE_WITH_KNOTS('',3,(#34800,#34801,#34802,#34803,#34804,
#34805,#34806,#34807,#34808,#34809,#34810,#34811,#34812,#34813,#34814,#34815,
#34816,#34817,#34818,#34819,#34820,#34821,#34822,#34823,#34824),
 .UNSPECIFIED.,.F.,.F.,(4,3,3,3,3,3,3,3,4),(-3.85502040352192,-3.42817487302914,
-2.93843560545355,-2.44869633787795,-1.95895707030236,-1.46921780272677,
-0.979478535151183,-0.489739267575592,0.),.UNSPECIFIED.);
#2857=B_SPLINE_CURVE_WITH_KNOTS('',3,(#34827,#34828,#34829,#34830,#34831,
#34832,#34833,#34834,#34835,#34836,#34837,#34838,#34839,#34840,#34841,#34842,
#34843,#34844,#34845,#34846,#34847,#34848,#34849,#34850,#34851,#34852,#34853,
#34854,#34855,#34856,#34857,#34858,#34859,#34860,#34861,#34862,#34863),
 .UNSPECIFIED.,.F.,.F.,(4,3,3,3,3,3,3,3,3,3,3,3,4),(2.02178169133308,2.44869633787795,
2.93843560545355,3.42817487302914,3.91791414060473,4.40765340818032,4.89739267575591,
5.3871319433315,5.87687121090709,6.36661047848268,6.85634974605827,7.34608901363386,
7.59153924858054),.UNSPECIFIED.);
#2858=B_SPLINE_CURVE_WITH_KNOTS('',3,(#34869,#34870,#34871,#34872,#34873,
#34874,#34875,#34876),.UNSPECIFIED.,.F.,.F.,(4,1,1,1,1,4),(40.8407044966673,
41.2372989189625,41.7270381865381,42.2167774541137,42.7065167216893,43.1962559892649),
 .UNSPECIFIED.);
#2859=B_SPLINE_CURVE_WITH_KNOTS('',3,(#34879,#34880,#34881,#34882,#34883,
#34884,#34885,#34886,#34887,#34888),.UNSPECIFIED.,.F.,.F.,(4,1,1,1,1,1,
1,4),(40.8407044966673,40.8455297756299,41.3352690432055,41.8250083107811,
42.3147475783567,42.8044868459323,43.2942261135079,43.7211407600527),
 .UNSPECIFIED.);
#2860=B_SPLINE_CURVE_WITH_KNOTS('',3,(#34893,#34894,#34895,#34896,#34897,
#34898,#34899,#34900,#34901,#34902,#34903,#34904,#34905,#34906,#34907,#34908,
#34909),.UNSPECIFIED.,.F.,.F.,(4,1,1,1,1,1,1,1,1,1,1,1,1,1,4),(34.5575191894877,
34.8706884404798,35.3604277080554,35.850166975631,36.3399062432066,36.8296455107822,
37.3193847783578,37.8091240459334,38.298863313509,38.7886025810846,39.2783418486601,
39.7680811162357,40.2578203838113,40.7475596513869,40.8407044966673),
 .UNSPECIFIED.);
#2861=B_SPLINE_CURVE_WITH_KNOTS('',3,(#34910,#34911,#34912,#34913,#34914,
#34915,#34916,#34917,#34918,#34919,#34920,#34921,#34922,#34923,#34924,#34925),
 .UNSPECIFIED.,.F.,.F.,(4,1,1,1,1,1,1,1,1,1,1,1,1,4),(34.5575191894877,
34.9686585647228,35.4583978322984,35.948137099874,36.4378763674496,36.9276156350252,
37.4173549026008,37.9070941701764,38.396833437752,38.8865727053276,39.3763119729032,
39.8660512404787,40.3557905080543,40.8407044966673),.UNSPECIFIED.);
#2862=B_SPLINE_CURVE_WITH_KNOTS('',3,(#34930,#34931,#34932,#34933,#34934,
#34935,#34936,#34937,#34938,#34939,#34940,#34941,#34942,#34943,#34944,#34945),
 .UNSPECIFIED.,.F.,.F.,(4,1,1,1,1,1,1,1,1,1,1,1,1,4),(28.2743338823081,
28.5040779619971,29.4835564971483,29.9732957647239,30.4630350322995,30.9527742998751,
31.4425135674507,31.9322528350263,32.4219921026019,32.9117313701775,33.4014706377531,
33.8912099053287,34.3809491729042,34.5575191894877),.UNSPECIFIED.);
#2863=B_SPLINE_CURVE_WITH_KNOTS('',3,(#34946,#34947,#34948,#34949,#34950,
#34951,#34952,#34953,#34954,#34955,#34956,#34957,#34958,#34959),
 .UNSPECIFIED.,.F.,.F.,(4,1,1,1,1,1,1,1,1,1,1,4),(28.2743338823081,28.6020480862402,
29.0917873538157,30.0712658889669,31.0507444241181,32.0302229592693,32.5199622268449,
33.0097014944205,33.4994407619961,33.9891800295717,34.4789192971472,34.5575191894877),
 .UNSPECIFIED.);
#2864=B_SPLINE_CURVE_WITH_KNOTS('',3,(#34964,#34965,#34966,#34967,#34968,
#34969,#34970,#34971,#34972,#34973,#34974,#34975,#34976,#34977,#34978),
 .UNSPECIFIED.,.F.,.F.,(4,1,1,1,1,1,1,1,1,1,1,1,4),(21.9911485751285,22.1374674835145,
22.6272067510901,23.1169460186656,23.6066852862412,24.0964245538168,24.5861638213924,
25.075903088968,25.5656423565436,26.0553816241192,26.5451208916948,27.524599426846,
28.2743338823081),.UNSPECIFIED.);
#2865=B_SPLINE_CURVE_WITH_KNOTS('',3,(#34979,#34980,#34981,#34982,#34983,
#34984,#34985,#34986,#34987,#34988,#34989,#34990,#34991,#34992,#34993,#34994,
#34995),.UNSPECIFIED.,.F.,.F.,(4,1,1,1,1,1,1,1,1,1,1,1,1,1,4),(21.9911485751285,
22.2354376077575,22.7251768753331,23.2149161429087,23.7046554104842,24.1943946780598,
24.6841339456354,25.173873213211,25.6636124807866,26.1533517483622,26.6430910159378,
27.1328302835134,27.622569551089,28.1123088186646,28.2743338823081),
 .UNSPECIFIED.);
#2866=B_SPLINE_CURVE_WITH_KNOTS('',3,(#35001,#35002,#35003,#35004,#35005,
#35006),.UNSPECIFIED.,.F.,.F.,(4,1,1,4),(14.399609326548,14.8893485941236,
15.3790878616992,15.707963267949),.UNSPECIFIED.);
#2867=B_SPLINE_CURVE_WITH_KNOTS('',3,(#35009,#35010,#35011,#35012,#35013,
#35014,#35015),.UNSPECIFIED.,.F.,.F.,(4,1,1,1,4),(13.8747245557601,14.301639202305,
14.7913784698806,15.2811177374562,15.707963267949),.UNSPECIFIED.);
#2868=B_SPLINE_CURVE_WITH_KNOTS('',3,(#35021,#35022,#35023,#35024,#35025,
#35026,#35027,#35028,#35029,#35030,#35031,#35032,#35033,#35034,#35035,#35036,
#35037,#35038,#35039,#35040,#35041,#35042,#35043,#35044,#35045,#35046,#35047,
#35048,#35049,#35050,#35051,#35052,#35053,#35054),.UNSPECIFIED.,.F.,.F.,
(4,3,3,3,3,3,3,3,3,3,3,4),(26.4410951701193,26.4459204490819,26.9356597166575,
27.4253989842331,27.9151382518087,28.4048775193843,28.8946167869599,29.3843560545355,
29.874095322111,30.3638345896866,30.8535738572622,31.3433131248378),
 .UNSPECIFIED.);
#2869=B_SPLINE_CURVE_WITH_KNOTS('',3,(#35058,#35059,#35060,#35061),
 .UNSPECIFIED.,.F.,.F.,(4,4),(-29.3215314335047,-28.9877616322403),
 .UNSPECIFIED.);
#2870=B_SPLINE_CURVE_WITH_KNOTS('',3,(#35065,#35066,#35067,#35068,#35069,
#35070,#35071,#35072,#35073,#35074,#35075,#35076,#35077,#35078,#35079,#35080,
#35081,#35082,#35083,#35084,#35085,#35086,#35087,#35088,#35089,#35090,#35091,
#35092,#35093,#35094,#35095,#35096,#35097,#35098,#35099,#35100,#35101,#35102,
#35103,#35104,#35105,#35106,#35107),.UNSPECIFIED.,.F.,.F.,(4,3,3,3,3,3,
3,3,3,3,3,3,3,3,4),(-28.9877616322403,-28.8946167869599,-28.4048775193843,
-27.9151382518087,-27.4253989842331,-26.9356597166575,-26.4459204490819,
-25.9561811815063,-25.4664419139307,-24.9767026463552,-24.4869633787796,
-23.997224111204,-23.5074848436284,-23.0177455760528,-22.7045763250607),
 .UNSPECIFIED.);
#2871=B_SPLINE_CURVE_WITH_KNOTS('',3,(#35112,#35113,#35114,#35115,#35116,
#35117,#35118,#35119,#35120,#35121,#35122,#35123,#35124,#35125,#35126,#35127,
#35128,#35129,#35130,#35131,#35132,#35133,#35134,#35135,#35136,#35137,#35138,
#35139,#35140,#35141,#35142,#35143,#35144,#35145,#35146,#35147,#35148,#35149,
#35150,#35151),.UNSPECIFIED.,.F.,.F.,(4,3,3,3,3,3,3,3,3,3,3,3,3,4),(20.1579098629397,
20.5690492381748,21.0587885057504,21.548527773326,22.0382670409016,22.5280063084772,
23.0177455760528,23.5074848436284,23.997224111204,24.4869633787796,24.9767026463551,
25.4664419139307,25.9561811815063,26.4410951701193),.UNSPECIFIED.);
#2872=B_SPLINE_CURVE_WITH_KNOTS('',3,(#35152,#35153,#35154,#35155,#35156,
#35157,#35158,#35159,#35160,#35161,#35162,#35163,#35164,#35165,#35166,#35167,
#35168,#35169,#35170,#35171,#35172,#35173,#35174,#35175,#35176,#35177,#35178,
#35179,#35180,#35181,#35182,#35183,#35184,#35185,#35186,#35187,#35188,#35189,
#35190,#35191),.UNSPECIFIED.,.F.,.F.,(4,3,3,3,3,3,3,3,3,3,3,3,3,4),(-22.7045763250607,
-22.5280063084772,-22.0382670409016,-21.548527773326,-21.0587885057504,
-20.5690492381748,-20.0793099705992,-19.5895707030236,-19.0998314354481,
-18.6100921678725,-18.1203529002969,-17.6306136327213,-16.6511350975701,
-16.4213910178811),.UNSPECIFIED.);
#2873=B_SPLINE_CURVE_WITH_KNOTS('',3,(#35196,#35197,#35198,#35199,#35200,
#35201,#35202,#35203,#35204,#35205,#35206,#35207,#35208,#35209,#35210,#35211,
#35212,#35213,#35214,#35215,#35216,#35217,#35218,#35219,#35220,#35221,#35222,
#35223,#35224,#35225,#35226,#35227,#35228,#35229),.UNSPECIFIED.,.F.,.F.,
(4,3,3,3,3,3,3,3,3,3,3,4),(13.8747245557601,14.2024387596921,14.6921780272677,
15.6716565624189,16.6511350975701,17.6306136327213,18.1203529002969,18.6100921678725,
19.0998314354481,19.5895707030236,20.0793099705992,20.1579098629397),
 .UNSPECIFIED.);
#2874=B_SPLINE_CURVE_WITH_KNOTS('',3,(#35230,#35231,#35232,#35233,#35234,
#35235,#35236,#35237,#35238,#35239,#35240,#35241,#35242,#35243,#35244,#35245,
#35246,#35247,#35248,#35249,#35250,#35251,#35252,#35253,#35254,#35255,#35256,
#35257,#35258,#35259,#35260,#35261,#35262,#35263,#35264,#35265,#35266),
 .UNSPECIFIED.,.F.,.F.,(4,3,3,3,3,3,3,3,3,3,3,3,4),(-16.4213910178811,-15.6716565624189,
-14.6921780272677,-14.2024387596921,-13.7126994921165,-13.222960224541,
-12.7332209569654,-12.2434816893898,-11.7537424218142,-11.2640031542386,
-10.774263886663,-10.2845246190874,-10.1382057107015),.UNSPECIFIED.);
#2875=B_SPLINE_CURVE_WITH_KNOTS('',3,(#35272,#35273,#35274,#35275,#35276,
#35277,#35278,#35279,#35280,#35281,#35282,#35283,#35284,#35285,#35286,#35287,
#35288,#35289,#35290,#35291,#35292,#35293,#35294,#35295,#35296),
 .UNSPECIFIED.,.F.,.F.,(4,3,3,3,3,3,3,3,4),(-3.85502040352192,-3.42817487302914,
-2.93843560545355,-2.44869633787795,-1.95895707030236,-1.46921780272677,
-0.979478535151183,-0.489739267575592,0.),.UNSPECIFIED.);
#2876=B_SPLINE_CURVE_WITH_KNOTS('',3,(#35299,#35300,#35301,#35302,#35303,
#35304,#35305,#35306,#35307,#35308,#35309,#35310,#35311,#35312,#35313,#35314,
#35315,#35316,#35317,#35318,#35319,#35320,#35321,#35322,#35323,#35324,#35325,
#35326,#35327,#35328,#35329,#35330,#35331,#35332,#35333,#35334,#35335),
 .UNSPECIFIED.,.F.,.F.,(4,3,3,3,3,3,3,3,3,3,3,3,4),(2.02178169133309,2.44869633787795,
2.93843560545355,3.42817487302914,3.91791414060473,4.40765340818032,4.89739267575591,
5.3871319433315,5.87687121090709,6.36661047848268,6.85634974605827,7.34608901363386,
7.59153924858054),.UNSPECIFIED.);
#2877=B_SPLINE_CURVE_WITH_KNOTS('',3,(#35341,#35342,#35343,#35344,#35345,
#35346,#35347,#35348),.UNSPECIFIED.,.F.,.F.,(4,1,1,1,1,4),(40.8407044966673,
41.2372989189625,41.7270381865381,42.2167774541137,42.7065167216893,43.1962559892649),
 .UNSPECIFIED.);
#2878=B_SPLINE_CURVE_WITH_KNOTS('',3,(#35351,#35352,#35353,#35354,#35355,
#35356,#35357,#35358,#35359,#35360),.UNSPECIFIED.,.F.,.F.,(4,1,1,1,1,1,
1,4),(40.8407044966673,40.8455297756299,41.3352690432055,41.8250083107811,
42.3147475783567,42.8044868459323,43.2942261135079,43.7211407600527),
 .UNSPECIFIED.);
#2879=B_SPLINE_CURVE_WITH_KNOTS('',3,(#35365,#35366,#35367,#35368,#35369,
#35370,#35371,#35372,#35373,#35374,#35375,#35376,#35377,#35378,#35379,#35380,
#35381),.UNSPECIFIED.,.F.,.F.,(4,1,1,1,1,1,1,1,1,1,1,1,1,1,4),(34.5575191894877,
34.8706884404798,35.3604277080554,35.850166975631,36.3399062432066,36.8296455107822,
37.3193847783578,37.8091240459334,38.298863313509,38.7886025810846,39.2783418486601,
39.7680811162357,40.2578203838113,40.7475596513869,40.8407044966673),
 .UNSPECIFIED.);
#2880=B_SPLINE_CURVE_WITH_KNOTS('',3,(#35382,#35383,#35384,#35385,#35386,
#35387,#35388,#35389,#35390,#35391,#35392,#35393,#35394,#35395,#35396,#35397),
 .UNSPECIFIED.,.F.,.F.,(4,1,1,1,1,1,1,1,1,1,1,1,1,4),(34.5575191894877,
34.9686585647228,35.4583978322984,35.948137099874,36.4378763674496,36.9276156350252,
37.4173549026008,37.9070941701764,38.396833437752,38.8865727053276,39.3763119729032,
39.8660512404787,40.3557905080543,40.8407044966673),.UNSPECIFIED.);
#2881=B_SPLINE_CURVE_WITH_KNOTS('',3,(#35402,#35403,#35404,#35405,#35406,
#35407,#35408,#35409,#35410,#35411,#35412,#35413,#35414,#35415,#35416,#35417),
 .UNSPECIFIED.,.F.,.F.,(4,1,1,1,1,1,1,1,1,1,1,1,1,4),(28.2743338823081,
28.5040779619971,29.4835564971483,29.9732957647239,30.4630350322995,30.9527742998751,
31.4425135674507,31.9322528350263,32.4219921026019,32.9117313701775,33.4014706377531,
33.8912099053287,34.3809491729042,34.5575191894877),.UNSPECIFIED.);
#2882=B_SPLINE_CURVE_WITH_KNOTS('',3,(#35418,#35419,#35420,#35421,#35422,
#35423,#35424,#35425,#35426,#35427,#35428,#35429,#35430,#35431),
 .UNSPECIFIED.,.F.,.F.,(4,1,1,1,1,1,1,1,1,1,1,4),(28.2743338823081,28.6020480862402,
29.0917873538157,30.0712658889669,31.0507444241181,32.0302229592693,32.5199622268449,
33.0097014944205,33.4994407619961,33.9891800295717,34.4789192971472,34.5575191894877),
 .UNSPECIFIED.);
#2883=B_SPLINE_CURVE_WITH_KNOTS('',3,(#35436,#35437,#35438,#35439,#35440,
#35441,#35442,#35443,#35444,#35445,#35446,#35447,#35448,#35449,#35450),
 .UNSPECIFIED.,.F.,.F.,(4,1,1,1,1,1,1,1,1,1,1,1,4),(21.9911485751285,22.1374674835145,
22.6272067510901,23.1169460186656,23.6066852862412,24.0964245538168,24.5861638213924,
25.075903088968,25.5656423565436,26.0553816241192,26.5451208916948,27.524599426846,
28.2743338823081),.UNSPECIFIED.);
#2884=B_SPLINE_CURVE_WITH_KNOTS('',3,(#35451,#35452,#35453,#35454,#35455,
#35456,#35457,#35458,#35459,#35460,#35461,#35462,#35463,#35464,#35465,#35466,
#35467),.UNSPECIFIED.,.F.,.F.,(4,1,1,1,1,1,1,1,1,1,1,1,1,1,4),(21.9911485751285,
22.2354376077575,22.7251768753331,23.2149161429087,23.7046554104842,24.1943946780598,
24.6841339456354,25.173873213211,25.6636124807866,26.1533517483622,26.6430910159378,
27.1328302835134,27.622569551089,28.1123088186646,28.2743338823081),
 .UNSPECIFIED.);
#2885=B_SPLINE_CURVE_WITH_KNOTS('',3,(#35473,#35474,#35475,#35476,#35477,
#35478),.UNSPECIFIED.,.F.,.F.,(4,1,1,4),(14.399609326548,14.8893485941236,
15.3790878616992,15.707963267949),.UNSPECIFIED.);
#2886=B_SPLINE_CURVE_WITH_KNOTS('',3,(#35481,#35482,#35483,#35484,#35485,
#35486,#35487),.UNSPECIFIED.,.F.,.F.,(4,1,1,1,4),(13.8747245557601,14.301639202305,
14.7913784698806,15.2811177374562,15.707963267949),.UNSPECIFIED.);
#2887=B_SPLINE_CURVE_WITH_KNOTS('',3,(#35489,#35490,#35491,#35492,#35493,
#35494,#35495,#35496,#35497,#35498,#35499,#35500,#35501,#35502,#35503,#35504,
#35505,#35506,#35507,#35508,#35509,#35510,#35511,#35512,#35513,#35514,#35515,
#35516,#35517,#35518,#35519,#35520,#35521,#35522,#35523,#35524,#35525,#35526,
#35527,#35528,#35529,#35530,#35531,#35532,#35533,#35534,#35535,#35536,#35537,
#35538,#35539,#35540,#35541,#35542,#35543,#35544,#35545,#35546,#35547,#35548,
#35549,#35550,#35551,#35552,#35553,#35554,#35555,#35556,#35557,#35558,#35559,
#35560,#35561,#35562,#35563,#35564,#35565,#35566,#35567,#35568,#35569,#35570,
#35571,#35572,#35573,#35574,#35575,#35576,#35577,#35578,#35579,#35580,#35581,
#35582,#35583,#35584,#35585,#35586,#35587,#35588,#35589,#35590,#35591,#35592,
#35593,#35594,#35595,#35596,#35597),.UNSPECIFIED.,.F.,.F.,(4,3,3,3,3,3,
3,3,3,3,3,3,3,3,3,3,3,3,3,3,3,3,3,3,3,3,3,3,3,3,3,3,3,3,3,3,4),(-0.954382097139102,
-0.915485219868088,-0.876011359398878,-0.858387716138701,-0.851290445572933,
-0.844232875542686,-0.803962784587969,-0.771371663532114,-0.755076103004186,
-0.74670724096049,-0.740703076045499,-0.738780542476259,-0.698754803213944,
-0.658013337818404,-0.616748686984212,-0.590809554692081,-0.56947683727088,
-0.564087732187264,-0.52197879042965,-0.512992157815691,-0.47126838346612,
-0.429066795270051,-0.391147230446158,-0.385001282265118,-0.379585400739026,
-0.33663022313337,-0.293213566977487,-0.277388535974477,-0.234198210308746,
-0.208936638957807,-0.199293375270686,-0.191586968622297,-0.147662130465962,
-0.103303648130549,-0.0589022233416743,-0.0321056395012393,0.),
 .UNSPECIFIED.);
#2888=B_SPLINE_CURVE_WITH_KNOTS('',3,(#35598,#35599,#35600,#35601,#35602,
#35603,#35604,#35605,#35606,#35607,#35608,#35609,#35610,#35611,#35612,#35613,
#35614,#35615,#35616,#35617,#35618,#35619,#35620,#35621,#35622,#35623,#35624,
#35625,#35626,#35627,#35628,#35629,#35630,#35631,#35632,#35633,#35634,#35635,
#35636,#35637,#35638,#35639,#35640,#35641,#35642,#35643,#35644,#35645,#35646,
#35647,#35648,#35649,#35650,#35651,#35652,#35653,#35654,#35655,#35656,#35657,
#35658,#35659,#35660,#35661,#35662,#35663,#35664,#35665,#35666,#35667,#35668,
#35669,#35670,#35671,#35672,#35673,#35674,#35675,#35676,#35677,#35678,#35679,
#35680,#35681,#35682,#35683,#35684,#35685,#35686,#35687,#35688,#35689,#35690,
#35691,#35692,#35693,#35694,#35695,#35696,#35697,#35698,#35699,#35700,#35701,
#35702,#35703,#35704,#35705,#35706,#35707,#35708,#35709),.UNSPECIFIED.,
 .F.,.F.,(4,3,3,3,3,3,3,3,3,3,3,3,3,3,3,3,3,3,3,3,3,3,3,3,3,3,3,3,3,3,3,
3,3,3,3,3,3,4),(-0.950777871811376,-0.906311283561082,-0.86180398566132,
-0.842287018017892,-0.832349797485745,-0.825106830080676,-0.781341119219643,
-0.743504681866769,-0.724586463190332,-0.715675956496024,-0.707599455142323,
-0.705668244513895,-0.662940062790035,-0.619927849095546,-0.577350782543376,
-0.550469628354302,-0.530308762712497,-0.524965684945637,-0.519443984453863,
-0.477671746282991,-0.469826165787081,-0.427882412217812,-0.386078816922957,
-0.350449958940854,-0.344039953632224,-0.338265645217358,-0.297454287905639,
-0.257005929493181,-0.243563384994542,-0.202803272714803,-0.180830798401061,
-0.172157453857976,-0.165074010527136,-0.125309029605361,-0.0856893299734917,
-0.0467731925692476,-0.0270234782048685,0.),.UNSPECIFIED.);
#2889=B_SPLINE_CURVE_WITH_KNOTS('',3,(#35711,#35712,#35713,#35714,#35715,
#35716,#35717,#35718,#35719,#35720,#35721,#35722,#35723,#35724,#35725,#35726,
#35727),.UNSPECIFIED.,.F.,.F.,(4,1,1,1,1,1,1,1,1,1,1,1,1,1,4),(15.707963267949,
15.7708570050318,16.2605962726074,16.750335540183,17.2400748077586,17.7298140753341,
18.2195533429097,18.7092926104853,19.1990318780609,19.6887711456365,20.1785104132121,
20.6682496807877,21.1579889483633,21.6477282159389,21.9911485751285),
 .UNSPECIFIED.);
#2890=B_SPLINE_CURVE_WITH_KNOTS('',3,(#35728,#35729,#35730,#35731,#35732,
#35733,#35734,#35735,#35736,#35737,#35738,#35739,#35740,#35741,#35742,#35743,
#35744),.UNSPECIFIED.,.F.,.F.,(4,1,1,1,1,1,1,1,1,1,1,1,1,1,4),(15.707963267949,
15.8688271292748,16.3585663968504,16.848305664426,17.3380449320016,17.8277841995772,
18.3175234671527,18.8072627347283,19.2970020023039,19.7867412698795,20.2764805374551,
20.7662198050307,21.2559590726063,21.7456983401819,21.9911485751285),
 .UNSPECIFIED.);
#2891=B_SPLINE_CURVE_WITH_KNOTS('',3,(#36001,#36002,#36003,#36004,#36005,
#36006,#36007,#36008,#36009,#36010,#36011,#36012,#36013,#36014,#36015,#36016,
#36017,#36018,#36019,#36020,#36021,#36022,#36023,#36024,#36025,#36026,#36027,
#36028,#36029,#36030,#36031,#36032,#36033,#36034,#36035,#36036,#36037,#36038,
#36039,#36040,#36041,#36042,#36043,#36044,#36045,#36046,#36047,#36048,#36049,
#36050,#36051,#36052,#36053,#36054,#36055,#36056,#36057,#36058,#36059,#36060,
#36061,#36062,#36063,#36064,#36065,#36066,#36067,#36068,#36069,#36070,#36071,
#36072,#36073,#36074,#36075,#36076,#36077,#36078,#36079,#36080,#36081,#36082,
#36083,#36084,#36085,#36086,#36087,#36088,#36089,#36090,#36091,#36092,#36093,
#36094,#36095,#36096,#36097,#36098,#36099,#36100,#36101,#36102,#36103,#36104,
#36105,#36106),.UNSPECIFIED.,.F.,.F.,(4,3,3,3,3,3,3,3,3,3,3,3,3,3,3,3,3,
3,3,3,3,3,3,3,3,3,3,3,3,3,3,3,3,3,3,4),(0.,0.0384977089125158,0.0777077350623172,
0.117481174077728,0.157167741411488,0.165169712071236,0.172509866250956,
0.215216950964984,0.255388062329607,0.296070379047766,0.332110061722789,
0.341131635592327,0.34758681189835,0.389053063764889,0.430985757208201,
0.440229109747859,0.481905267093181,0.506030612217038,0.51916002073821,
0.524507558309914,0.530100422386233,0.57258610074797,0.615488329040074,
0.658430771840619,0.674908028084036,0.705394548776867,0.711667703485966,
0.718009631396055,0.761258294065309,0.800643768955652,0.821412106017802,
0.829287077220563,0.837097365220166,0.881633892178726,0.918800193626682,
0.950777871811493),.UNSPECIFIED.);
#2892=B_SPLINE_CURVE_WITH_KNOTS('',3,(#36107,#36108,#36109,#36110,#36111,
#36112,#36113,#36114,#36115,#36116,#36117,#36118,#36119,#36120,#36121,#36122,
#36123,#36124,#36125,#36126,#36127,#36128,#36129,#36130,#36131,#36132,#36133,
#36134,#36135,#36136,#36137,#36138,#36139,#36140,#36141,#36142,#36143,#36144,
#36145,#36146,#36147,#36148,#36149),.UNSPECIFIED.,.F.,.F.,(4,3,3,3,3,3,
3,3,3,3,3,3,3,3,4),(-10.1382057107015,-9.79478535151183,-9.30504608393623,
-8.81530681636064,-8.32556754878505,-7.83582828120946,-7.34608901363387,
-6.85634974605828,-6.36661047848269,-5.87687121090709,-5.3871319433315,
-4.89739267575591,-4.40765340818032,-3.91791414060473,-3.85502040352192),
 .UNSPECIFIED.);
#2893=B_SPLINE_CURVE_WITH_KNOTS('',3,(#36406,#36407,#36408,#36409,#36410,
#36411,#36412,#36413,#36414,#36415,#36416,#36417,#36418,#36419,#36420,#36421,
#36422,#36423,#36424,#36425,#36426,#36427,#36428,#36429,#36430,#36431,#36432,
#36433,#36434,#36435,#36436,#36437,#36438,#36439,#36440,#36441,#36442,#36443,
#36444,#36445,#36446,#36447,#36448),.UNSPECIFIED.,.F.,.F.,(4,3,3,3,3,3,
3,3,3,3,3,3,3,3,4),(7.59153924858054,7.83582828120946,8.32556754878505,
8.81530681636064,9.30504608393623,9.79478535151182,10.2845246190874,10.774263886663,
11.2640031542386,11.7537424218142,12.2434816893898,12.7332209569654,13.222960224541,
13.7126994921165,13.8747245557601),.UNSPECIFIED.);
#2894=B_SPLINE_CURVE_WITH_KNOTS('',3,(#36449,#36450,#36451,#36452,#36453,
#36454,#36455,#36456,#36457,#36458,#36459,#36460,#36461,#36462,#36463,#36464,
#36465,#36466,#36467,#36468,#36469,#36470,#36471,#36472,#36473,#36474,#36475,
#36476,#36477,#36478,#36479,#36480,#36481,#36482,#36483,#36484,#36485,#36486,
#36487,#36488,#36489,#36490,#36491,#36492,#36493,#36494,#36495,#36496,#36497,
#36498,#36499,#36500,#36501,#36502,#36503,#36504,#36505,#36506,#36507,#36508,
#36509,#36510,#36511,#36512,#36513,#36514,#36515,#36516,#36517,#36518,#36519,
#36520,#36521,#36522,#36523,#36524,#36525,#36526,#36527,#36528,#36529,#36530,
#36531,#36532,#36533,#36534,#36535,#36536,#36537,#36538,#36539,#36540,#36541,
#36542,#36543,#36544,#36545,#36546,#36547,#36548,#36549,#36550,#36551),
 .UNSPECIFIED.,.F.,.F.,(4,3,3,3,3,3,3,3,3,3,3,3,3,3,3,3,3,3,3,3,3,3,3,3,
3,3,3,3,3,3,3,3,3,3,4),(0.,0.0441184545897234,0.0885852303427278,0.132705881239172,
0.176248827766947,0.188641766735101,0.194919743535348,0.201110164739286,
0.246435079457907,0.289836405211179,0.333162204589208,0.37069232129194,
0.380555088969513,0.388891713726302,0.431181300092753,0.473131877202055,
0.483282671400137,0.525568063027558,0.54867105757415,0.563330516703862,
0.568979423171459,0.610227610749445,0.651359426261816,0.691816928157437,
0.710392019400299,0.737503640980283,0.744688179095465,0.751191992318133,
0.79162882737332,0.825542868540032,0.845308948087482,0.852099049520499,
0.89146337026381,0.927284992040167,0.954382097139104),.UNSPECIFIED.);
#2895=B_SPLINE_CURVE_WITH_KNOTS('',3,(#36554,#36555,#36556,#36557,#36558,
#36559,#36560,#36561,#36562,#36563,#36564,#36565,#36566,#36567,#36568,#36569,
#36570,#36571,#36572,#36573,#36574,#36575,#36576,#36577,#36578,#36579,#36580,
#36581,#36582,#36583,#36584,#36585,#36586,#36587,#36588,#36589,#36590,#36591,
#36592,#36593,#36594,#36595,#36596,#36597,#36598,#36599,#36600,#36601,#36602,
#36603,#36604,#36605,#36606,#36607,#36608,#36609,#36610,#36611,#36612,#36613,
#36614,#36615,#36616,#36617,#36618,#36619,#36620,#36621,#36622,#36623,#36624,
#36625,#36626,#36627,#36628,#36629,#36630,#36631,#36632,#36633,#36634,#36635,
#36636,#36637,#36638,#36639,#36640,#36641,#36642,#36643,#36644,#36645,#36646,
#36647,#36648,#36649,#36650,#36651,#36652,#36653,#36654,#36655,#36656,#36657,
#36658,#36659,#36660,#36661,#36662),.UNSPECIFIED.,.F.,.F.,(4,3,3,3,3,3,
3,3,3,3,3,3,3,3,3,3,3,3,3,3,3,3,3,3,3,3,3,3,3,3,3,3,3,3,3,3,4),(-0.954382097139068,
-0.915485230776449,-0.876011377695649,-0.858387741528348,-0.851290401489917,
-0.844232864888672,-0.803962779602644,-0.771371661039454,-0.755076101757858,
-0.746707237711699,-0.740703072512022,-0.738780542476263,-0.698754793624434,
-0.658013320988911,-0.616748667997841,-0.590809540452306,-0.569476809965562,
-0.564087700718665,-0.521978753994884,-0.512992157815699,-0.471268385903021,
-0.429066799073804,-0.391147233298974,-0.385001285630552,-0.379585401384325,
-0.33663022579062,-0.293213570311272,-0.277388535974486,-0.234198210334854,
-0.208936638980652,-0.199293375267056,-0.191586968611106,-0.147662130367022,
-0.103303648093833,-0.058902223280959,-0.0321056395012389,0.),
 .UNSPECIFIED.);
#2896=B_SPLINE_CURVE_WITH_KNOTS('',3,(#36663,#36664,#36665,#36666,#36667,
#36668,#36669,#36670,#36671,#36672,#36673,#36674,#36675,#36676,#36677,#36678,
#36679,#36680,#36681,#36682,#36683,#36684,#36685,#36686,#36687,#36688,#36689,
#36690,#36691,#36692,#36693,#36694,#36695,#36696,#36697,#36698,#36699,#36700,
#36701,#36702,#36703,#36704,#36705,#36706,#36707,#36708,#36709,#36710,#36711,
#36712,#36713,#36714,#36715,#36716,#36717,#36718,#36719,#36720,#36721,#36722,
#36723,#36724,#36725,#36726,#36727,#36728,#36729,#36730,#36731,#36732,#36733,
#36734,#36735,#36736,#36737,#36738,#36739,#36740,#36741,#36742,#36743,#36744,
#36745,#36746,#36747,#36748,#36749,#36750,#36751,#36752,#36753,#36754,#36755,
#36756,#36757,#36758,#36759,#36760,#36761,#36762,#36763,#36764,#36765,#36766,
#36767,#36768,#36769,#36770,#36771,#36772,#36773,#36774),.UNSPECIFIED.,
 .F.,.F.,(4,3,3,3,3,3,3,3,3,3,3,3,3,3,3,3,3,3,3,3,3,3,3,3,3,3,3,3,3,3,3,
3,3,3,3,3,3,4),(-0.950777871811448,-0.906311270744792,-0.861803977893823,
-0.842287011221341,-0.832349777444776,-0.825106814972194,-0.781341114085539,
-0.743504679299753,-0.72458646190686,-0.715675954522707,-0.70759945509899,
-0.705668244513967,-0.662940076465589,-0.619927866635559,-0.577350796294309,
-0.550469638667513,-0.530308770447415,-0.524965697973984,-0.519443987026582,
-0.477671747191907,-0.469826165787123,-0.427882411307492,-0.386078815571722,
-0.350449957927431,-0.344039951609201,-0.338265644735927,-0.297454287004672,
-0.25700592740343,-0.243563384994556,-0.202803273177456,-0.180830798805883,
-0.172157454950964,-0.165074010626906,-0.125309029570385,-0.0856893307960596,
-0.0467731959717267,-0.0270234782048714,0.),.UNSPECIFIED.);
#2897=B_SPLINE_CURVE_WITH_KNOTS('',3,(#36776,#36777,#36778,#36779,#36780,
#36781,#36782,#36783,#36784,#36785,#36786,#36787,#36788,#36789,#36790,#36791,
#36792),.UNSPECIFIED.,.F.,.F.,(4,1,1,1,1,1,1,1,1,1,1,1,1,1,4),(15.707963267949,
15.7708570050318,16.2605962726074,16.750335540183,17.2400748077586,17.7298140753341,
18.2195533429097,18.7092926104853,19.1990318780609,19.6887711456365,20.1785104132121,
20.6682496807877,21.1579889483633,21.6477282159389,21.9911485751285),
 .UNSPECIFIED.);
#2898=B_SPLINE_CURVE_WITH_KNOTS('',3,(#36793,#36794,#36795,#36796,#36797,
#36798,#36799,#36800,#36801,#36802,#36803,#36804,#36805,#36806,#36807,#36808,
#36809),.UNSPECIFIED.,.F.,.F.,(4,1,1,1,1,1,1,1,1,1,1,1,1,1,4),(15.707963267949,
15.8688271292748,16.3585663968504,16.848305664426,17.3380449320016,17.8277841995772,
18.3175234671527,18.8072627347283,19.2970020023039,19.7867412698795,20.2764805374551,
20.7662198050307,21.2559590726063,21.7456983401819,21.9911485751285),
 .UNSPECIFIED.);
#2899=B_SPLINE_CURVE_WITH_KNOTS('',3,(#37066,#37067,#37068,#37069,#37070,
#37071,#37072,#37073,#37074,#37075,#37076,#37077,#37078,#37079,#37080,#37081,
#37082,#37083,#37084,#37085,#37086,#37087,#37088,#37089,#37090,#37091,#37092,
#37093,#37094,#37095,#37096,#37097,#37098,#37099,#37100,#37101,#37102,#37103,
#37104,#37105,#37106,#37107,#37108,#37109,#37110,#37111,#37112,#37113,#37114,
#37115,#37116,#37117,#37118,#37119,#37120,#37121,#37122,#37123,#37124,#37125,
#37126,#37127,#37128,#37129,#37130,#37131,#37132,#37133,#37134,#37135,#37136,
#37137,#37138,#37139,#37140,#37141,#37142,#37143,#37144,#37145,#37146,#37147,
#37148,#37149,#37150,#37151,#37152,#37153,#37154,#37155,#37156,#37157,#37158,
#37159,#37160,#37161,#37162,#37163,#37164,#37165,#37166,#37167,#37168,#37169,
#37170,#37171),.UNSPECIFIED.,.F.,.F.,(4,3,3,3,3,3,3,3,3,3,3,3,3,3,3,3,3,
3,3,3,3,3,3,3,3,3,3,3,3,3,3,3,3,3,3,4),(0.,0.0384977475150248,0.0777078043309608,
0.117481251338807,0.157167811108441,0.165169791324504,0.172509865645824,
0.21521695096498,0.255388037601424,0.296070338910308,0.332110031619694,
0.341131619391498,0.347586807233502,0.389053038740716,0.430985725027015,
0.440229109747851,0.481905272272016,0.506030616748518,0.519160021122491,
0.524507558777488,0.530100422405358,0.572586107541232,0.615488339646026,
0.658430782990829,0.674908028084035,0.705394548776863,0.711667703381707,
0.718009631315357,0.761258293552277,0.800643768570873,0.821412105483859,
0.829287072559959,0.837097364722895,0.881633891927705,0.918800193626661,
0.950777871811476),.UNSPECIFIED.);
#2900=B_SPLINE_CURVE_WITH_KNOTS('',3,(#37172,#37173,#37174,#37175,#37176,
#37177,#37178,#37179,#37180,#37181,#37182,#37183,#37184,#37185,#37186,#37187,
#37188,#37189,#37190,#37191,#37192,#37193,#37194,#37195,#37196,#37197,#37198,
#37199,#37200,#37201,#37202,#37203,#37204,#37205,#37206,#37207,#37208,#37209,
#37210,#37211,#37212,#37213,#37214),.UNSPECIFIED.,.F.,.F.,(4,3,3,3,3,3,
3,3,3,3,3,3,3,3,4),(-10.1382057107015,-9.79478535151183,-9.30504608393623,
-8.81530681636064,-8.32556754878505,-7.83582828120946,-7.34608901363387,
-6.85634974605828,-6.36661047848269,-5.87687121090709,-5.3871319433315,
-4.89739267575591,-4.40765340818032,-3.91791414060473,-3.85502040352192),
 .UNSPECIFIED.);
#2901=B_SPLINE_CURVE_WITH_KNOTS('',3,(#37471,#37472,#37473,#37474,#37475,
#37476,#37477,#37478,#37479,#37480,#37481,#37482,#37483,#37484,#37485,#37486,
#37487,#37488,#37489,#37490,#37491,#37492,#37493,#37494,#37495,#37496,#37497,
#37498,#37499,#37500,#37501,#37502,#37503,#37504,#37505,#37506,#37507,#37508,
#37509,#37510,#37511,#37512,#37513),.UNSPECIFIED.,.F.,.F.,(4,3,3,3,3,3,
3,3,3,3,3,3,3,3,4),(7.59153924858054,7.83582828120946,8.32556754878505,
8.81530681636064,9.30504608393623,9.79478535151182,10.2845246190874,10.774263886663,
11.2640031542386,11.7537424218142,12.2434816893898,12.7332209569654,13.222960224541,
13.7126994921165,13.8747245557601),.UNSPECIFIED.);
#2902=B_SPLINE_CURVE_WITH_KNOTS('',3,(#37514,#37515,#37516,#37517,#37518,
#37519,#37520,#37521,#37522,#37523,#37524,#37525,#37526,#37527,#37528,#37529,
#37530,#37531,#37532,#37533,#37534,#37535,#37536,#37537,#37538,#37539,#37540,
#37541,#37542,#37543,#37544,#37545,#37546,#37547,#37548,#37549,#37550,#37551,
#37552,#37553,#37554,#37555,#37556,#37557,#37558,#37559,#37560,#37561,#37562,
#37563,#37564,#37565,#37566,#37567,#37568,#37569,#37570,#37571,#37572,#37573,
#37574,#37575,#37576,#37577,#37578,#37579,#37580,#37581,#37582,#37583,#37584,
#37585,#37586,#37587,#37588,#37589,#37590,#37591,#37592,#37593,#37594,#37595,
#37596,#37597,#37598,#37599,#37600,#37601,#37602,#37603,#37604,#37605,#37606,
#37607,#37608,#37609,#37610,#37611,#37612,#37613,#37614,#37615,#37616),
 .UNSPECIFIED.,.F.,.F.,(4,3,3,3,3,3,3,3,3,3,3,3,3,3,3,3,3,3,3,3,3,3,3,3,
3,3,3,3,3,3,3,3,3,3,4),(0.,0.0441184469048226,0.0885852208367534,0.132705877001749,
0.176248830667822,0.188641774332082,0.19491905746566,0.201110035903684,
0.246435079457913,0.289836407260929,0.333162206289049,0.370692322566821,
0.380555108078741,0.388891708168043,0.431181294952235,0.473131870976936,
0.483282671400138,0.525568062903358,0.548671057465475,0.563330517012381,
0.568979423553707,0.610227610939762,0.651359426294659,0.691816927448079,
0.710392019400295,0.737503640980278,0.744688179724382,0.751191992440766,
0.79162882740354,0.825542868562695,0.845308948055337,0.852099049553749,
0.891463370783818,0.927284992040159,0.954382097139101),.UNSPECIFIED.);
#2903=B_SPLINE_CURVE_WITH_KNOTS('',3,(#37619,#37620,#37621,#37622,#37623,
#37624,#37625,#37626,#37627,#37628,#37629,#37630,#37631,#37632,#37633,#37634,
#37635,#37636,#37637,#37638,#37639,#37640,#37641,#37642,#37643,#37644,#37645,
#37646,#37647,#37648,#37649,#37650,#37651,#37652,#37653,#37654,#37655,#37656,
#37657,#37658,#37659,#37660,#37661,#37662,#37663,#37664,#37665,#37666,#37667,
#37668,#37669,#37670,#37671,#37672,#37673,#37674,#37675,#37676,#37677,#37678,
#37679,#37680,#37681,#37682,#37683,#37684,#37685,#37686,#37687,#37688,#37689,
#37690,#37691,#37692,#37693,#37694,#37695,#37696,#37697,#37698,#37699,#37700,
#37701,#37702,#37703,#37704,#37705,#37706,#37707,#37708,#37709,#37710,#37711,
#37712,#37713,#37714,#37715,#37716,#37717,#37718,#37719,#37720,#37721,#37722,
#37723,#37724,#37725,#37726,#37727),.UNSPECIFIED.,.F.,.F.,(4,3,3,3,3,3,
3,3,3,3,3,3,3,3,3,3,3,3,3,3,3,3,3,3,3,3,3,3,3,3,3,3,3,3,3,3,4),(-0.954382097138977,
-0.915485207744247,-0.876011339058948,-0.858387687911483,-0.85129049416266,
-0.844232887287554,-0.803962790021771,-0.771371666248987,-0.755076104362594,
-0.74670724449792,-0.74070308011976,-0.738780542476202,-0.698754813889051,
-0.65801335656101,-0.616748708123891,-0.590809570546834,-0.569476867671065,
-0.564087767374825,-0.521978831154271,-0.512992157815662,-0.471268380752573,
-0.429066791033322,-0.391147227268606,-0.385001278360174,-0.379585399990937,
-0.336630220157075,-0.293213563249867,-0.277388535974458,-0.2341982102794,
-0.208936638932129,-0.199293375273106,-0.191586968667389,-0.147662130603415,
-0.103303648196658,-0.05890222343554,-0.0321056395012341,0.),
 .UNSPECIFIED.);
#2904=B_SPLINE_CURVE_WITH_KNOTS('',3,(#37728,#37729,#37730,#37731,#37732,
#37733,#37734,#37735,#37736,#37737,#37738,#37739,#37740,#37741,#37742,#37743,
#37744,#37745,#37746,#37747,#37748,#37749,#37750,#37751,#37752,#37753,#37754,
#37755,#37756,#37757,#37758,#37759,#37760,#37761,#37762,#37763,#37764,#37765,
#37766,#37767,#37768,#37769,#37770,#37771,#37772,#37773,#37774,#37775,#37776,
#37777,#37778,#37779,#37780,#37781,#37782,#37783,#37784,#37785,#37786,#37787,
#37788,#37789,#37790,#37791,#37792,#37793,#37794,#37795,#37796,#37797,#37798,
#37799,#37800,#37801,#37802,#37803,#37804,#37805,#37806,#37807,#37808,#37809,
#37810,#37811,#37812,#37813,#37814,#37815,#37816,#37817,#37818,#37819,#37820,
#37821,#37822,#37823,#37824,#37825,#37826,#37827,#37828,#37829,#37830,#37831,
#37832,#37833,#37834,#37835,#37836,#37837,#37838,#37839),.UNSPECIFIED.,
 .F.,.F.,(4,3,3,3,3,3,3,3,3,3,3,3,3,3,3,3,3,3,3,3,3,3,3,3,3,3,3,3,3,3,3,
3,3,3,3,3,3,4),(-0.950777871811478,-0.906311279635952,-0.861803983277576,
-0.842287015932126,-0.832349791336995,-0.825106825323525,-0.781341117514485,
-0.743504681014231,-0.724586462764104,-0.715675955845772,-0.70759945511304,
-0.705668244513976,-0.662940066976017,-0.619927854462604,-0.577350786751952,
-0.550469631510745,-0.530308765079839,-0.524965688989733,-0.519443985250198,
-0.477671746572218,-0.469826165787122,-0.427882411937048,-0.386078816514926,
-0.350449958634833,-0.344039953072562,-0.338265645084795,-0.297454287641941,
-0.257005928865392,-0.243563384994553,-0.202803272858004,-0.180830798526362,
-0.172157454195869,-0.165074010559054,-0.125309029596673,-0.0856893302259524,
-0.0467731936127253,-0.0270234782048685,0.),.UNSPECIFIED.);
#2905=B_SPLINE_CURVE_WITH_KNOTS('',3,(#37841,#37842,#37843,#37844,#37845,
#37846,#37847,#37848,#37849,#37850,#37851,#37852,#37853,#37854,#37855,#37856,
#37857),.UNSPECIFIED.,.F.,.F.,(4,1,1,1,1,1,1,1,1,1,1,1,1,1,4),(15.707963267949,
15.7708570050318,16.2605962726074,16.750335540183,17.2400748077586,17.7298140753341,
18.2195533429097,18.7092926104853,19.1990318780609,19.6887711456365,20.1785104132121,
20.6682496807877,21.1579889483633,21.6477282159389,21.9911485751285),
 .UNSPECIFIED.);
#2906=B_SPLINE_CURVE_WITH_KNOTS('',3,(#37858,#37859,#37860,#37861,#37862,
#37863,#37864,#37865,#37866,#37867,#37868,#37869,#37870,#37871,#37872,#37873,
#37874),.UNSPECIFIED.,.F.,.F.,(4,1,1,1,1,1,1,1,1,1,1,1,1,1,4),(15.707963267949,
15.8688271292748,16.3585663968504,16.848305664426,17.3380449320016,17.8277841995772,
18.3175234671527,18.8072627347283,19.2970020023039,19.7867412698795,20.2764805374551,
20.7662198050307,21.2559590726063,21.7456983401819,21.9911485751285),
 .UNSPECIFIED.);
#2907=B_SPLINE_CURVE_WITH_KNOTS('',3,(#38131,#38132,#38133,#38134,#38135,
#38136,#38137,#38138,#38139,#38140,#38141,#38142,#38143,#38144,#38145,#38146,
#38147,#38148,#38149,#38150,#38151,#38152,#38153,#38154,#38155,#38156,#38157,
#38158,#38159,#38160,#38161,#38162,#38163,#38164,#38165,#38166,#38167,#38168,
#38169,#38170,#38171,#38172,#38173,#38174,#38175,#38176,#38177,#38178,#38179,
#38180,#38181,#38182,#38183,#38184,#38185,#38186,#38187,#38188,#38189,#38190,
#38191,#38192,#38193,#38194,#38195,#38196,#38197,#38198,#38199,#38200,#38201,
#38202,#38203,#38204,#38205,#38206,#38207,#38208,#38209,#38210,#38211,#38212,
#38213,#38214,#38215,#38216,#38217,#38218,#38219,#38220,#38221,#38222,#38223,
#38224,#38225,#38226,#38227,#38228,#38229,#38230,#38231,#38232,#38233,#38234,
#38235,#38236),.UNSPECIFIED.,.F.,.F.,(4,3,3,3,3,3,3,3,3,3,3,3,3,3,3,3,3,
3,3,3,3,3,3,3,3,3,3,3,3,3,3,3,3,3,3,4),(0.,0.0384977207228922,0.0777077562539873,
0.117481197715763,0.157167762737478,0.165169736321266,0.172509866069542,
0.215216950964976,0.255388054767118,0.29607036677152,0.332110052515598,
0.341131630636987,0.347586810455887,0.389053056094659,0.430985747347695,
0.440229109747833,0.481905268675028,0.50603061360115,0.519160020855356,
0.524507558424947,0.530100422386196,0.572586102817588,0.615488332273333,
0.65843077524041,0.674908028084002,0.705394548776831,0.711667703500688,
0.718009631383646,0.761258293923528,0.800643768849303,0.821412105867649,
0.829287075911994,0.837097365077352,0.88163389211237,0.91880019362663,0.950777871811445),
 .UNSPECIFIED.);
#2908=B_SPLINE_CURVE_WITH_KNOTS('',3,(#38237,#38238,#38239,#38240,#38241,
#38242,#38243,#38244,#38245,#38246,#38247,#38248,#38249,#38250,#38251,#38252,
#38253,#38254,#38255,#38256,#38257,#38258,#38259,#38260,#38261,#38262,#38263,
#38264,#38265,#38266,#38267,#38268,#38269,#38270,#38271,#38272,#38273,#38274,
#38275,#38276,#38277,#38278,#38279),.UNSPECIFIED.,.F.,.F.,(4,3,3,3,3,3,
3,3,3,3,3,3,3,3,4),(-10.1382057107015,-9.79478535151182,-9.30504608393623,
-8.81530681636064,-8.32556754878505,-7.83582828120945,-7.34608901363386,
-6.85634974605827,-6.36661047848268,-5.87687121090709,-5.3871319433315,
-4.89739267575591,-4.40765340818032,-3.91791414060473,-3.85502040352192),
 .UNSPECIFIED.);
#2909=B_SPLINE_CURVE_WITH_KNOTS('',3,(#38536,#38537,#38538,#38539,#38540,
#38541,#38542,#38543,#38544,#38545,#38546,#38547,#38548,#38549,#38550,#38551,
#38552,#38553,#38554,#38555,#38556,#38557,#38558,#38559,#38560,#38561,#38562,
#38563,#38564,#38565,#38566,#38567,#38568,#38569,#38570,#38571,#38572,#38573,
#38574,#38575,#38576,#38577,#38578),.UNSPECIFIED.,.F.,.F.,(4,3,3,3,3,3,
3,3,3,3,3,3,3,3,4),(7.59153924858054,7.83582828120946,8.32556754878505,
8.81530681636064,9.30504608393623,9.79478535151182,10.2845246190874,10.774263886663,
11.2640031542386,11.7537424218142,12.2434816893898,12.7332209569654,13.222960224541,
13.7126994921165,13.8747245557601),.UNSPECIFIED.);
#2910=B_SPLINE_CURVE_WITH_KNOTS('',3,(#38579,#38580,#38581,#38582,#38583,
#38584,#38585,#38586,#38587,#38588,#38589,#38590,#38591,#38592,#38593,#38594,
#38595,#38596,#38597,#38598,#38599,#38600,#38601,#38602,#38603,#38604,#38605,
#38606,#38607,#38608,#38609,#38610,#38611,#38612,#38613,#38614,#38615,#38616,
#38617,#38618,#38619,#38620,#38621,#38622,#38623,#38624,#38625,#38626,#38627,
#38628,#38629,#38630,#38631,#38632,#38633,#38634,#38635,#38636,#38637,#38638,
#38639,#38640,#38641,#38642,#38643,#38644,#38645,#38646,#38647,#38648,#38649,
#38650,#38651,#38652,#38653,#38654,#38655,#38656,#38657,#38658,#38659,#38660,
#38661,#38662,#38663,#38664,#38665,#38666,#38667,#38668,#38669,#38670,#38671,
#38672,#38673,#38674,#38675,#38676,#38677,#38678,#38679,#38680,#38681),
 .UNSPECIFIED.,.F.,.F.,(4,3,3,3,3,3,3,3,3,3,3,3,3,3,3,3,3,3,3,3,3,3,3,3,
3,3,3,3,3,3,3,3,3,3,4),(0.,0.0441184631390831,0.0885852409169272,0.132705885951212,
0.176248824533162,0.188641758266505,0.194920509910256,0.201110308777038,
0.246435079457889,0.289836402930589,0.333162202698913,0.370692319874208,
0.380555067756269,0.388891719911904,0.431181305813495,0.473131884132789,
0.483282671400094,0.525568063164174,0.548671057693681,0.563330516361131,
0.568979422724069,0.610227610515779,0.6513594262039,0.691816928928125,0.710392019400234,
0.737503640980213,0.744688178741843,0.751191992239498,0.791628827388096,
0.825542868551089,0.845308948164629,0.85209904962518,0.891463369824715,
0.927284992040065,0.954382097139),.UNSPECIFIED.);
#2911=B_SPLINE_CURVE_WITH_KNOTS('',3,(#38684,#38685,#38686,#38687,#38688,
#38689,#38690,#38691,#38692,#38693,#38694,#38695,#38696,#38697,#38698,#38699,
#38700,#38701,#38702,#38703,#38704,#38705,#38706,#38707,#38708,#38709,#38710,
#38711,#38712,#38713,#38714,#38715,#38716,#38717,#38718,#38719,#38720,#38721,
#38722,#38723,#38724,#38725,#38726,#38727,#38728,#38729,#38730,#38731,#38732,
#38733,#38734,#38735,#38736,#38737,#38738,#38739,#38740,#38741,#38742,#38743,
#38744,#38745,#38746,#38747,#38748,#38749,#38750,#38751,#38752,#38753,#38754,
#38755,#38756,#38757,#38758,#38759,#38760,#38761,#38762,#38763,#38764,#38765,
#38766,#38767,#38768,#38769,#38770,#38771,#38772,#38773,#38774,#38775,#38776,
#38777,#38778,#38779,#38780,#38781,#38782,#38783,#38784,#38785,#38786,#38787,
#38788,#38789,#38790,#38791,#38792),.UNSPECIFIED.,.F.,.F.,(4,3,3,3,3,3,
3,3,3,3,3,3,3,3,3,3,3,3,3,3,3,3,3,3,3,3,3,3,3,3,3,3,3,3,3,3,4),(-0.954382097139049,
-0.915485243799018,-0.876011399544332,-0.85838777184726,-0.851290348307254,
-0.844232852031221,-0.80396277352234,-0.771371657999283,-0.755076100237755,
-0.746707233752317,-0.740703067945048,-0.738780542476226,-0.698754782173372,
-0.658013300891092,-0.616748645324364,-0.590809523447192,-0.569476777358248,
-0.564087663108025,-0.521978710451211,-0.512992157815676,-0.471268388808549,
-0.429066803611481,-0.391147236702228,-0.385001289855828,-0.379585402193585,
-0.33663022899104,-0.293213574317017,-0.277388535974469,-0.23419821036879,
-0.208936639010346,-0.199293375269724,-0.191586968520703,-0.147662130179972,
-0.1033036479831,-0.0589022231403947,-0.0321056395012349,0.),
 .UNSPECIFIED.);
#2912=B_SPLINE_CURVE_WITH_KNOTS('',3,(#38793,#38794,#38795,#38796,#38797,
#38798,#38799,#38800,#38801,#38802,#38803,#38804,#38805,#38806,#38807,#38808,
#38809,#38810,#38811,#38812,#38813,#38814,#38815,#38816,#38817,#38818,#38819,
#38820,#38821,#38822,#38823,#38824,#38825,#38826,#38827,#38828,#38829,#38830,
#38831,#38832,#38833,#38834,#38835,#38836,#38837,#38838,#38839,#38840,#38841,
#38842,#38843,#38844,#38845,#38846,#38847,#38848,#38849,#38850,#38851,#38852,
#38853,#38854,#38855,#38856,#38857,#38858,#38859,#38860,#38861,#38862,#38863,
#38864,#38865,#38866,#38867,#38868,#38869,#38870,#38871,#38872,#38873,#38874,
#38875,#38876,#38877,#38878,#38879,#38880,#38881,#38882,#38883,#38884,#38885,
#38886,#38887,#38888,#38889,#38890,#38891,#38892,#38893,#38894,#38895,#38896,
#38897,#38898,#38899,#38900,#38901,#38902,#38903,#38904),.UNSPECIFIED.,
 .F.,.F.,(4,3,3,3,3,3,3,3,3,3,3,3,3,3,3,3,3,3,3,3,3,3,3,3,3,3,3,3,3,3,3,
3,3,3,3,3,3,4),(-0.950777871811488,-0.906311274832857,-0.861803980370618,
-0.842287013388538,-0.832349783836988,-0.825106819793286,-0.781341115719767,
-0.743504680116872,-0.724586462315425,-0.715675955150876,-0.707599455145821,
-0.705668244513978,-0.662940072098965,-0.619927861036148,-0.577350791907412,
-0.550469635377338,-0.530308767979781,-0.524965693857714,-0.519443986212373,
-0.477671746910201,-0.469826165787113,-0.427882411597154,-0.386078816010451,
-0.350449958256475,-0.34403995205164,-0.338265644838692,-0.29745428724094,
-0.257005928020942,-0.243563384994547,-0.202803273036419,-0.180830798682476,
-0.172157454615961,-0.165074010553165,-0.125309029539932,-0.0856893304901558,
-0.0467731948431029,-0.0270234782048771,0.),.UNSPECIFIED.);
#2913=B_SPLINE_CURVE_WITH_KNOTS('',3,(#38906,#38907,#38908,#38909,#38910,
#38911,#38912,#38913,#38914,#38915,#38916,#38917,#38918,#38919,#38920,#38921,
#38922),.UNSPECIFIED.,.F.,.F.,(4,1,1,1,1,1,1,1,1,1,1,1,1,1,4),(15.707963267949,
15.7708570050318,16.2605962726074,16.750335540183,17.2400748077586,17.7298140753341,
18.2195533429097,18.7092926104853,19.1990318780609,19.6887711456365,20.1785104132121,
20.6682496807877,21.1579889483633,21.6477282159389,21.9911485751285),
 .UNSPECIFIED.);
#2914=B_SPLINE_CURVE_WITH_KNOTS('',3,(#38923,#38924,#38925,#38926,#38927,
#38928,#38929,#38930,#38931,#38932,#38933,#38934,#38935,#38936,#38937,#38938,
#38939),.UNSPECIFIED.,.F.,.F.,(4,1,1,1,1,1,1,1,1,1,1,1,1,1,4),(15.707963267949,
15.8688271292748,16.3585663968504,16.848305664426,17.3380449320016,17.8277841995772,
18.3175234671527,18.8072627347283,19.2970020023039,19.7867412698795,20.2764805374551,
20.7662198050307,21.2559590726063,21.7456983401819,21.9911485751285),
 .UNSPECIFIED.);
#2915=B_SPLINE_CURVE_WITH_KNOTS('',3,(#39196,#39197,#39198,#39199,#39200,
#39201,#39202,#39203,#39204,#39205,#39206,#39207,#39208,#39209,#39210,#39211,
#39212,#39213,#39214,#39215,#39216,#39217,#39218,#39219,#39220,#39221,#39222,
#39223,#39224,#39225,#39226,#39227,#39228,#39229,#39230,#39231,#39232,#39233,
#39234,#39235,#39236,#39237,#39238,#39239,#39240,#39241,#39242,#39243,#39244,
#39245,#39246,#39247,#39248,#39249,#39250,#39251,#39252,#39253,#39254,#39255,
#39256,#39257,#39258,#39259,#39260,#39261,#39262,#39263,#39264,#39265,#39266,
#39267,#39268,#39269,#39270,#39271,#39272,#39273,#39274,#39275,#39276,#39277,
#39278,#39279,#39280,#39281,#39282,#39283,#39284,#39285,#39286,#39287,#39288,
#39289,#39290,#39291,#39292,#39293,#39294,#39295,#39296,#39297,#39298,#39299,
#39300,#39301),.UNSPECIFIED.,.F.,.F.,(4,3,3,3,3,3,3,3,3,3,3,3,3,3,3,3,3,
3,3,3,3,3,3,3,3,3,3,3,3,3,3,3,3,3,3,4),(0.,0.0384977351933318,0.0777077822193152,
0.117481226676887,0.157167788863923,0.165169766029963,0.17250986583581,
0.215216950964983,0.255388045498387,0.296070351727255,0.332110041232406,
0.341131624564715,0.347586808736851,0.389053046746773,0.430985735316375,
0.440229109747859,0.481905270616845,0.506030615300244,0.519160020999484,
0.524507558604161,0.53010042239424,0.572586105363907,0.61548833624855,0.658430779419949,
0.674908028084036,0.705394548776866,0.711667703489009,0.718009631360576,
0.761258293736136,0.80064376870877,0.821412105671848,0.829287074196938,
0.837097364893477,0.881633892019366,0.918800193626673,0.950777871811486),
 .UNSPECIFIED.);
#2916=B_SPLINE_CURVE_WITH_KNOTS('',3,(#39302,#39303,#39304,#39305,#39306,
#39307,#39308,#39309,#39310,#39311,#39312,#39313,#39314,#39315,#39316,#39317,
#39318,#39319,#39320,#39321,#39322,#39323,#39324,#39325,#39326,#39327,#39328,
#39329,#39330,#39331,#39332,#39333,#39334,#39335,#39336,#39337,#39338,#39339,
#39340,#39341,#39342,#39343,#39344),.UNSPECIFIED.,.F.,.F.,(4,3,3,3,3,3,
3,3,3,3,3,3,3,3,4),(-10.1382057107015,-9.79478535151183,-9.30504608393623,
-8.81530681636065,-8.32556754878505,-7.83582828120946,-7.34608901363387,
-6.85634974605828,-6.36661047848269,-5.8768712109071,-5.3871319433315,-4.89739267575591,
-4.40765340818032,-3.91791414060473,-3.85502040352192),.UNSPECIFIED.);
#2917=B_SPLINE_CURVE_WITH_KNOTS('',3,(#39601,#39602,#39603,#39604,#39605,
#39606,#39607,#39608,#39609,#39610,#39611,#39612,#39613,#39614,#39615,#39616,
#39617,#39618,#39619,#39620,#39621,#39622,#39623,#39624,#39625,#39626,#39627,
#39628,#39629,#39630,#39631,#39632,#39633,#39634,#39635,#39636,#39637,#39638,
#39639,#39640,#39641,#39642,#39643),.UNSPECIFIED.,.F.,.F.,(4,3,3,3,3,3,
3,3,3,3,3,3,3,3,4),(7.59153924858054,7.83582828120945,8.32556754878505,
8.81530681636064,9.30504608393623,9.79478535151182,10.2845246190874,10.774263886663,
11.2640031542386,11.7537424218142,12.2434816893898,12.7332209569654,13.222960224541,
13.7126994921165,13.8747245557601),.UNSPECIFIED.);
#2918=B_SPLINE_CURVE_WITH_KNOTS('',3,(#39644,#39645,#39646,#39647,#39648,
#39649,#39650,#39651,#39652,#39653,#39654,#39655,#39656,#39657,#39658,#39659,
#39660,#39661,#39662,#39663,#39664,#39665,#39666,#39667,#39668,#39669,#39670,
#39671,#39672,#39673,#39674,#39675,#39676,#39677,#39678,#39679,#39680,#39681,
#39682,#39683,#39684,#39685,#39686,#39687,#39688,#39689,#39690,#39691,#39692,
#39693,#39694,#39695,#39696,#39697,#39698,#39699,#39700,#39701,#39702,#39703,
#39704,#39705,#39706,#39707,#39708,#39709,#39710,#39711,#39712,#39713,#39714,
#39715,#39716,#39717,#39718,#39719,#39720,#39721,#39722,#39723,#39724,#39725,
#39726,#39727,#39728,#39729,#39730,#39731,#39732,#39733,#39734,#39735,#39736,
#39737,#39738,#39739,#39740,#39741,#39742,#39743,#39744,#39745,#39746),
 .UNSPECIFIED.,.F.,.F.,(4,3,3,3,3,3,3,3,3,3,3,3,3,3,3,3,3,3,3,3,3,3,3,3,
3,3,3,3,3,3,3,3,3,3,4),(0.,0.0441184377234137,0.0885852094785448,0.132705871934227,
0.176248834126375,0.18864178338789,0.19491823898691,0.201109882338307,0.246435079457898,
0.289836409708683,0.333162208320045,0.370692324090062,0.380555130854219,
0.38889170154541,0.431181288829226,0.473131863558235,0.483282671400115,
0.525568062754779,0.548671057335465,0.56333051737996,0.568979423977601,
0.610227611133655,0.651359426299229,0.691816926566307,0.710392019400264,
0.737503640980246,0.744688180059427,0.751191992518895,0.791628827376913,
0.825542868542715,0.845308947964658,0.852099049499542,0.891463371311063,
0.92728499204012,0.954382097139051),.UNSPECIFIED.);
#2919=B_SPLINE_CURVE_WITH_KNOTS('',3,(#39753,#39754,#39755,#39756,#39757,
#39758,#39759,#39760,#39761,#39762,#39763,#39764,#39765,#39766,#39767,#39768,
#39769,#39770,#39771,#39772,#39773,#39774,#39775,#39776,#39777,#39778,#39779,
#39780,#39781,#39782,#39783,#39784,#39785,#39786,#39787,#39788,#39789,#39790,
#39791,#39792,#39793,#39794,#39795,#39796,#39797,#39798,#39799,#39800,#39801,
#39802,#39803,#39804,#39805,#39806,#39807,#39808,#39809,#39810,#39811,#39812,
#39813,#39814,#39815,#39816,#39817,#39818,#39819,#39820,#39821,#39822,#39823,
#39824,#39825,#39826,#39827,#39828,#39829,#39830,#39831,#39832,#39833,#39834,
#39835,#39836,#39837,#39838,#39839,#39840,#39841,#39842,#39843,#39844,#39845,
#39846,#39847,#39848,#39849,#39850,#39851,#39852),.UNSPECIFIED.,.F.,.F.,
(4,3,3,3,3,3,3,3,3,3,3,3,3,3,3,3,3,3,3,3,3,3,3,3,3,3,3,3,3,3,3,3,3,4),(-0.760759816994569,
-0.72862787829937,-0.695756720514147,-0.68606839026359,-0.679579333012852,
-0.673178904811534,-0.639342185929258,-0.610292612829778,-0.600454920433494,
-0.594751295643759,-0.5602179171347,-0.525201053232817,-0.490288939350313,
-0.469453104796089,-0.455093610752485,-0.450652652628591,-0.414664231423942,
-0.406945601133418,-0.372348152705916,-0.337004174076161,-0.31718673063397,
-0.308923304598713,-0.304448472040256,-0.268404613806068,-0.231699686844986,
-0.194697269281947,-0.172850745496843,-0.161340406317873,-0.156038360829996,
-0.118189716276133,-0.0802678600345118,-0.0429993716816808,-0.0199250790011154,
0.),.UNSPECIFIED.);
#2920=B_SPLINE_CURVE_WITH_KNOTS('',3,(#39853,#39854,#39855,#39856,#39857,
#39858,#39859,#39860,#39861,#39862,#39863,#39864,#39865,#39866,#39867,#39868,
#39869,#39870,#39871,#39872,#39873,#39874,#39875,#39876,#39877,#39878,#39879,
#39880,#39881,#39882,#39883,#39884,#39885,#39886,#39887,#39888,#39889,#39890,
#39891,#39892,#39893,#39894,#39895,#39896,#39897,#39898,#39899,#39900,#39901,
#39902,#39903,#39904,#39905,#39906,#39907,#39908,#39909,#39910,#39911,#39912,
#39913,#39914,#39915,#39916,#39917,#39918,#39919,#39920,#39921,#39922,#39923,
#39924,#39925,#39926,#39927,#39928,#39929,#39930,#39931,#39932,#39933,#39934,
#39935,#39936,#39937,#39938,#39939,#39940,#39941,#39942,#39943,#39944,#39945,
#39946,#39947,#39948,#39949,#39950,#39951,#39952),.UNSPECIFIED.,.F.,.F.,
(4,3,3,3,3,3,3,3,3,3,3,3,3,3,3,3,3,3,3,3,3,3,3,3,3,3,3,3,3,3,3,3,3,4),(-0.757763664684572,
-0.720377639686879,-0.68246665016733,-0.666432992745214,-0.657234612624417,
-0.619826663102441,-0.588739338539928,-0.575138634043828,-0.567711759329971,
-0.562381430293886,-0.525809998287688,-0.489512576741164,-0.454189714609801,
-0.433424302607935,-0.418943938986772,-0.414278003736301,-0.379386458468707,
-0.371128066602335,-0.335727258188192,-0.300034647812248,-0.282321970831172,
-0.275156765762531,-0.270309060105739,-0.23559711240685,-0.200919055510916,
-0.166729845604536,-0.147967591918348,-0.137478179675258,-0.130951779287757,
-0.0975592011702397,-0.0646630819112997,-0.0327161480307065,-0.0166318161150331,
0.),.UNSPECIFIED.);
#2921=B_SPLINE_CURVE_WITH_KNOTS('',3,(#39954,#39955,#39956,#39957,#39958,
#39959,#39960,#39961,#39962,#39963,#39964),.UNSPECIFIED.,.F.,.F.,(4,1,1,
1,1,1,1,1,4),(15.7079632679489,15.7955882081887,16.7801008045318,17.7646134008748,
18.7491259972179,19.733638593561,20.718151189904,21.7026637862471,21.9911485751285),
 .UNSPECIFIED.);
#2922=B_SPLINE_CURVE_WITH_KNOTS('',3,(#39965,#39966,#39967,#39968,#39969,
#39970,#39971,#39972,#39973,#39974),.UNSPECIFIED.,.F.,.F.,(4,1,1,1,1,1,
1,4),(15.7079632679489,16.3681508394037,17.3526634357467,18.3371760320898,
19.3216886284329,20.3062012247759,21.290713821119,21.9911485751285),
 .UNSPECIFIED.);
#2923=B_SPLINE_CURVE_WITH_KNOTS('',3,(#40179,#40180,#40181,#40182,#40183,
#40184,#40185,#40186,#40187,#40188,#40189,#40190,#40191,#40192,#40193,#40194,
#40195,#40196,#40197,#40198,#40199,#40200,#40201,#40202,#40203,#40204,#40205,
#40206,#40207,#40208,#40209,#40210,#40211,#40212,#40213,#40214,#40215,#40216,
#40217,#40218,#40219,#40220,#40221,#40222,#40223,#40224,#40225,#40226,#40227,
#40228,#40229,#40230,#40231,#40232,#40233,#40234,#40235,#40236,#40237,#40238,
#40239,#40240,#40241,#40242,#40243,#40244,#40245,#40246,#40247,#40248,#40249,
#40250,#40251,#40252,#40253,#40254,#40255,#40256,#40257,#40258,#40259,#40260,
#40261,#40262,#40263,#40264,#40265,#40266,#40267,#40268,#40269,#40270,#40271,
#40272),.UNSPECIFIED.,.F.,.F.,(4,3,3,3,3,3,3,3,3,3,3,3,3,3,3,3,3,3,3,3,
3,3,3,3,3,3,3,3,3,3,3,4),(0.,0.0317393131722086,0.0642710888601908,0.0974907644309431,
0.129407607237421,0.134009844296982,0.138840357948445,0.172956104929503,
0.207581737824153,0.243892680088807,0.271125886787297,0.277136007979861,
0.312751955574691,0.348252906207798,0.352825506882768,0.387546385450957,
0.409444611894283,0.417180287420671,0.422139708315971,0.457113923397589,
0.493313993607226,0.529906408582694,0.555907858577878,0.563763193650837,
0.571495314967843,0.608811788498078,0.641088343509601,0.655846955831368,
0.662600714484889,0.700434562175506,0.73791800854417,0.757763664684532),
 .UNSPECIFIED.);
#2924=B_SPLINE_CURVE_WITH_KNOTS('',3,(#40273,#40274,#40275,#40276,#40277,
#40278,#40279,#40280,#40281,#40282,#40283,#40284,#40285,#40286,#40287,#40288,
#40289,#40290,#40291,#40292,#40293,#40294,#40295,#40296,#40297),
 .UNSPECIFIED.,.F.,.F.,(4,3,3,3,3,3,3,3,4),(-10.1336107523121,-9.84512596343066,
-8.86061336708759,-7.87610077074453,-6.89158817440146,-5.9070755780584,
-4.92256298171533,-3.93805038537226,-3.85042544513252),.UNSPECIFIED.);
#2925=B_SPLINE_CURVE_WITH_KNOTS('',3,(#40502,#40503,#40504,#40505,#40506,
#40507,#40508,#40509,#40510,#40511,#40512,#40513,#40514,#40515,#40516,#40517,
#40518,#40519,#40520,#40521,#40522,#40523,#40524,#40525,#40526),
 .UNSPECIFIED.,.F.,.F.,(4,3,3,3,3,3,3,3,4),(7.59202292841098,7.87610077074452,
8.86061336708759,9.84512596343066,10.8296385597737,11.8141511561168,12.7986637524599,
13.7831763488029,13.8752082355906),.UNSPECIFIED.);
#2926=B_SPLINE_CURVE_WITH_KNOTS('',3,(#40527,#40528,#40529,#40530,#40531,
#40532,#40533,#40534,#40535,#40536,#40537,#40538,#40539,#40540,#40541,#40542,
#40543,#40544,#40545,#40546,#40547,#40548,#40549,#40550,#40551,#40552,#40553,
#40554,#40555,#40556,#40557,#40558,#40559,#40560,#40561,#40562,#40563,#40564,
#40565,#40566,#40567,#40568,#40569,#40570,#40571,#40572,#40573,#40574,#40575,
#40576,#40577,#40578,#40579,#40580,#40581,#40582,#40583,#40584,#40585,#40586,
#40587,#40588,#40589,#40590,#40591,#40592,#40593,#40594,#40595,#40596,#40597,
#40598,#40599,#40600,#40601,#40602,#40603,#40604,#40605,#40606,#40607,#40608,
#40609,#40610,#40611,#40612,#40613,#40614,#40615,#40616,#40617,#40618,#40619,
#40620,#40621,#40622,#40623),.UNSPECIFIED.,.F.,.F.,(4,3,3,3,3,3,3,3,3,3,
3,3,3,3,3,3,3,3,3,3,3,3,3,3,3,3,3,3,3,3,3,3,4),(0.,0.0368231104917497,0.0744313668444073,
0.113698757913489,0.148057725098936,0.154809695453249,0.159905279610154,
0.196856237502933,0.233660813338438,0.269922734929624,0.299584675046484,
0.306586456956745,0.311530200028528,0.347067656739102,0.381889315190812,
0.388570495397064,0.424561732072777,0.444531524904213,0.452400918448495,
0.457441217514027,0.493270867496743,0.528364028122716,0.56305045338481,
0.585678948883678,0.594960281935166,0.600628204014577,0.634676029427075,
0.662026626414246,0.675581363680469,0.683279768149963,0.715772844080334,
0.744078417375757,0.760759816994505),.UNSPECIFIED.);
#2927=B_SPLINE_CURVE_WITH_KNOTS('',3,(#40626,#40627,#40628,#40629,#40630,
#40631,#40632,#40633,#40634,#40635,#40636,#40637,#40638,#40639,#40640,#40641,
#40642,#40643,#40644,#40645,#40646,#40647,#40648,#40649,#40650,#40651,#40652,
#40653,#40654,#40655,#40656,#40657,#40658,#40659,#40660,#40661,#40662,#40663,
#40664,#40665,#40666,#40667,#40668,#40669,#40670,#40671,#40672,#40673,#40674,
#40675,#40676,#40677,#40678,#40679,#40680,#40681,#40682,#40683,#40684,#40685,
#40686,#40687,#40688,#40689,#40690,#40691,#40692,#40693,#40694,#40695,#40696,
#40697,#40698,#40699,#40700,#40701,#40702,#40703,#40704,#40705,#40706,#40707,
#40708,#40709,#40710,#40711,#40712,#40713,#40714,#40715,#40716,#40717,#40718,
#40719,#40720,#40721,#40722,#40723,#40724,#40725),.UNSPECIFIED.,.F.,.F.,
(4,3,3,3,3,3,3,3,3,3,3,3,3,3,3,3,3,3,3,3,3,3,3,3,3,3,3,3,3,3,3,3,3,4),(-0.760759816994564,
-0.72862788991672,-0.69575674190594,-0.686068386386768,-0.679579306421937,
-0.673178902123493,-0.639342190945096,-0.610292617218635,-0.600454931774126,
-0.594751307989734,-0.560217937481691,-0.525201077134436,-0.490288959777163,
-0.469453120116225,-0.455093617098093,-0.450652664319302,-0.414664242634724,
-0.40694560113341,-0.372348145271188,-0.337004161764575,-0.317186719091858,
-0.308923268328764,-0.304448416954742,-0.268404551836861,-0.231699621164082,
-0.194697202953257,-0.172850687459238,-0.161340379081848,-0.156038350660818,
-0.118189704854676,-0.080267848749223,-0.0429993598106653,-0.0199250790011036,
0.),.UNSPECIFIED.);
#2928=B_SPLINE_CURVE_WITH_KNOTS('',3,(#40726,#40727,#40728,#40729,#40730,
#40731,#40732,#40733,#40734,#40735,#40736,#40737,#40738,#40739,#40740,#40741,
#40742,#40743,#40744,#40745,#40746,#40747,#40748,#40749,#40750,#40751,#40752,
#40753,#40754,#40755,#40756,#40757,#40758,#40759,#40760,#40761,#40762,#40763,
#40764,#40765,#40766,#40767,#40768,#40769,#40770,#40771,#40772,#40773,#40774,
#40775,#40776,#40777,#40778,#40779,#40780,#40781,#40782,#40783,#40784,#40785,
#40786,#40787,#40788,#40789,#40790,#40791,#40792,#40793,#40794,#40795,#40796,
#40797,#40798,#40799,#40800,#40801,#40802,#40803,#40804,#40805,#40806,#40807,
#40808,#40809,#40810,#40811,#40812,#40813,#40814,#40815,#40816,#40817,#40818,
#40819,#40820,#40821,#40822,#40823,#40824,#40825),.UNSPECIFIED.,.F.,.F.,
(4,3,3,3,3,3,3,3,3,3,3,3,3,3,3,3,3,3,3,3,3,3,3,3,3,3,3,3,3,3,3,3,3,4),(-0.757763664684492,
-0.720377623574381,-0.682466628623801,-0.66643289277039,-0.657234612451942,
-0.619826662873363,-0.588739338339482,-0.575138633855909,-0.567711744977049,
-0.562381426500434,-0.525809996194753,-0.489512580893587,-0.454189724729181,
-0.433424310197464,-0.418943937897784,-0.414278001003576,-0.379386462480084,
-0.371128066602314,-0.335727259413989,-0.300034648045544,-0.282321971049887,
-0.275156772069666,-0.270309064544493,-0.235597116037967,-0.200919059265354,
-0.166729853637965,-0.147967598947598,-0.137478187843834,-0.130951779920804,
-0.0975592047704314,-0.0646630925664832,-0.032716171474427,-0.0166318161150306,
0.),.UNSPECIFIED.);
#2929=B_SPLINE_CURVE_WITH_KNOTS('',3,(#40827,#40828,#40829,#40830,#40831,
#40832,#40833,#40834,#40835,#40836,#40837),.UNSPECIFIED.,.F.,.F.,(4,1,1,
1,1,1,1,1,4),(15.7079632679489,15.7955882081887,16.7801008045318,17.7646134008748,
18.7491259972179,19.733638593561,20.718151189904,21.7026637862471,21.9911485751285),
 .UNSPECIFIED.);
#2930=B_SPLINE_CURVE_WITH_KNOTS('',3,(#40838,#40839,#40840,#40841,#40842,
#40843,#40844,#40845,#40846,#40847),.UNSPECIFIED.,.F.,.F.,(4,1,1,1,1,1,
1,4),(15.7079632679489,16.3681508394037,17.3526634357467,18.3371760320898,
19.3216886284329,20.3062012247759,21.290713821119,21.9911485751285),
 .UNSPECIFIED.);
#2931=B_SPLINE_CURVE_WITH_KNOTS('',3,(#41052,#41053,#41054,#41055,#41056,
#41057,#41058,#41059,#41060,#41061,#41062,#41063,#41064,#41065,#41066,#41067,
#41068,#41069,#41070,#41071,#41072,#41073,#41074,#41075,#41076,#41077,#41078,
#41079,#41080,#41081,#41082,#41083,#41084,#41085,#41086,#41087,#41088,#41089,
#41090,#41091,#41092,#41093,#41094,#41095,#41096,#41097,#41098,#41099,#41100,
#41101,#41102,#41103,#41104,#41105,#41106,#41107,#41108,#41109,#41110,#41111,
#41112,#41113,#41114,#41115,#41116,#41117,#41118,#41119,#41120,#41121,#41122,
#41123,#41124,#41125,#41126,#41127,#41128,#41129,#41130,#41131,#41132,#41133,
#41134,#41135,#41136,#41137,#41138,#41139,#41140,#41141,#41142,#41143,#41144,
#41145),.UNSPECIFIED.,.F.,.F.,(4,3,3,3,3,3,3,3,3,3,3,3,3,3,3,3,3,3,3,3,
3,3,3,3,3,3,3,3,3,3,3,4),(0.,0.0317393385474546,0.0642711372305777,0.0974908302253786,
0.129407664807553,0.134009929659094,0.138840372798717,0.172956137150136,
0.207581778796227,0.243892710817864,0.271125909834093,0.277136017604199,
0.312751969178281,0.34825291267891,0.352825506882778,0.387546373463078,
0.409444600655646,0.417180277227003,0.422139689655615,0.457113887842331,
0.493313950003616,0.529906362555575,0.555907818304148,0.563762874105919,
0.571495346164915,0.60881181674222,0.641088364692705,0.655846960756109,
0.662600717097456,0.700434565111295,0.73791800854416,0.757763664684518),
 .UNSPECIFIED.);
#2932=B_SPLINE_CURVE_WITH_KNOTS('',3,(#41146,#41147,#41148,#41149,#41150,
#41151,#41152,#41153,#41154,#41155,#41156,#41157,#41158,#41159,#41160,#41161,
#41162,#41163,#41164,#41165,#41166,#41167,#41168,#41169,#41170),
 .UNSPECIFIED.,.F.,.F.,(4,3,3,3,3,3,3,3,4),(-10.1336107523121,-9.84512596343066,
-8.86061336708759,-7.87610077074453,-6.89158817440146,-5.9070755780584,
-4.92256298171533,-3.93805038537226,-3.85042544513253),.UNSPECIFIED.);
#2933=B_SPLINE_CURVE_WITH_KNOTS('',3,(#41375,#41376,#41377,#41378,#41379,
#41380,#41381,#41382,#41383,#41384,#41385,#41386,#41387,#41388,#41389,#41390,
#41391,#41392,#41393,#41394,#41395,#41396,#41397,#41398,#41399),
 .UNSPECIFIED.,.F.,.F.,(4,3,3,3,3,3,3,3,4),(7.592022928411,7.87610077074453,
8.8606133670876,9.84512596343066,10.8296385597737,11.8141511561168,12.7986637524599,
13.7831763488029,13.8752082355906),.UNSPECIFIED.);
#2934=B_SPLINE_CURVE_WITH_KNOTS('',3,(#41400,#41401,#41402,#41403,#41404,
#41405,#41406,#41407,#41408,#41409,#41410,#41411,#41412,#41413,#41414,#41415,
#41416,#41417,#41418,#41419,#41420,#41421,#41422,#41423,#41424,#41425,#41426,
#41427,#41428,#41429,#41430,#41431,#41432,#41433,#41434,#41435,#41436,#41437,
#41438,#41439,#41440,#41441,#41442,#41443,#41444,#41445,#41446,#41447,#41448,
#41449,#41450,#41451,#41452,#41453,#41454,#41455,#41456,#41457,#41458,#41459,
#41460,#41461,#41462,#41463,#41464,#41465,#41466,#41467,#41468,#41469,#41470,
#41471,#41472,#41473,#41474,#41475,#41476,#41477,#41478,#41479,#41480,#41481,
#41482,#41483,#41484,#41485,#41486,#41487,#41488,#41489,#41490,#41491,#41492,
#41493,#41494,#41495,#41496),.UNSPECIFIED.,.F.,.F.,(4,3,3,3,3,3,3,3,3,3,
3,3,3,3,3,3,3,3,3,3,3,3,3,3,3,3,3,3,3,3,3,3,4),(0.,0.0368231001962915,0.0744313508791827,
0.113698743943915,0.148057712875556,0.154809587820709,0.159905235470134,
0.196856192833996,0.233660771612868,0.269922697362649,0.299584646871248,
0.306586382979425,0.31153012555125,0.347067586247613,0.38188924839607,0.388570495397043,
0.424561731743958,0.444531524595945,0.452400916951006,0.457441217399145,
0.493270867396221,0.52836402777598,0.563050454529762,0.58567894988551,0.594960252908482,
0.600628199835682,0.634676026456314,0.662026624186173,0.675581364411591,
0.683279768872821,0.71577284943675,0.744078417375749,0.7607598169945),
 .UNSPECIFIED.);
#2935=B_SPLINE_CURVE_WITH_KNOTS('',3,(#41499,#41500,#41501,#41502,#41503,
#41504,#41505,#41506,#41507,#41508,#41509,#41510,#41511,#41512,#41513,#41514,
#41515,#41516,#41517,#41518,#41519,#41520,#41521,#41522,#41523,#41524,#41525,
#41526,#41527,#41528,#41529,#41530,#41531,#41532,#41533,#41534,#41535,#41536,
#41537,#41538,#41539,#41540,#41541,#41542,#41543,#41544,#41545,#41546,#41547,
#41548,#41549,#41550,#41551,#41552,#41553,#41554,#41555,#41556,#41557,#41558,
#41559,#41560,#41561,#41562,#41563,#41564,#41565,#41566,#41567,#41568,#41569,
#41570,#41571,#41572,#41573,#41574,#41575,#41576,#41577,#41578,#41579,#41580,
#41581,#41582,#41583,#41584,#41585,#41586,#41587,#41588,#41589,#41590,#41591,
#41592,#41593,#41594,#41595,#41596,#41597,#41598),.UNSPECIFIED.,.F.,.F.,
(4,3,3,3,3,3,3,3,3,3,3,3,3,3,3,3,3,3,3,3,3,3,3,3,3,3,3,3,3,3,3,3,3,4),(-0.760759816994606,
-0.728627835147078,-0.695756641029334,-0.686068404654108,-0.679579431591451,
-0.673178914772871,-0.639342167265441,-0.610292596498939,-0.600454878237806,
-0.594751249714991,-0.560217841490549,-0.525200964388687,-0.490288863419066,
-0.469453047847656,-0.455093587171559,-0.450652608595185,-0.414664189190038,
-0.406945601133428,-0.372348180330614,-0.337004219823422,-0.317186773522027,
-0.30892343932953,-0.304448676715557,-0.268404844057691,-0.231699930890561,
-0.194697515735063,-0.172850961143318,-0.161340507514556,-0.156038398693486,
-0.118189758791589,-0.0802679020340656,-0.0429994158654706,-0.0199250790011039,
0.),.UNSPECIFIED.);
#2936=B_SPLINE_CURVE_WITH_KNOTS('',3,(#41599,#41600,#41601,#41602,#41603,
#41604,#41605,#41606,#41607,#41608,#41609,#41610,#41611,#41612,#41613,#41614,
#41615,#41616,#41617,#41618,#41619,#41620,#41621,#41622,#41623,#41624,#41625,
#41626,#41627,#41628,#41629,#41630,#41631,#41632,#41633,#41634,#41635,#41636,
#41637,#41638,#41639,#41640,#41641,#41642,#41643,#41644,#41645,#41646,#41647,
#41648,#41649,#41650,#41651,#41652,#41653,#41654,#41655,#41656,#41657,#41658,
#41659,#41660,#41661,#41662,#41663,#41664,#41665,#41666,#41667,#41668,#41669,
#41670,#41671,#41672,#41673,#41674,#41675,#41676,#41677,#41678,#41679,#41680,
#41681,#41682,#41683,#41684,#41685,#41686,#41687,#41688,#41689,#41690,#41691,
#41692,#41693,#41694,#41695,#41696,#41697,#41698),.UNSPECIFIED.,.F.,.F.,
(4,3,3,3,3,3,3,3,3,3,3,3,3,3,3,3,3,3,3,3,3,3,3,3,3,3,3,3,3,3,3,3,3,4),(-0.75776366468449,
-0.720377652726986,-0.682466667598983,-0.666433073646011,-0.657234612750941,
-0.619826663274133,-0.588739338690156,-0.575138634184666,-0.567711770657871,
-0.562381433308457,-0.525809999923709,-0.489512573327164,-0.454189706368117,
-0.433424296426666,-0.418943939880433,-0.414278005844695,-0.379386455118474,
-0.371128066602313,-0.33572725719849,-0.300034647625018,-0.282321970655644,
-0.275156760805834,-0.270309056596631,-0.235597109555266,-0.200919052556176,
-0.166729839187693,-0.147967586303611,-0.137478173109318,-0.130951778681891,
-0.0975591981658623,-0.0646630732109414,-0.0327161289923639,-0.0166318161150331,
0.),.UNSPECIFIED.);
#2937=B_SPLINE_CURVE_WITH_KNOTS('',3,(#41700,#41701,#41702,#41703,#41704,
#41705,#41706,#41707,#41708,#41709,#41710),.UNSPECIFIED.,.F.,.F.,(4,1,1,
1,1,1,1,1,4),(15.7079632679489,15.7955882081887,16.7801008045318,17.7646134008748,
18.7491259972179,19.733638593561,20.718151189904,21.7026637862471,21.9911485751285),
 .UNSPECIFIED.);
#2938=B_SPLINE_CURVE_WITH_KNOTS('',3,(#41711,#41712,#41713,#41714,#41715,
#41716,#41717,#41718,#41719,#41720),.UNSPECIFIED.,.F.,.F.,(4,1,1,1,1,1,
1,4),(15.7079632679489,16.3681508394037,17.3526634357467,18.3371760320898,
19.3216886284329,20.3062012247759,21.290713821119,21.9911485751285),
 .UNSPECIFIED.);
#2939=B_SPLINE_CURVE_WITH_KNOTS('',3,(#41925,#41926,#41927,#41928,#41929,
#41930,#41931,#41932,#41933,#41934,#41935,#41936,#41937,#41938,#41939,#41940,
#41941,#41942,#41943,#41944,#41945,#41946,#41947,#41948,#41949,#41950,#41951,
#41952,#41953,#41954,#41955,#41956,#41957,#41958,#41959,#41960,#41961,#41962,
#41963,#41964,#41965,#41966,#41967,#41968,#41969,#41970,#41971,#41972,#41973,
#41974,#41975,#41976,#41977,#41978,#41979,#41980,#41981,#41982,#41983,#41984,
#41985,#41986,#41987,#41988,#41989,#41990,#41991,#41992,#41993,#41994,#41995,
#41996,#41997,#41998,#41999,#42000,#42001,#42002,#42003,#42004,#42005,#42006,
#42007,#42008,#42009,#42010,#42011,#42012,#42013,#42014,#42015,#42016,#42017,
#42018),.UNSPECIFIED.,.F.,.F.,(4,3,3,3,3,3,3,3,3,3,3,3,3,3,3,3,3,3,3,3,
3,3,3,3,3,3,3,3,3,3,3,4),(0.,0.0317392926390111,0.06427104971894,0.0974907111890735,
0.129407560650786,0.134009775207885,0.138840345930619,0.172956078855192,
0.207581704666645,0.243892655220677,0.271125868136201,0.277136000189074,
0.312751944561103,0.348252900965451,0.352825506882774,0.387546395149149,
0.409444620986338,0.417180295663684,0.422139723441818,0.457113952190099,
0.493314028911904,0.529906445847685,0.555907891184747,0.563763452421676,
0.571495289748545,0.608811765665218,0.641088326384959,0.655846951854627,
0.662600712364462,0.700434559793948,0.737918008544181,0.757763664684543),
 .UNSPECIFIED.);
#2940=B_SPLINE_CURVE_WITH_KNOTS('',3,(#42019,#42020,#42021,#42022,#42023,
#42024,#42025,#42026,#42027,#42028,#42029,#42030,#42031,#42032,#42033,#42034,
#42035,#42036,#42037,#42038,#42039,#42040,#42041,#42042,#42043),
 .UNSPECIFIED.,.F.,.F.,(4,3,3,3,3,3,3,3,4),(-10.1336107523121,-9.84512596343066,
-8.86061336708759,-7.87610077074453,-6.89158817440147,-5.9070755780584,
-4.92256298171533,-3.93805038537227,-3.85042544513253),.UNSPECIFIED.);
#2941=B_SPLINE_CURVE_WITH_KNOTS('',3,(#42248,#42249,#42250,#42251,#42252,
#42253,#42254,#42255,#42256,#42257,#42258,#42259,#42260,#42261,#42262,#42263,
#42264,#42265,#42266,#42267,#42268,#42269,#42270,#42271,#42272),
 .UNSPECIFIED.,.F.,.F.,(4,3,3,3,3,3,3,3,4),(7.592022928411,7.87610077074452,
8.86061336708759,9.84512596343066,10.8296385597737,11.8141511561168,12.7986637524599,
13.7831763488029,13.8752082355906),.UNSPECIFIED.);
#2942=B_SPLINE_CURVE_WITH_KNOTS('',3,(#42273,#42274,#42275,#42276,#42277,
#42278,#42279,#42280,#42281,#42282,#42283,#42284,#42285,#42286,#42287,#42288,
#42289,#42290,#42291,#42292,#42293,#42294,#42295,#42296,#42297,#42298,#42299,
#42300,#42301,#42302,#42303,#42304,#42305,#42306,#42307,#42308,#42309,#42310,
#42311,#42312,#42313,#42314,#42315,#42316,#42317,#42318,#42319,#42320,#42321,
#42322,#42323,#42324,#42325,#42326,#42327,#42328,#42329,#42330,#42331,#42332,
#42333,#42334,#42335,#42336,#42337,#42338,#42339,#42340,#42341,#42342,#42343,
#42344,#42345,#42346,#42347,#42348,#42349,#42350,#42351,#42352,#42353,#42354,
#42355,#42356,#42357,#42358,#42359,#42360,#42361,#42362,#42363,#42364,#42365,
#42366,#42367,#42368,#42369),.UNSPECIFIED.,.F.,.F.,(4,3,3,3,3,3,3,3,3,3,
3,3,3,3,3,3,3,3,3,3,3,3,3,3,3,3,3,3,3,3,3,3,4),(0.,0.0368231487405989,0.0744314261587949,
0.113698809813578,0.148057770511513,0.15481009538365,0.159905443760235,
0.196856403615778,0.233660968511241,0.269922874636576,0.299584779826697,
0.306586732072781,0.311530477043913,0.34706791893824,0.381889563649704,
0.388570495397059,0.424561733289204,0.444531526044614,0.452400923962074,
0.457441217806984,0.493270867753082,0.528364029290525,0.56305044901109,
0.585678945056675,0.594960393985588,0.600628220264455,0.634676041165029,
0.662026635217714,0.675581361298493,0.683279765486755,0.715772824187495,
0.74407841737577,0.760759816994523),.UNSPECIFIED.);
#2943=B_SPLINE_CURVE_WITH_KNOTS('',3,(#42372,#42373,#42374,#42375,#42376,
#42377,#42378,#42379,#42380,#42381,#42382,#42383,#42384,#42385,#42386,#42387,
#42388,#42389,#42390,#42391,#42392,#42393,#42394,#42395,#42396,#42397,#42398,
#42399,#42400,#42401,#42402,#42403,#42404,#42405,#42406,#42407,#42408,#42409,
#42410,#42411,#42412,#42413,#42414,#42415,#42416,#42417,#42418,#42419,#42420,
#42421,#42422,#42423,#42424,#42425,#42426,#42427,#42428,#42429,#42430,#42431,
#42432,#42433,#42434,#42435,#42436,#42437,#42438,#42439,#42440,#42441,#42442,
#42443,#42444,#42445,#42446,#42447,#42448,#42449,#42450,#42451,#42452,#42453,
#42454,#42455,#42456,#42457,#42458,#42459,#42460,#42461,#42462,#42463,#42464,
#42465,#42466,#42467,#42468,#42469,#42470,#42471),.UNSPECIFIED.,.F.,.F.,
(4,3,3,3,3,3,3,3,3,3,3,3,3,3,3,3,3,3,3,3,3,3,3,3,3,3,3,3,3,3,3,3,3,4),(-0.760759816994564,
-0.728627854008442,-0.695756675766866,-0.686068398368336,-0.679579388481393,
-0.673178910415624,-0.639342175416784,-0.610292603631362,-0.600454896667282,
-0.594751269714701,-0.5602178744711,-0.525201003137007,-0.490288896523447,
-0.469453072675938,-0.45509359744204,-0.450652627702033,-0.414664207509709,
-0.40694560113341,-0.37234816825657,-0.33700419983174,-0.317186754779825,
-0.308923380424535,-0.304448587240479,-0.268404743404054,-0.231699824208938,
-0.194697408001487,-0.172850866876439,-0.161340463279929,-0.156038382119757,
-0.118189740184684,-0.0802678836542896,-0.0429993965311957,-0.0199250790011036,
0.),.UNSPECIFIED.);
#2944=B_SPLINE_CURVE_WITH_KNOTS('',3,(#42472,#42473,#42474,#42475,#42476,
#42477,#42478,#42479,#42480,#42481,#42482,#42483,#42484,#42485,#42486,#42487,
#42488,#42489,#42490,#42491,#42492,#42493,#42494,#42495,#42496,#42497,#42498,
#42499,#42500,#42501,#42502,#42503,#42504,#42505,#42506,#42507,#42508,#42509,
#42510,#42511,#42512,#42513,#42514,#42515,#42516,#42517,#42518,#42519,#42520,
#42521,#42522,#42523,#42524,#42525,#42526,#42527,#42528,#42529,#42530,#42531,
#42532,#42533,#42534,#42535,#42536,#42537,#42538,#42539,#42540,#42541,#42542,
#42543,#42544,#42545,#42546,#42547,#42548,#42549,#42550,#42551,#42552,#42553,
#42554,#42555,#42556,#42557,#42558,#42559,#42560,#42561,#42562,#42563,#42564,
#42565,#42566,#42567,#42568,#42569,#42570,#42571),.UNSPECIFIED.,.F.,.F.,
(4,3,3,3,3,3,3,3,3,3,3,3,3,3,3,3,3,3,3,3,3,3,3,3,3,3,3,3,3,3,3,3,3,4),(-0.757763664684492,
-0.72037767484086,-0.682466697174141,-0.666433210881691,-0.657234612921716,
-0.619826663526386,-0.588739338910877,-0.575138634391592,-0.56771178998584,
-0.562381438442901,-0.525810002728897,-0.48951256756756,-0.454189692426994,
-0.433424285970824,-0.418943941384036,-0.414278009542087,-0.379386449564138,
-0.371128066602314,-0.335727255522783,-0.300034647303691,-0.282321970354399,
-0.2751567520521,-0.270309050351438,-0.235597104423164,-0.200919047261525,
-0.166729828033903,-0.147967576544044,-0.137478161837071,-0.130951777779855,
-0.097559193204338,-0.0646630585919135,-0.0327160968510094,-0.0166318161150306,
0.),.UNSPECIFIED.);
#2945=B_SPLINE_CURVE_WITH_KNOTS('',3,(#42573,#42574,#42575,#42576,#42577,
#42578,#42579,#42580,#42581,#42582,#42583),.UNSPECIFIED.,.F.,.F.,(4,1,1,
1,1,1,1,1,4),(15.7079632679489,15.7955882081887,16.7801008045318,17.7646134008748,
18.7491259972179,19.733638593561,20.718151189904,21.7026637862471,21.9911485751285),
 .UNSPECIFIED.);
#2946=B_SPLINE_CURVE_WITH_KNOTS('',3,(#42584,#42585,#42586,#42587,#42588,
#42589,#42590,#42591,#42592,#42593),.UNSPECIFIED.,.F.,.F.,(4,1,1,1,1,1,
1,4),(15.7079632679489,16.3681508394037,17.3526634357467,18.3371760320898,
19.3216886284329,20.3062012247759,21.290713821119,21.9911485751285),
 .UNSPECIFIED.);
#2947=B_SPLINE_CURVE_WITH_KNOTS('',3,(#42798,#42799,#42800,#42801,#42802,
#42803,#42804,#42805,#42806,#42807,#42808,#42809,#42810,#42811,#42812,#42813,
#42814,#42815,#42816,#42817,#42818,#42819,#42820,#42821,#42822,#42823,#42824,
#42825,#42826,#42827,#42828,#42829,#42830,#42831,#42832,#42833,#42834,#42835,
#42836,#42837,#42838,#42839,#42840,#42841,#42842,#42843,#42844,#42845,#42846,
#42847,#42848,#42849,#42850,#42851,#42852,#42853,#42854,#42855,#42856,#42857,
#42858,#42859,#42860,#42861,#42862,#42863,#42864,#42865,#42866,#42867,#42868,
#42869,#42870,#42871,#42872,#42873,#42874,#42875,#42876,#42877,#42878,#42879,
#42880,#42881,#42882,#42883,#42884,#42885,#42886,#42887,#42888,#42889,#42890,
#42891),.UNSPECIFIED.,.F.,.F.,(4,3,3,3,3,3,3,3,3,3,3,3,3,3,3,3,3,3,3,3,
3,3,3,3,3,3,3,3,3,3,3,4),(0.,0.0317392578223645,0.0642709833499116,0.0974906209103936,
0.129407481656942,0.134009658091857,0.138840325560996,0.172956034648678,
0.20758164844901,0.243892613057452,0.271125836513783,0.277135986973077,
0.312751925881509,0.348252892065859,0.352825506882778,0.387546411589169,
0.409444636398856,0.417180309631433,0.422139749096638,0.45711400101409,
0.493314088775489,0.529906509036106,0.555907946474613,0.56376389125674,
0.571495247015118,0.608811726985233,0.641088297374965,0.655846945118752,
0.662600708826001,0.700434555809607,0.73791800854416,0.757763664684518),
 .UNSPECIFIED.);
#2948=B_SPLINE_CURVE_WITH_KNOTS('',3,(#42892,#42893,#42894,#42895,#42896,
#42897,#42898,#42899,#42900,#42901,#42902,#42903,#42904,#42905,#42906,#42907,
#42908,#42909,#42910,#42911,#42912,#42913,#42914,#42915,#42916),
 .UNSPECIFIED.,.F.,.F.,(4,3,3,3,3,3,3,3,4),(-10.1336107523121,-9.84512596343066,
-8.86061336708759,-7.87610077074453,-6.89158817440146,-5.9070755780584,
-4.92256298171533,-3.93805038537226,-3.85042544513253),.UNSPECIFIED.);
#2949=B_SPLINE_CURVE_WITH_KNOTS('',3,(#43121,#43122,#43123,#43124,#43125,
#43126,#43127,#43128,#43129,#43130,#43131,#43132,#43133,#43134,#43135,#43136,
#43137,#43138,#43139,#43140,#43141,#43142,#43143,#43144,#43145),
 .UNSPECIFIED.,.F.,.F.,(4,3,3,3,3,3,3,3,4),(7.592022928411,7.87610077074453,
8.8606133670876,9.84512596343066,10.8296385597737,11.8141511561168,12.7986637524599,
13.7831763488029,13.8752082355906),.UNSPECIFIED.);
#2950=B_SPLINE_CURVE_WITH_KNOTS('',3,(#43146,#43147,#43148,#43149,#43150,
#43151,#43152,#43153,#43154,#43155,#43156,#43157,#43158,#43159,#43160,#43161,
#43162,#43163,#43164,#43165,#43166,#43167,#43168,#43169,#43170,#43171,#43172,
#43173,#43174,#43175,#43176,#43177,#43178,#43179,#43180,#43181,#43182,#43183,
#43184,#43185,#43186,#43187,#43188,#43189,#43190,#43191,#43192,#43193,#43194,
#43195,#43196,#43197,#43198,#43199,#43200,#43201,#43202,#43203,#43204,#43205,
#43206,#43207,#43208,#43209,#43210,#43211,#43212,#43213,#43214,#43215,#43216,
#43217,#43218,#43219,#43220,#43221,#43222,#43223,#43224,#43225,#43226,#43227,
#43228,#43229,#43230,#43231,#43232,#43233,#43234,#43235,#43236,#43237,#43238,
#43239,#43240,#43241,#43242),.UNSPECIFIED.,.F.,.F.,(4,3,3,3,3,3,3,3,3,3,
3,3,3,3,3,3,3,3,3,3,3,3,3,3,3,3,3,3,3,3,3,3,4),(0.,0.0368231320265742,0.0744314002406353,
0.113698787135186,0.148057750667918,0.154809920619753,0.159905372006135,
0.196856331004292,0.233660900681144,0.269922813568411,0.299584734025569,
0.306586611813478,0.311530355932456,0.347067804301497,0.381889455018008,
0.388570495397043,0.424561732757698,0.444531525546326,0.452400921561243,
0.457441217682179,0.493270867643875,0.528364028783657,0.563050450927217,
0.585678946733283,0.594960344676032,0.600628213104039,0.634676035977772,
0.662026631327266,0.675581362311545,0.683279766638027,0.715772832870445,
0.744078417375749,0.7607598169945),.UNSPECIFIED.);
#3842=LINE('',#31643,#4690);
#3843=LINE('',#31655,#4691);
#3844=LINE('',#31675,#4692);
#3845=LINE('',#31729,#4693);
#3846=LINE('',#31777,#4694);
#3847=LINE('',#31828,#4695);
#3848=LINE('',#31879,#4696);
#3849=LINE('',#31927,#4697);
#3850=LINE('',#31966,#4698);
#3851=LINE('',#31992,#4699);
#3852=LINE('',#32017,#4700);
#3853=LINE('',#32042,#4701);
#3854=LINE('',#32066,#4702);
#3855=LINE('',#32091,#4703);
#3856=LINE('',#32116,#4704);
#3857=LINE('',#32133,#4705);
#3858=LINE('',#32145,#4706);
#3859=LINE('',#32165,#4707);
#3860=LINE('',#32219,#4708);
#3861=LINE('',#32267,#4709);
#3862=LINE('',#32318,#4710);
#3863=LINE('',#32369,#4711);
#3864=LINE('',#32417,#4712);
#3865=LINE('',#32456,#4713);
#3866=LINE('',#32482,#4714);
#3867=LINE('',#32507,#4715);
#3868=LINE('',#32532,#4716);
#3869=LINE('',#32556,#4717);
#3870=LINE('',#32581,#4718);
#3871=LINE('',#32606,#4719);
#3872=LINE('',#32623,#4720);
#3873=LINE('',#32635,#4721);
#3874=LINE('',#32655,#4722);
#3875=LINE('',#32709,#4723);
#3876=LINE('',#32757,#4724);
#3877=LINE('',#32808,#4725);
#3878=LINE('',#32859,#4726);
#3879=LINE('',#32907,#4727);
#3880=LINE('',#32946,#4728);
#3881=LINE('',#32972,#4729);
#3882=LINE('',#32997,#4730);
#3883=LINE('',#33022,#4731);
#3884=LINE('',#33046,#4732);
#3885=LINE('',#33071,#4733);
#3886=LINE('',#33096,#4734);
#3887=LINE('',#33113,#4735);
#3888=LINE('',#33125,#4736);
#3889=LINE('',#33145,#4737);
#3890=LINE('',#33199,#4738);
#3891=LINE('',#33247,#4739);
#3892=LINE('',#33298,#4740);
#3893=LINE('',#33349,#4741);
#3894=LINE('',#33397,#4742);
#3895=LINE('',#33436,#4743);
#3896=LINE('',#33462,#4744);
#3897=LINE('',#33487,#4745);
#3898=LINE('',#33512,#4746);
#3899=LINE('',#33536,#4747);
#3900=LINE('',#33561,#4748);
#3901=LINE('',#33586,#4749);
#3902=LINE('',#33603,#4750);
#3903=LINE('',#33647,#4751);
#3904=LINE('',#33695,#4752);
#3905=LINE('',#33779,#4753);
#3906=LINE('',#33854,#4754);
#3907=LINE('',#33923,#4755);
#3908=LINE('',#33948,#4756);
#3909=LINE('',#33985,#4757);
#3910=LINE('',#34019,#4758);
#3911=LINE('',#34055,#4759);
#3912=LINE('',#34075,#4760);
#3913=LINE('',#34119,#4761);
#3914=LINE('',#34167,#4762);
#3915=LINE('',#34251,#4763);
#3916=LINE('',#34326,#4764);
#3917=LINE('',#34395,#4765);
#3918=LINE('',#34420,#4766);
#3919=LINE('',#34457,#4767);
#3920=LINE('',#34491,#4768);
#3921=LINE('',#34527,#4769);
#3922=LINE('',#34547,#4770);
#3923=LINE('',#34591,#4771);
#3924=LINE('',#34639,#4772);
#3925=LINE('',#34723,#4773);
#3926=LINE('',#34798,#4774);
#3927=LINE('',#34867,#4775);
#3928=LINE('',#34892,#4776);
#3929=LINE('',#34929,#4777);
#3930=LINE('',#34963,#4778);
#3931=LINE('',#34999,#4779);
#3932=LINE('',#35019,#4780);
#3933=LINE('',#35063,#4781);
#3934=LINE('',#35111,#4782);
#3935=LINE('',#35195,#4783);
#3936=LINE('',#35270,#4784);
#3937=LINE('',#35339,#4785);
#3938=LINE('',#35364,#4786);
#3939=LINE('',#35401,#4787);
#3940=LINE('',#35435,#4788);
#3941=LINE('',#35471,#4789);
#3942=LINE('',#43248,#4790);
#3943=LINE('',#43255,#4791);
#3944=LINE('',#43261,#4792);
#4690=VECTOR('',#16840,4.);
#4691=VECTOR('',#16843,4.);
#4692=VECTOR('',#16850,4.);
#4693=VECTOR('',#16853,4.);
#4694=VECTOR('',#16856,4.);
#4695=VECTOR('',#16859,4.);
#4696=VECTOR('',#16862,4.);
#4697=VECTOR('',#16865,4.);
#4698=VECTOR('',#16870,4.085);
#4699=VECTOR('',#16875,4.085);
#4700=VECTOR('',#16878,4.085);
#4701=VECTOR('',#16881,4.085);
#4702=VECTOR('',#16884,4.085);
#4703=VECTOR('',#16887,4.085);
#4704=VECTOR('',#16890,4.085);
#4705=VECTOR('',#16895,4.);
#4706=VECTOR('',#16898,4.);
#4707=VECTOR('',#16905,4.);
#4708=VECTOR('',#16908,4.);
#4709=VECTOR('',#16911,4.);
#4710=VECTOR('',#16914,4.);
#4711=VECTOR('',#16917,4.);
#4712=VECTOR('',#16920,4.);
#4713=VECTOR('',#16925,4.085);
#4714=VECTOR('',#16930,4.085);
#4715=VECTOR('',#16933,4.085);
#4716=VECTOR('',#16936,4.085);
#4717=VECTOR('',#16939,4.085);
#4718=VECTOR('',#16942,4.085);
#4719=VECTOR('',#16945,4.085);
#4720=VECTOR('',#16950,4.);
#4721=VECTOR('',#16953,4.);
#4722=VECTOR('',#16960,4.);
#4723=VECTOR('',#16963,4.);
#4724=VECTOR('',#16966,4.);
#4725=VECTOR('',#16969,4.);
#4726=VECTOR('',#16972,4.);
#4727=VECTOR('',#16975,4.);
#4728=VECTOR('',#16980,4.085);
#4729=VECTOR('',#16985,4.085);
#4730=VECTOR('',#16988,4.085);
#4731=VECTOR('',#16991,4.085);
#4732=VECTOR('',#16994,4.085);
#4733=VECTOR('',#16997,4.085);
#4734=VECTOR('',#17000,4.085);
#4735=VECTOR('',#17005,4.);
#4736=VECTOR('',#17008,4.);
#4737=VECTOR('',#17015,4.);
#4738=VECTOR('',#17018,4.);
#4739=VECTOR('',#17021,4.);
#4740=VECTOR('',#17024,4.);
#4741=VECTOR('',#17027,4.);
#4742=VECTOR('',#17030,4.);
#4743=VECTOR('',#17035,4.085);
#4744=VECTOR('',#17040,4.085);
#4745=VECTOR('',#17043,4.085);
#4746=VECTOR('',#17046,4.085);
#4747=VECTOR('',#17049,4.085);
#4748=VECTOR('',#17052,4.085);
#4749=VECTOR('',#17055,4.085);
#4750=VECTOR('',#17060,5.);
#4751=VECTOR('',#17063,5.);
#4752=VECTOR('',#17068,5.);
#4753=VECTOR('',#17071,5.);
#4754=VECTOR('',#17074,5.);
#4755=VECTOR('',#17079,5.099);
#4756=VECTOR('',#17084,5.099);
#4757=VECTOR('',#17087,5.099);
#4758=VECTOR('',#17090,5.099);
#4759=VECTOR('',#17093,5.099);
#4760=VECTOR('',#17098,5.);
#4761=VECTOR('',#17101,5.);
#4762=VECTOR('',#17106,5.);
#4763=VECTOR('',#17109,5.);
#4764=VECTOR('',#17112,5.);
#4765=VECTOR('',#17117,5.099);
#4766=VECTOR('',#17122,5.099);
#4767=VECTOR('',#17125,5.099);
#4768=VECTOR('',#17128,5.099);
#4769=VECTOR('',#17131,5.099);
#4770=VECTOR('',#17136,5.);
#4771=VECTOR('',#17139,5.);
#4772=VECTOR('',#17144,5.);
#4773=VECTOR('',#17147,5.);
#4774=VECTOR('',#17150,5.);
#4775=VECTOR('',#17155,5.099);
#4776=VECTOR('',#17160,5.099);
#4777=VECTOR('',#17163,5.099);
#4778=VECTOR('',#17166,5.099);
#4779=VECTOR('',#17169,5.099);
#4780=VECTOR('',#17174,5.);
#4781=VECTOR('',#17177,5.);
#4782=VECTOR('',#17182,5.);
#4783=VECTOR('',#17185,5.);
#4784=VECTOR('',#17188,5.);
#4785=VECTOR('',#17193,5.099);
#4786=VECTOR('',#17198,5.099);
#4787=VECTOR('',#17201,5.099);
#4788=VECTOR('',#17204,5.099);
#4789=VECTOR('',#17207,5.099);
#4790=VECTOR('',#17270,40.);
#4791=VECTOR('',#17279,20.);
#4792=VECTOR('',#17286,100.);
#5717=VERTEX_POINT('',#31641);
#5718=VERTEX_POINT('',#31642);
#5719=VERTEX_POINT('',#31644);
#5720=VERTEX_POINT('',#31652);
#5721=VERTEX_POINT('',#31654);
#5722=VERTEX_POINT('',#31657);
#5723=VERTEX_POINT('',#31673);
#5724=VERTEX_POINT('',#31674);
#5725=VERTEX_POINT('',#31727);
#5726=VERTEX_POINT('',#31728);
#5727=VERTEX_POINT('',#31775);
#5728=VERTEX_POINT('',#31776);
#5729=VERTEX_POINT('',#31826);
#5730=VERTEX_POINT('',#31827);
#5731=VERTEX_POINT('',#31877);
#5732=VERTEX_POINT('',#31878);
#5733=VERTEX_POINT('',#31925);
#5734=VERTEX_POINT('',#31926);
#5735=VERTEX_POINT('',#31928);
#5736=VERTEX_POINT('',#31942);
#5737=VERTEX_POINT('',#31964);
#5738=VERTEX_POINT('',#31965);
#5739=VERTEX_POINT('',#31967);
#5740=VERTEX_POINT('',#31977);
#5741=VERTEX_POINT('',#31990);
#5742=VERTEX_POINT('',#31991);
#5743=VERTEX_POINT('',#32015);
#5744=VERTEX_POINT('',#32016);
#5745=VERTEX_POINT('',#32040);
#5746=VERTEX_POINT('',#32041);
#5747=VERTEX_POINT('',#32064);
#5748=VERTEX_POINT('',#32065);
#5749=VERTEX_POINT('',#32089);
#5750=VERTEX_POINT('',#32090);
#5751=VERTEX_POINT('',#32114);
#5752=VERTEX_POINT('',#32115);
#5753=VERTEX_POINT('',#32117);
#5754=VERTEX_POINT('',#32123);
#5755=VERTEX_POINT('',#32131);
#5756=VERTEX_POINT('',#32132);
#5757=VERTEX_POINT('',#32134);
#5758=VERTEX_POINT('',#32142);
#5759=VERTEX_POINT('',#32144);
#5760=VERTEX_POINT('',#32147);
#5761=VERTEX_POINT('',#32163);
#5762=VERTEX_POINT('',#32164);
#5763=VERTEX_POINT('',#32217);
#5764=VERTEX_POINT('',#32218);
#5765=VERTEX_POINT('',#32265);
#5766=VERTEX_POINT('',#32266);
#5767=VERTEX_POINT('',#32316);
#5768=VERTEX_POINT('',#32317);
#5769=VERTEX_POINT('',#32367);
#5770=VERTEX_POINT('',#32368);
#5771=VERTEX_POINT('',#32415);
#5772=VERTEX_POINT('',#32416);
#5773=VERTEX_POINT('',#32418);
#5774=VERTEX_POINT('',#32432);
#5775=VERTEX_POINT('',#32454);
#5776=VERTEX_POINT('',#32455);
#5777=VERTEX_POINT('',#32457);
#5778=VERTEX_POINT('',#32467);
#5779=VERTEX_POINT('',#32480);
#5780=VERTEX_POINT('',#32481);
#5781=VERTEX_POINT('',#32505);
#5782=VERTEX_POINT('',#32506);
#5783=VERTEX_POINT('',#32530);
#5784=VERTEX_POINT('',#32531);
#5785=VERTEX_POINT('',#32554);
#5786=VERTEX_POINT('',#32555);
#5787=VERTEX_POINT('',#32579);
#5788=VERTEX_POINT('',#32580);
#5789=VERTEX_POINT('',#32604);
#5790=VERTEX_POINT('',#32605);
#5791=VERTEX_POINT('',#32607);
#5792=VERTEX_POINT('',#32613);
#5793=VERTEX_POINT('',#32621);
#5794=VERTEX_POINT('',#32622);
#5795=VERTEX_POINT('',#32624);
#5796=VERTEX_POINT('',#32632);
#5797=VERTEX_POINT('',#32634);
#5798=VERTEX_POINT('',#32637);
#5799=VERTEX_POINT('',#32653);
#5800=VERTEX_POINT('',#32654);
#5801=VERTEX_POINT('',#32707);
#5802=VERTEX_POINT('',#32708);
#5803=VERTEX_POINT('',#32755);
#5804=VERTEX_POINT('',#32756);
#5805=VERTEX_POINT('',#32806);
#5806=VERTEX_POINT('',#32807);
#5807=VERTEX_POINT('',#32857);
#5808=VERTEX_POINT('',#32858);
#5809=VERTEX_POINT('',#32905);
#5810=VERTEX_POINT('',#32906);
#5811=VERTEX_POINT('',#32908);
#5812=VERTEX_POINT('',#32922);
#5813=VERTEX_POINT('',#32944);
#5814=VERTEX_POINT('',#32945);
#5815=VERTEX_POINT('',#32947);
#5816=VERTEX_POINT('',#32957);
#5817=VERTEX_POINT('',#32970);
#5818=VERTEX_POINT('',#32971);
#5819=VERTEX_POINT('',#32995);
#5820=VERTEX_POINT('',#32996);
#5821=VERTEX_POINT('',#33020);
#5822=VERTEX_POINT('',#33021);
#5823=VERTEX_POINT('',#33044);
#5824=VERTEX_POINT('',#33045);
#5825=VERTEX_POINT('',#33069);
#5826=VERTEX_POINT('',#33070);
#5827=VERTEX_POINT('',#33094);
#5828=VERTEX_POINT('',#33095);
#5829=VERTEX_POINT('',#33097);
#5830=VERTEX_POINT('',#33103);
#5831=VERTEX_POINT('',#33111);
#5832=VERTEX_POINT('',#33112);
#5833=VERTEX_POINT('',#33114);
#5834=VERTEX_POINT('',#33122);
#5835=VERTEX_POINT('',#33124);
#5836=VERTEX_POINT('',#33127);
#5837=VERTEX_POINT('',#33143);
#5838=VERTEX_POINT('',#33144);
#5839=VERTEX_POINT('',#33197);
#5840=VERTEX_POINT('',#33198);
#5841=VERTEX_POINT('',#33245);
#5842=VERTEX_POINT('',#33246);
#5843=VERTEX_POINT('',#33296);
#5844=VERTEX_POINT('',#33297);
#5845=VERTEX_POINT('',#33347);
#5846=VERTEX_POINT('',#33348);
#5847=VERTEX_POINT('',#33395);
#5848=VERTEX_POINT('',#33396);
#5849=VERTEX_POINT('',#33398);
#5850=VERTEX_POINT('',#33412);
#5851=VERTEX_POINT('',#33434);
#5852=VERTEX_POINT('',#33435);
#5853=VERTEX_POINT('',#33437);
#5854=VERTEX_POINT('',#33447);
#5855=VERTEX_POINT('',#33460);
#5856=VERTEX_POINT('',#33461);
#5857=VERTEX_POINT('',#33485);
#5858=VERTEX_POINT('',#33486);
#5859=VERTEX_POINT('',#33510);
#5860=VERTEX_POINT('',#33511);
#5861=VERTEX_POINT('',#33534);
#5862=VERTEX_POINT('',#33535);
#5863=VERTEX_POINT('',#33559);
#5864=VERTEX_POINT('',#33560);
#5865=VERTEX_POINT('',#33584);
#5866=VERTEX_POINT('',#33585);
#5867=VERTEX_POINT('',#33587);
#5868=VERTEX_POINT('',#33593);
#5869=VERTEX_POINT('',#33601);
#5870=VERTEX_POINT('',#33602);
#5871=VERTEX_POINT('',#33604);
#5872=VERTEX_POINT('',#33639);
#5873=VERTEX_POINT('',#33641);
#5874=VERTEX_POINT('',#33646);
#5875=VERTEX_POINT('',#33693);
#5876=VERTEX_POINT('',#33694);
#5877=VERTEX_POINT('',#33777);
#5878=VERTEX_POINT('',#33778);
#5879=VERTEX_POINT('',#33852);
#5880=VERTEX_POINT('',#33853);
#5881=VERTEX_POINT('',#33855);
#5882=VERTEX_POINT('',#33881);
#5883=VERTEX_POINT('',#33921);
#5884=VERTEX_POINT('',#33922);
#5885=VERTEX_POINT('',#33924);
#5886=VERTEX_POINT('',#33933);
#5887=VERTEX_POINT('',#33946);
#5888=VERTEX_POINT('',#33947);
#5889=VERTEX_POINT('',#33983);
#5890=VERTEX_POINT('',#33984);
#5891=VERTEX_POINT('',#34017);
#5892=VERTEX_POINT('',#34018);
#5893=VERTEX_POINT('',#34053);
#5894=VERTEX_POINT('',#34054);
#5895=VERTEX_POINT('',#34056);
#5896=VERTEX_POINT('',#34063);
#5897=VERTEX_POINT('',#34073);
#5898=VERTEX_POINT('',#34074);
#5899=VERTEX_POINT('',#34076);
#5900=VERTEX_POINT('',#34111);
#5901=VERTEX_POINT('',#34113);
#5902=VERTEX_POINT('',#34118);
#5903=VERTEX_POINT('',#34165);
#5904=VERTEX_POINT('',#34166);
#5905=VERTEX_POINT('',#34249);
#5906=VERTEX_POINT('',#34250);
#5907=VERTEX_POINT('',#34324);
#5908=VERTEX_POINT('',#34325);
#5909=VERTEX_POINT('',#34327);
#5910=VERTEX_POINT('',#34353);
#5911=VERTEX_POINT('',#34393);
#5912=VERTEX_POINT('',#34394);
#5913=VERTEX_POINT('',#34396);
#5914=VERTEX_POINT('',#34405);
#5915=VERTEX_POINT('',#34418);
#5916=VERTEX_POINT('',#34419);
#5917=VERTEX_POINT('',#34455);
#5918=VERTEX_POINT('',#34456);
#5919=VERTEX_POINT('',#34489);
#5920=VERTEX_POINT('',#34490);
#5921=VERTEX_POINT('',#34525);
#5922=VERTEX_POINT('',#34526);
#5923=VERTEX_POINT('',#34528);
#5924=VERTEX_POINT('',#34535);
#5925=VERTEX_POINT('',#34545);
#5926=VERTEX_POINT('',#34546);
#5927=VERTEX_POINT('',#34548);
#5928=VERTEX_POINT('',#34583);
#5929=VERTEX_POINT('',#34585);
#5930=VERTEX_POINT('',#34590);
#5931=VERTEX_POINT('',#34637);
#5932=VERTEX_POINT('',#34638);
#5933=VERTEX_POINT('',#34721);
#5934=VERTEX_POINT('',#34722);
#5935=VERTEX_POINT('',#34796);
#5936=VERTEX_POINT('',#34797);
#5937=VERTEX_POINT('',#34799);
#5938=VERTEX_POINT('',#34825);
#5939=VERTEX_POINT('',#34865);
#5940=VERTEX_POINT('',#34866);
#5941=VERTEX_POINT('',#34868);
#5942=VERTEX_POINT('',#34877);
#5943=VERTEX_POINT('',#34890);
#5944=VERTEX_POINT('',#34891);
#5945=VERTEX_POINT('',#34927);
#5946=VERTEX_POINT('',#34928);
#5947=VERTEX_POINT('',#34961);
#5948=VERTEX_POINT('',#34962);
#5949=VERTEX_POINT('',#34997);
#5950=VERTEX_POINT('',#34998);
#5951=VERTEX_POINT('',#35000);
#5952=VERTEX_POINT('',#35007);
#5953=VERTEX_POINT('',#35017);
#5954=VERTEX_POINT('',#35018);
#5955=VERTEX_POINT('',#35020);
#5956=VERTEX_POINT('',#35055);
#5957=VERTEX_POINT('',#35057);
#5958=VERTEX_POINT('',#35062);
#5959=VERTEX_POINT('',#35109);
#5960=VERTEX_POINT('',#35110);
#5961=VERTEX_POINT('',#35193);
#5962=VERTEX_POINT('',#35194);
#5963=VERTEX_POINT('',#35268);
#5964=VERTEX_POINT('',#35269);
#5965=VERTEX_POINT('',#35271);
#5966=VERTEX_POINT('',#35297);
#5967=VERTEX_POINT('',#35337);
#5968=VERTEX_POINT('',#35338);
#5969=VERTEX_POINT('',#35340);
#5970=VERTEX_POINT('',#35349);
#5971=VERTEX_POINT('',#35362);
#5972=VERTEX_POINT('',#35363);
#5973=VERTEX_POINT('',#35399);
#5974=VERTEX_POINT('',#35400);
#5975=VERTEX_POINT('',#35433);
#5976=VERTEX_POINT('',#35434);
#5977=VERTEX_POINT('',#35469);
#5978=VERTEX_POINT('',#35470);
#5979=VERTEX_POINT('',#35472);
#5980=VERTEX_POINT('',#35479);
#5981=VERTEX_POINT('',#43245);
#5982=VERTEX_POINT('',#43247);
#5983=VERTEX_POINT('',#43251);
#5984=VERTEX_POINT('',#43254);
#5985=VERTEX_POINT('',#43258);
#5986=VERTEX_POINT('',#43260);
#7450=EDGE_CURVE('',#5717,#5718,#3842,.T.);
#7451=EDGE_CURVE('',#5718,#5719,#2699,.T.);
#7452=EDGE_CURVE('',#5719,#5720,#2237,.T.);
#7453=EDGE_CURVE('',#5720,#5721,#3843,.T.);
#7454=EDGE_CURVE('',#5721,#5721,#2238,.F.);
#7455=EDGE_CURVE('',#5720,#5722,#2239,.T.);
#7456=EDGE_CURVE('',#5722,#5717,#2700,.T.);
#7457=EDGE_CURVE('',#5723,#5724,#3844,.T.);
#7458=EDGE_CURVE('',#5724,#5718,#2701,.T.);
#7459=EDGE_CURVE('',#5717,#5723,#2702,.T.);
#7460=EDGE_CURVE('',#5725,#5726,#3845,.T.);
#7461=EDGE_CURVE('',#5726,#5724,#2703,.T.);
#7462=EDGE_CURVE('',#5723,#5725,#2704,.T.);
#7463=EDGE_CURVE('',#5727,#5728,#3846,.T.);
#7464=EDGE_CURVE('',#5728,#5726,#2705,.T.);
#7465=EDGE_CURVE('',#5725,#5727,#2706,.T.);
#7466=EDGE_CURVE('',#5729,#5730,#3847,.T.);
#7467=EDGE_CURVE('',#5730,#5728,#2707,.T.);
#7468=EDGE_CURVE('',#5727,#5729,#2708,.T.);
#7469=EDGE_CURVE('',#5731,#5732,#3848,.T.);
#7470=EDGE_CURVE('',#5732,#5730,#2709,.T.);
#7471=EDGE_CURVE('',#5729,#5731,#2710,.T.);
#7472=EDGE_CURVE('',#5733,#5734,#3849,.T.);
#7473=EDGE_CURVE('',#5733,#5735,#2711,.T.);
#7474=EDGE_CURVE('',#5736,#5735,#2240,.T.);
#7475=EDGE_CURVE('',#5736,#5734,#2712,.T.);
#7476=EDGE_CURVE('',#5737,#5738,#3850,.T.);
#7477=EDGE_CURVE('',#5738,#5739,#2713,.T.);
#7478=EDGE_CURVE('',#5740,#5739,#2241,.T.);
#7479=EDGE_CURVE('',#5737,#5740,#2714,.T.);
#7480=EDGE_CURVE('',#5741,#5742,#3851,.T.);
#7481=EDGE_CURVE('',#5742,#5738,#2715,.T.);
#7482=EDGE_CURVE('',#5741,#5737,#2716,.T.);
#7483=EDGE_CURVE('',#5743,#5744,#3852,.T.);
#7484=EDGE_CURVE('',#5744,#5742,#2717,.T.);
#7485=EDGE_CURVE('',#5743,#5741,#2718,.T.);
#7486=EDGE_CURVE('',#5745,#5746,#3853,.T.);
#7487=EDGE_CURVE('',#5746,#5744,#2719,.T.);
#7488=EDGE_CURVE('',#5745,#5743,#2720,.T.);
#7489=EDGE_CURVE('',#5747,#5748,#3854,.T.);
#7490=EDGE_CURVE('',#5748,#5746,#2721,.T.);
#7491=EDGE_CURVE('',#5747,#5745,#2722,.T.);
#7492=EDGE_CURVE('',#5749,#5750,#3855,.T.);
#7493=EDGE_CURVE('',#5750,#5748,#2723,.T.);
#7494=EDGE_CURVE('',#5749,#5747,#2724,.T.);
#7495=EDGE_CURVE('',#5751,#5752,#3856,.T.);
#7496=EDGE_CURVE('',#5753,#5751,#2725,.T.);
#7497=EDGE_CURVE('',#5754,#5753,#2242,.T.);
#7498=EDGE_CURVE('',#5754,#5752,#2726,.T.);
#7499=EDGE_CURVE('',#5755,#5756,#3857,.T.);
#7500=EDGE_CURVE('',#5756,#5757,#2727,.T.);
#7501=EDGE_CURVE('',#5757,#5758,#2243,.T.);
#7502=EDGE_CURVE('',#5758,#5759,#3858,.T.);
#7503=EDGE_CURVE('',#5759,#5759,#2244,.F.);
#7504=EDGE_CURVE('',#5758,#5760,#2245,.T.);
#7505=EDGE_CURVE('',#5760,#5755,#2728,.T.);
#7506=EDGE_CURVE('',#5761,#5762,#3859,.T.);
#7507=EDGE_CURVE('',#5762,#5756,#2729,.T.);
#7508=EDGE_CURVE('',#5755,#5761,#2730,.T.);
#7509=EDGE_CURVE('',#5763,#5764,#3860,.T.);
#7510=EDGE_CURVE('',#5764,#5762,#2731,.T.);
#7511=EDGE_CURVE('',#5761,#5763,#2732,.T.);
#7512=EDGE_CURVE('',#5765,#5766,#3861,.T.);
#7513=EDGE_CURVE('',#5766,#5764,#2733,.T.);
#7514=EDGE_CURVE('',#5763,#5765,#2734,.T.);
#7515=EDGE_CURVE('',#5767,#5768,#3862,.T.);
#7516=EDGE_CURVE('',#5768,#5766,#2735,.T.);
#7517=EDGE_CURVE('',#5765,#5767,#2736,.T.);
#7518=EDGE_CURVE('',#5769,#5770,#3863,.T.);
#7519=EDGE_CURVE('',#5770,#5768,#2737,.T.);
#7520=EDGE_CURVE('',#5767,#5769,#2738,.T.);
#7521=EDGE_CURVE('',#5771,#5772,#3864,.T.);
#7522=EDGE_CURVE('',#5771,#5773,#2739,.T.);
#7523=EDGE_CURVE('',#5774,#5773,#2246,.T.);
#7524=EDGE_CURVE('',#5774,#5772,#2740,.T.);
#7525=EDGE_CURVE('',#5775,#5776,#3865,.T.);
#7526=EDGE_CURVE('',#5776,#5777,#2741,.T.);
#7527=EDGE_CURVE('',#5778,#5777,#2247,.T.);
#7528=EDGE_CURVE('',#5775,#5778,#2742,.T.);
#7529=EDGE_CURVE('',#5779,#5780,#3866,.T.);
#7530=EDGE_CURVE('',#5780,#5776,#2743,.T.);
#7531=EDGE_CURVE('',#5779,#5775,#2744,.T.);
#7532=EDGE_CURVE('',#5781,#5782,#3867,.T.);
#7533=EDGE_CURVE('',#5782,#5780,#2745,.T.);
#7534=EDGE_CURVE('',#5781,#5779,#2746,.T.);
#7535=EDGE_CURVE('',#5783,#5784,#3868,.T.);
#7536=EDGE_CURVE('',#5784,#5782,#2747,.T.);
#7537=EDGE_CURVE('',#5783,#5781,#2748,.T.);
#7538=EDGE_CURVE('',#5785,#5786,#3869,.T.);
#7539=EDGE_CURVE('',#5786,#5784,#2749,.T.);
#7540=EDGE_CURVE('',#5785,#5783,#2750,.T.);
#7541=EDGE_CURVE('',#5787,#5788,#3870,.T.);
#7542=EDGE_CURVE('',#5788,#5786,#2751,.T.);
#7543=EDGE_CURVE('',#5787,#5785,#2752,.T.);
#7544=EDGE_CURVE('',#5789,#5790,#3871,.T.);
#7545=EDGE_CURVE('',#5791,#5789,#2753,.T.);
#7546=EDGE_CURVE('',#5792,#5791,#2248,.T.);
#7547=EDGE_CURVE('',#5792,#5790,#2754,.T.);
#7548=EDGE_CURVE('',#5793,#5794,#3872,.T.);
#7549=EDGE_CURVE('',#5794,#5795,#2755,.T.);
#7550=EDGE_CURVE('',#5795,#5796,#2249,.T.);
#7551=EDGE_CURVE('',#5796,#5797,#3873,.T.);
#7552=EDGE_CURVE('',#5797,#5797,#2250,.F.);
#7553=EDGE_CURVE('',#5796,#5798,#2251,.T.);
#7554=EDGE_CURVE('',#5798,#5793,#2756,.T.);
#7555=EDGE_CURVE('',#5799,#5800,#3874,.T.);
#7556=EDGE_CURVE('',#5800,#5794,#2757,.T.);
#7557=EDGE_CURVE('',#5793,#5799,#2758,.T.);
#7558=EDGE_CURVE('',#5801,#5802,#3875,.T.);
#7559=EDGE_CURVE('',#5802,#5800,#2759,.T.);
#7560=EDGE_CURVE('',#5799,#5801,#2760,.T.);
#7561=EDGE_CURVE('',#5803,#5804,#3876,.T.);
#7562=EDGE_CURVE('',#5804,#5802,#2761,.T.);
#7563=EDGE_CURVE('',#5801,#5803,#2762,.T.);
#7564=EDGE_CURVE('',#5805,#5806,#3877,.T.);
#7565=EDGE_CURVE('',#5806,#5804,#2763,.T.);
#7566=EDGE_CURVE('',#5803,#5805,#2764,.T.);
#7567=EDGE_CURVE('',#5807,#5808,#3878,.T.);
#7568=EDGE_CURVE('',#5808,#5806,#2765,.T.);
#7569=EDGE_CURVE('',#5805,#5807,#2766,.T.);
#7570=EDGE_CURVE('',#5809,#5810,#3879,.T.);
#7571=EDGE_CURVE('',#5809,#5811,#2767,.T.);
#7572=EDGE_CURVE('',#5812,#5811,#2252,.T.);
#7573=EDGE_CURVE('',#5812,#5810,#2768,.T.);
#7574=EDGE_CURVE('',#5813,#5814,#3880,.T.);
#7575=EDGE_CURVE('',#5814,#5815,#2769,.T.);
#7576=EDGE_CURVE('',#5816,#5815,#2253,.T.);
#7577=EDGE_CURVE('',#5813,#5816,#2770,.T.);
#7578=EDGE_CURVE('',#5817,#5818,#3881,.T.);
#7579=EDGE_CURVE('',#5818,#5814,#2771,.T.);
#7580=EDGE_CURVE('',#5817,#5813,#2772,.T.);
#7581=EDGE_CURVE('',#5819,#5820,#3882,.T.);
#7582=EDGE_CURVE('',#5820,#5818,#2773,.T.);
#7583=EDGE_CURVE('',#5819,#5817,#2774,.T.);
#7584=EDGE_CURVE('',#5821,#5822,#3883,.T.);
#7585=EDGE_CURVE('',#5822,#5820,#2775,.T.);
#7586=EDGE_CURVE('',#5821,#5819,#2776,.T.);
#7587=EDGE_CURVE('',#5823,#5824,#3884,.T.);
#7588=EDGE_CURVE('',#5824,#5822,#2777,.T.);
#7589=EDGE_CURVE('',#5823,#5821,#2778,.T.);
#7590=EDGE_CURVE('',#5825,#5826,#3885,.T.);
#7591=EDGE_CURVE('',#5826,#5824,#2779,.T.);
#7592=EDGE_CURVE('',#5825,#5823,#2780,.T.);
#7593=EDGE_CURVE('',#5827,#5828,#3886,.T.);
#7594=EDGE_CURVE('',#5829,#5827,#2781,.T.);
#7595=EDGE_CURVE('',#5830,#5829,#2254,.T.);
#7596=EDGE_CURVE('',#5830,#5828,#2782,.T.);
#7597=EDGE_CURVE('',#5831,#5832,#3887,.T.);
#7598=EDGE_CURVE('',#5832,#5833,#2783,.T.);
#7599=EDGE_CURVE('',#5833,#5834,#2255,.T.);
#7600=EDGE_CURVE('',#5834,#5835,#3888,.T.);
#7601=EDGE_CURVE('',#5835,#5835,#2256,.F.);
#7602=EDGE_CURVE('',#5834,#5836,#2257,.T.);
#7603=EDGE_CURVE('',#5836,#5831,#2784,.T.);
#7604=EDGE_CURVE('',#5837,#5838,#3889,.T.);
#7605=EDGE_CURVE('',#5838,#5832,#2785,.T.);
#7606=EDGE_CURVE('',#5831,#5837,#2786,.T.);
#7607=EDGE_CURVE('',#5839,#5840,#3890,.T.);
#7608=EDGE_CURVE('',#5840,#5838,#2787,.T.);
#7609=EDGE_CURVE('',#5837,#5839,#2788,.T.);
#7610=EDGE_CURVE('',#5841,#5842,#3891,.T.);
#7611=EDGE_CURVE('',#5842,#5840,#2789,.T.);
#7612=EDGE_CURVE('',#5839,#5841,#2790,.T.);
#7613=EDGE_CURVE('',#5843,#5844,#3892,.T.);
#7614=EDGE_CURVE('',#5844,#5842,#2791,.T.);
#7615=EDGE_CURVE('',#5841,#5843,#2792,.T.);
#7616=EDGE_CURVE('',#5845,#5846,#3893,.T.);
#7617=EDGE_CURVE('',#5846,#5844,#2793,.T.);
#7618=EDGE_CURVE('',#5843,#5845,#2794,.T.);
#7619=EDGE_CURVE('',#5847,#5848,#3894,.T.);
#7620=EDGE_CURVE('',#5847,#5849,#2795,.T.);
#7621=EDGE_CURVE('',#5850,#5849,#2258,.T.);
#7622=EDGE_CURVE('',#5850,#5848,#2796,.T.);
#7623=EDGE_CURVE('',#5851,#5852,#3895,.T.);
#7624=EDGE_CURVE('',#5852,#5853,#2797,.T.);
#7625=EDGE_CURVE('',#5854,#5853,#2259,.T.);
#7626=EDGE_CURVE('',#5851,#5854,#2798,.T.);
#7627=EDGE_CURVE('',#5855,#5856,#3896,.T.);
#7628=EDGE_CURVE('',#5856,#5852,#2799,.T.);
#7629=EDGE_CURVE('',#5855,#5851,#2800,.T.);
#7630=EDGE_CURVE('',#5857,#5858,#3897,.T.);
#7631=EDGE_CURVE('',#5858,#5856,#2801,.T.);
#7632=EDGE_CURVE('',#5857,#5855,#2802,.T.);
#7633=EDGE_CURVE('',#5859,#5860,#3898,.T.);
#7634=EDGE_CURVE('',#5860,#5858,#2803,.T.);
#7635=EDGE_CURVE('',#5859,#5857,#2804,.T.);
#7636=EDGE_CURVE('',#5861,#5862,#3899,.T.);
#7637=EDGE_CURVE('',#5862,#5860,#2805,.T.);
#7638=EDGE_CURVE('',#5861,#5859,#2806,.T.);
#7639=EDGE_CURVE('',#5863,#5864,#3900,.T.);
#7640=EDGE_CURVE('',#5864,#5862,#2807,.T.);
#7641=EDGE_CURVE('',#5863,#5861,#2808,.T.);
#7642=EDGE_CURVE('',#5865,#5866,#3901,.T.);
#7643=EDGE_CURVE('',#5867,#5865,#2809,.T.);
#7644=EDGE_CURVE('',#5868,#5867,#2260,.T.);
#7645=EDGE_CURVE('',#5868,#5866,#2810,.T.);
#7646=EDGE_CURVE('',#5869,#5870,#3902,.T.);
#7647=EDGE_CURVE('',#5870,#5871,#2811,.T.);
#7648=EDGE_CURVE('',#5871,#5872,#2261,.T.);
#7649=EDGE_CURVE('',#5872,#5873,#2812,.T.);
#7650=EDGE_CURVE('',#5873,#5874,#3903,.T.);
#7651=EDGE_CURVE('',#5874,#5874,#2262,.F.);
#7652=EDGE_CURVE('',#5873,#5869,#2813,.T.);
#7653=EDGE_CURVE('',#5875,#5876,#3904,.T.);
#7654=EDGE_CURVE('',#5876,#5870,#2814,.T.);
#7655=EDGE_CURVE('',#5869,#5875,#2815,.T.);
#7656=EDGE_CURVE('',#5877,#5878,#3905,.T.);
#7657=EDGE_CURVE('',#5878,#5876,#2816,.T.);
#7658=EDGE_CURVE('',#5875,#5877,#2817,.T.);
#7659=EDGE_CURVE('',#5879,#5880,#3906,.T.);
#7660=EDGE_CURVE('',#5879,#5881,#2818,.T.);
#7661=EDGE_CURVE('',#5882,#5881,#2263,.F.);
#7662=EDGE_CURVE('',#5882,#5880,#2819,.T.);
#7663=EDGE_CURVE('',#5883,#5884,#3907,.T.);
#7664=EDGE_CURVE('',#5884,#5885,#2820,.T.);
#7665=EDGE_CURVE('',#5886,#5885,#2264,.T.);
#7666=EDGE_CURVE('',#5883,#5886,#2821,.T.);
#7667=EDGE_CURVE('',#5887,#5888,#3908,.T.);
#7668=EDGE_CURVE('',#5888,#5884,#2822,.T.);
#7669=EDGE_CURVE('',#5887,#5883,#2823,.T.);
#7670=EDGE_CURVE('',#5889,#5890,#3909,.T.);
#7671=EDGE_CURVE('',#5890,#5888,#2824,.T.);
#7672=EDGE_CURVE('',#5889,#5887,#2825,.T.);
#7673=EDGE_CURVE('',#5891,#5892,#3910,.T.);
#7674=EDGE_CURVE('',#5892,#5890,#2826,.T.);
#7675=EDGE_CURVE('',#5891,#5889,#2827,.T.);
#7676=EDGE_CURVE('',#5893,#5894,#3911,.T.);
#7677=EDGE_CURVE('',#5895,#5893,#2828,.T.);
#7678=EDGE_CURVE('',#5896,#5895,#2265,.T.);
#7679=EDGE_CURVE('',#5896,#5894,#2829,.T.);
#7680=EDGE_CURVE('',#5897,#5898,#3912,.T.);
#7681=EDGE_CURVE('',#5898,#5899,#2830,.T.);
#7682=EDGE_CURVE('',#5899,#5900,#2266,.T.);
#7683=EDGE_CURVE('',#5900,#5901,#2831,.T.);
#7684=EDGE_CURVE('',#5901,#5902,#3913,.T.);
#7685=EDGE_CURVE('',#5902,#5902,#2267,.F.);
#7686=EDGE_CURVE('',#5901,#5897,#2832,.T.);
#7687=EDGE_CURVE('',#5903,#5904,#3914,.T.);
#7688=EDGE_CURVE('',#5904,#5898,#2833,.T.);
#7689=EDGE_CURVE('',#5897,#5903,#2834,.T.);
#7690=EDGE_CURVE('',#5905,#5906,#3915,.T.);
#7691=EDGE_CURVE('',#5906,#5904,#2835,.T.);
#7692=EDGE_CURVE('',#5903,#5905,#2836,.T.);
#7693=EDGE_CURVE('',#5907,#5908,#3916,.T.);
#7694=EDGE_CURVE('',#5907,#5909,#2837,.T.);
#7695=EDGE_CURVE('',#5910,#5909,#2268,.F.);
#7696=EDGE_CURVE('',#5910,#5908,#2838,.T.);
#7697=EDGE_CURVE('',#5911,#5912,#3917,.T.);
#7698=EDGE_CURVE('',#5912,#5913,#2839,.T.);
#7699=EDGE_CURVE('',#5914,#5913,#2269,.T.);
#7700=EDGE_CURVE('',#5911,#5914,#2840,.T.);
#7701=EDGE_CURVE('',#5915,#5916,#3918,.T.);
#7702=EDGE_CURVE('',#5916,#5912,#2841,.T.);
#7703=EDGE_CURVE('',#5915,#5911,#2842,.T.);
#7704=EDGE_CURVE('',#5917,#5918,#3919,.T.);
#7705=EDGE_CURVE('',#5918,#5916,#2843,.T.);
#7706=EDGE_CURVE('',#5917,#5915,#2844,.T.);
#7707=EDGE_CURVE('',#5919,#5920,#3920,.T.);
#7708=EDGE_CURVE('',#5920,#5918,#2845,.T.);
#7709=EDGE_CURVE('',#5919,#5917,#2846,.T.);
#7710=EDGE_CURVE('',#5921,#5922,#3921,.T.);
#7711=EDGE_CURVE('',#5923,#5921,#2847,.T.);
#7712=EDGE_CURVE('',#5924,#5923,#2270,.T.);
#7713=EDGE_CURVE('',#5924,#5922,#2848,.T.);
#7714=EDGE_CURVE('',#5925,#5926,#3922,.T.);
#7715=EDGE_CURVE('',#5926,#5927,#2849,.T.);
#7716=EDGE_CURVE('',#5927,#5928,#2271,.T.);
#7717=EDGE_CURVE('',#5928,#5929,#2850,.T.);
#7718=EDGE_CURVE('',#5929,#5930,#3923,.T.);
#7719=EDGE_CURVE('',#5930,#5930,#2272,.F.);
#7720=EDGE_CURVE('',#5929,#5925,#2851,.T.);
#7721=EDGE_CURVE('',#5931,#5932,#3924,.T.);
#7722=EDGE_CURVE('',#5932,#5926,#2852,.T.);
#7723=EDGE_CURVE('',#5925,#5931,#2853,.T.);
#7724=EDGE_CURVE('',#5933,#5934,#3925,.T.);
#7725=EDGE_CURVE('',#5934,#5932,#2854,.T.);
#7726=EDGE_CURVE('',#5931,#5933,#2855,.T.);
#7727=EDGE_CURVE('',#5935,#5936,#3926,.T.);
#7728=EDGE_CURVE('',#5935,#5937,#2856,.T.);
#7729=EDGE_CURVE('',#5938,#5937,#2273,.F.);
#7730=EDGE_CURVE('',#5938,#5936,#2857,.T.);
#7731=EDGE_CURVE('',#5939,#5940,#3927,.T.);
#7732=EDGE_CURVE('',#5940,#5941,#2858,.T.);
#7733=EDGE_CURVE('',#5942,#5941,#2274,.T.);
#7734=EDGE_CURVE('',#5939,#5942,#2859,.T.);
#7735=EDGE_CURVE('',#5943,#5944,#3928,.T.);
#7736=EDGE_CURVE('',#5944,#5940,#2860,.T.);
#7737=EDGE_CURVE('',#5943,#5939,#2861,.T.);
#7738=EDGE_CURVE('',#5945,#5946,#3929,.T.);
#7739=EDGE_CURVE('',#5946,#5944,#2862,.T.);
#7740=EDGE_CURVE('',#5945,#5943,#2863,.T.);
#7741=EDGE_CURVE('',#5947,#5948,#3930,.T.);
#7742=EDGE_CURVE('',#5948,#5946,#2864,.T.);
#7743=EDGE_CURVE('',#5947,#5945,#2865,.T.);
#7744=EDGE_CURVE('',#5949,#5950,#3931,.T.);
#7745=EDGE_CURVE('',#5951,#5949,#2866,.T.);
#7746=EDGE_CURVE('',#5952,#5951,#2275,.T.);
#7747=EDGE_CURVE('',#5952,#5950,#2867,.T.);
#7748=EDGE_CURVE('',#5953,#5954,#3932,.T.);
#7749=EDGE_CURVE('',#5954,#5955,#2868,.T.);
#7750=EDGE_CURVE('',#5955,#5956,#2276,.T.);
#7751=EDGE_CURVE('',#5956,#5957,#2869,.T.);
#7752=EDGE_CURVE('',#5957,#5958,#3933,.T.);
#7753=EDGE_CURVE('',#5958,#5958,#2277,.F.);
#7754=EDGE_CURVE('',#5957,#5953,#2870,.T.);
#7755=EDGE_CURVE('',#5959,#5960,#3934,.T.);
#7756=EDGE_CURVE('',#5960,#5954,#2871,.T.);
#7757=EDGE_CURVE('',#5953,#5959,#2872,.T.);
#7758=EDGE_CURVE('',#5961,#5962,#3935,.T.);
#7759=EDGE_CURVE('',#5962,#5960,#2873,.T.);
#7760=EDGE_CURVE('',#5959,#5961,#2874,.T.);
#7761=EDGE_CURVE('',#5963,#5964,#3936,.T.);
#7762=EDGE_CURVE('',#5963,#5965,#2875,.T.);
#7763=EDGE_CURVE('',#5966,#5965,#2278,.F.);
#7764=EDGE_CURVE('',#5966,#5964,#2876,.T.);
#7765=EDGE_CURVE('',#5967,#5968,#3937,.T.);
#7766=EDGE_CURVE('',#5968,#5969,#2877,.T.);
#7767=EDGE_CURVE('',#5970,#5969,#2279,.T.);
#7768=EDGE_CURVE('',#5967,#5970,#2878,.T.);
#7769=EDGE_CURVE('',#5971,#5972,#3938,.T.);
#7770=EDGE_CURVE('',#5972,#5968,#2879,.T.);
#7771=EDGE_CURVE('',#5971,#5967,#2880,.T.);
#7772=EDGE_CURVE('',#5973,#5974,#3939,.T.);
#7773=EDGE_CURVE('',#5974,#5972,#2881,.T.);
#7774=EDGE_CURVE('',#5973,#5971,#2882,.T.);
#7775=EDGE_CURVE('',#5975,#5976,#3940,.T.);
#7776=EDGE_CURVE('',#5976,#5974,#2883,.T.);
#7777=EDGE_CURVE('',#5975,#5973,#2884,.T.);
#7778=EDGE_CURVE('',#5977,#5978,#3941,.T.);
#7779=EDGE_CURVE('',#5979,#5977,#2885,.T.);
#7780=EDGE_CURVE('',#5980,#5979,#2280,.T.);
#7781=EDGE_CURVE('',#5980,#5978,#2886,.T.);
#7782=EDGE_CURVE('',#5955,#5970,#2887,.T.);
#7783=EDGE_CURVE('',#5969,#5956,#2888,.T.);
#7784=EDGE_CURVE('',#5978,#5976,#2889,.T.);
#7785=EDGE_CURVE('',#5977,#5975,#2890,.T.);
#7786=EDGE_CURVE('',#5965,#5980,#2891,.T.);
#7787=EDGE_CURVE('',#5961,#5963,#2892,.T.);
#7788=EDGE_CURVE('',#5964,#5962,#2893,.T.);
#7789=EDGE_CURVE('',#5979,#5966,#2894,.T.);
#7790=EDGE_CURVE('',#5927,#5942,#2895,.T.);
#7791=EDGE_CURVE('',#5941,#5928,#2896,.T.);
#7792=EDGE_CURVE('',#5950,#5948,#2897,.T.);
#7793=EDGE_CURVE('',#5949,#5947,#2898,.T.);
#7794=EDGE_CURVE('',#5937,#5952,#2899,.T.);
#7795=EDGE_CURVE('',#5933,#5935,#2900,.T.);
#7796=EDGE_CURVE('',#5936,#5934,#2901,.T.);
#7797=EDGE_CURVE('',#5951,#5938,#2902,.T.);
#7798=EDGE_CURVE('',#5899,#5914,#2903,.T.);
#7799=EDGE_CURVE('',#5913,#5900,#2904,.T.);
#7800=EDGE_CURVE('',#5922,#5920,#2905,.T.);
#7801=EDGE_CURVE('',#5921,#5919,#2906,.T.);
#7802=EDGE_CURVE('',#5909,#5924,#2907,.T.);
#7803=EDGE_CURVE('',#5905,#5907,#2908,.T.);
#7804=EDGE_CURVE('',#5908,#5906,#2909,.T.);
#7805=EDGE_CURVE('',#5923,#5910,#2910,.T.);
#7806=EDGE_CURVE('',#5871,#5886,#2911,.T.);
#7807=EDGE_CURVE('',#5885,#5872,#2912,.T.);
#7808=EDGE_CURVE('',#5894,#5892,#2913,.T.);
#7809=EDGE_CURVE('',#5893,#5891,#2914,.T.);
#7810=EDGE_CURVE('',#5881,#5896,#2915,.T.);
#7811=EDGE_CURVE('',#5877,#5879,#2916,.T.);
#7812=EDGE_CURVE('',#5880,#5878,#2917,.T.);
#7813=EDGE_CURVE('',#5895,#5882,#2918,.T.);
#7814=EDGE_CURVE('',#5833,#5854,#2919,.T.);
#7815=EDGE_CURVE('',#5853,#5836,#2920,.T.);
#7816=EDGE_CURVE('',#5866,#5864,#2921,.T.);
#7817=EDGE_CURVE('',#5865,#5863,#2922,.T.);
#7818=EDGE_CURVE('',#5849,#5868,#2923,.T.);
#7819=EDGE_CURVE('',#5845,#5847,#2924,.T.);
#7820=EDGE_CURVE('',#5848,#5846,#2925,.T.);
#7821=EDGE_CURVE('',#5867,#5850,#2926,.T.);
#7822=EDGE_CURVE('',#5795,#5816,#2927,.T.);
#7823=EDGE_CURVE('',#5815,#5798,#2928,.T.);
#7824=EDGE_CURVE('',#5828,#5826,#2929,.T.);
#7825=EDGE_CURVE('',#5827,#5825,#2930,.T.);
#7826=EDGE_CURVE('',#5811,#5830,#2931,.T.);
#7827=EDGE_CURVE('',#5807,#5809,#2932,.T.);
#7828=EDGE_CURVE('',#5810,#5808,#2933,.T.);
#7829=EDGE_CURVE('',#5829,#5812,#2934,.T.);
#7830=EDGE_CURVE('',#5757,#5778,#2935,.T.);
#7831=EDGE_CURVE('',#5777,#5760,#2936,.T.);
#7832=EDGE_CURVE('',#5790,#5788,#2937,.T.);
#7833=EDGE_CURVE('',#5789,#5787,#2938,.T.);
#7834=EDGE_CURVE('',#5773,#5792,#2939,.T.);
#7835=EDGE_CURVE('',#5769,#5771,#2940,.T.);
#7836=EDGE_CURVE('',#5772,#5770,#2941,.T.);
#7837=EDGE_CURVE('',#5791,#5774,#2942,.T.);
#7838=EDGE_CURVE('',#5719,#5740,#2943,.T.);
#7839=EDGE_CURVE('',#5739,#5722,#2944,.T.);
#7840=EDGE_CURVE('',#5752,#5750,#2945,.T.);
#7841=EDGE_CURVE('',#5751,#5749,#2946,.T.);
#7842=EDGE_CURVE('',#5735,#5754,#2947,.T.);
#7843=EDGE_CURVE('',#5731,#5733,#2948,.T.);
#7844=EDGE_CURVE('',#5734,#5732,#2949,.T.);
#7845=EDGE_CURVE('',#5753,#5736,#2950,.T.);
#7846=EDGE_CURVE('',#5981,#5981,#2281,.T.);
#7847=EDGE_CURVE('',#5981,#5982,#3942,.T.);
#7848=EDGE_CURVE('',#5982,#5982,#2282,.T.);
#7849=EDGE_CURVE('',#5983,#5983,#2283,.T.);
#7850=EDGE_CURVE('',#5983,#5984,#3943,.T.);
#7851=EDGE_CURVE('',#5984,#5984,#2284,.T.);
#7852=EDGE_CURVE('',#5985,#5985,#2285,.F.);
#7853=EDGE_CURVE('',#5985,#5986,#3944,.T.);
#7854=EDGE_CURVE('',#5986,#5986,#2286,.F.);
#10427=ORIENTED_EDGE('',*,*,#7450,.T.);
#10428=ORIENTED_EDGE('',*,*,#7451,.T.);
#10429=ORIENTED_EDGE('',*,*,#7452,.T.);
#10430=ORIENTED_EDGE('',*,*,#7453,.T.);
#10431=ORIENTED_EDGE('',*,*,#7454,.F.);
#10432=ORIENTED_EDGE('',*,*,#7453,.F.);
#10433=ORIENTED_EDGE('',*,*,#7455,.T.);
#10434=ORIENTED_EDGE('',*,*,#7456,.T.);
#10435=ORIENTED_EDGE('',*,*,#7457,.T.);
#10436=ORIENTED_EDGE('',*,*,#7458,.T.);
#10437=ORIENTED_EDGE('',*,*,#7450,.F.);
#10438=ORIENTED_EDGE('',*,*,#7459,.T.);
#10439=ORIENTED_EDGE('',*,*,#7460,.T.);
#10440=ORIENTED_EDGE('',*,*,#7461,.T.);
#10441=ORIENTED_EDGE('',*,*,#7457,.F.);
#10442=ORIENTED_EDGE('',*,*,#7462,.T.);
#10443=ORIENTED_EDGE('',*,*,#7463,.T.);
#10444=ORIENTED_EDGE('',*,*,#7464,.T.);
#10445=ORIENTED_EDGE('',*,*,#7460,.F.);
#10446=ORIENTED_EDGE('',*,*,#7465,.T.);
#10447=ORIENTED_EDGE('',*,*,#7466,.T.);
#10448=ORIENTED_EDGE('',*,*,#7467,.T.);
#10449=ORIENTED_EDGE('',*,*,#7463,.F.);
#10450=ORIENTED_EDGE('',*,*,#7468,.T.);
#10451=ORIENTED_EDGE('',*,*,#7469,.T.);
#10452=ORIENTED_EDGE('',*,*,#7470,.T.);
#10453=ORIENTED_EDGE('',*,*,#7466,.F.);
#10454=ORIENTED_EDGE('',*,*,#7471,.T.);
#10455=ORIENTED_EDGE('',*,*,#7472,.F.);
#10456=ORIENTED_EDGE('',*,*,#7473,.T.);
#10457=ORIENTED_EDGE('',*,*,#7474,.F.);
#10458=ORIENTED_EDGE('',*,*,#7475,.T.);
#10459=ORIENTED_EDGE('',*,*,#7476,.T.);
#10460=ORIENTED_EDGE('',*,*,#7477,.T.);
#10461=ORIENTED_EDGE('',*,*,#7478,.F.);
#10462=ORIENTED_EDGE('',*,*,#7479,.F.);
#10463=ORIENTED_EDGE('',*,*,#7480,.T.);
#10464=ORIENTED_EDGE('',*,*,#7481,.T.);
#10465=ORIENTED_EDGE('',*,*,#7476,.F.);
#10466=ORIENTED_EDGE('',*,*,#7482,.F.);
#10467=ORIENTED_EDGE('',*,*,#7483,.T.);
#10468=ORIENTED_EDGE('',*,*,#7484,.T.);
#10469=ORIENTED_EDGE('',*,*,#7480,.F.);
#10470=ORIENTED_EDGE('',*,*,#7485,.F.);
#10471=ORIENTED_EDGE('',*,*,#7486,.T.);
#10472=ORIENTED_EDGE('',*,*,#7487,.T.);
#10473=ORIENTED_EDGE('',*,*,#7483,.F.);
#10474=ORIENTED_EDGE('',*,*,#7488,.F.);
#10475=ORIENTED_EDGE('',*,*,#7489,.T.);
#10476=ORIENTED_EDGE('',*,*,#7490,.T.);
#10477=ORIENTED_EDGE('',*,*,#7486,.F.);
#10478=ORIENTED_EDGE('',*,*,#7491,.F.);
#10479=ORIENTED_EDGE('',*,*,#7492,.T.);
#10480=ORIENTED_EDGE('',*,*,#7493,.T.);
#10481=ORIENTED_EDGE('',*,*,#7489,.F.);
#10482=ORIENTED_EDGE('',*,*,#7494,.F.);
#10483=ORIENTED_EDGE('',*,*,#7495,.F.);
#10484=ORIENTED_EDGE('',*,*,#7496,.F.);
#10485=ORIENTED_EDGE('',*,*,#7497,.F.);
#10486=ORIENTED_EDGE('',*,*,#7498,.T.);
#10487=ORIENTED_EDGE('',*,*,#7499,.T.);
#10488=ORIENTED_EDGE('',*,*,#7500,.T.);
#10489=ORIENTED_EDGE('',*,*,#7501,.T.);
#10490=ORIENTED_EDGE('',*,*,#7502,.T.);
#10491=ORIENTED_EDGE('',*,*,#7503,.F.);
#10492=ORIENTED_EDGE('',*,*,#7502,.F.);
#10493=ORIENTED_EDGE('',*,*,#7504,.T.);
#10494=ORIENTED_EDGE('',*,*,#7505,.T.);
#10495=ORIENTED_EDGE('',*,*,#7506,.T.);
#10496=ORIENTED_EDGE('',*,*,#7507,.T.);
#10497=ORIENTED_EDGE('',*,*,#7499,.F.);
#10498=ORIENTED_EDGE('',*,*,#7508,.T.);
#10499=ORIENTED_EDGE('',*,*,#7509,.T.);
#10500=ORIENTED_EDGE('',*,*,#7510,.T.);
#10501=ORIENTED_EDGE('',*,*,#7506,.F.);
#10502=ORIENTED_EDGE('',*,*,#7511,.T.);
#10503=ORIENTED_EDGE('',*,*,#7512,.T.);
#10504=ORIENTED_EDGE('',*,*,#7513,.T.);
#10505=ORIENTED_EDGE('',*,*,#7509,.F.);
#10506=ORIENTED_EDGE('',*,*,#7514,.T.);
#10507=ORIENTED_EDGE('',*,*,#7515,.T.);
#10508=ORIENTED_EDGE('',*,*,#7516,.T.);
#10509=ORIENTED_EDGE('',*,*,#7512,.F.);
#10510=ORIENTED_EDGE('',*,*,#7517,.T.);
#10511=ORIENTED_EDGE('',*,*,#7518,.T.);
#10512=ORIENTED_EDGE('',*,*,#7519,.T.);
#10513=ORIENTED_EDGE('',*,*,#7515,.F.);
#10514=ORIENTED_EDGE('',*,*,#7520,.T.);
#10515=ORIENTED_EDGE('',*,*,#7521,.F.);
#10516=ORIENTED_EDGE('',*,*,#7522,.T.);
#10517=ORIENTED_EDGE('',*,*,#7523,.F.);
#10518=ORIENTED_EDGE('',*,*,#7524,.T.);
#10519=ORIENTED_EDGE('',*,*,#7525,.T.);
#10520=ORIENTED_EDGE('',*,*,#7526,.T.);
#10521=ORIENTED_EDGE('',*,*,#7527,.F.);
#10522=ORIENTED_EDGE('',*,*,#7528,.F.);
#10523=ORIENTED_EDGE('',*,*,#7529,.T.);
#10524=ORIENTED_EDGE('',*,*,#7530,.T.);
#10525=ORIENTED_EDGE('',*,*,#7525,.F.);
#10526=ORIENTED_EDGE('',*,*,#7531,.F.);
#10527=ORIENTED_EDGE('',*,*,#7532,.T.);
#10528=ORIENTED_EDGE('',*,*,#7533,.T.);
#10529=ORIENTED_EDGE('',*,*,#7529,.F.);
#10530=ORIENTED_EDGE('',*,*,#7534,.F.);
#10531=ORIENTED_EDGE('',*,*,#7535,.T.);
#10532=ORIENTED_EDGE('',*,*,#7536,.T.);
#10533=ORIENTED_EDGE('',*,*,#7532,.F.);
#10534=ORIENTED_EDGE('',*,*,#7537,.F.);
#10535=ORIENTED_EDGE('',*,*,#7538,.T.);
#10536=ORIENTED_EDGE('',*,*,#7539,.T.);
#10537=ORIENTED_EDGE('',*,*,#7535,.F.);
#10538=ORIENTED_EDGE('',*,*,#7540,.F.);
#10539=ORIENTED_EDGE('',*,*,#7541,.T.);
#10540=ORIENTED_EDGE('',*,*,#7542,.T.);
#10541=ORIENTED_EDGE('',*,*,#7538,.F.);
#10542=ORIENTED_EDGE('',*,*,#7543,.F.);
#10543=ORIENTED_EDGE('',*,*,#7544,.F.);
#10544=ORIENTED_EDGE('',*,*,#7545,.F.);
#10545=ORIENTED_EDGE('',*,*,#7546,.F.);
#10546=ORIENTED_EDGE('',*,*,#7547,.T.);
#10547=ORIENTED_EDGE('',*,*,#7548,.T.);
#10548=ORIENTED_EDGE('',*,*,#7549,.T.);
#10549=ORIENTED_EDGE('',*,*,#7550,.T.);
#10550=ORIENTED_EDGE('',*,*,#7551,.T.);
#10551=ORIENTED_EDGE('',*,*,#7552,.F.);
#10552=ORIENTED_EDGE('',*,*,#7551,.F.);
#10553=ORIENTED_EDGE('',*,*,#7553,.T.);
#10554=ORIENTED_EDGE('',*,*,#7554,.T.);
#10555=ORIENTED_EDGE('',*,*,#7555,.T.);
#10556=ORIENTED_EDGE('',*,*,#7556,.T.);
#10557=ORIENTED_EDGE('',*,*,#7548,.F.);
#10558=ORIENTED_EDGE('',*,*,#7557,.T.);
#10559=ORIENTED_EDGE('',*,*,#7558,.T.);
#10560=ORIENTED_EDGE('',*,*,#7559,.T.);
#10561=ORIENTED_EDGE('',*,*,#7555,.F.);
#10562=ORIENTED_EDGE('',*,*,#7560,.T.);
#10563=ORIENTED_EDGE('',*,*,#7561,.T.);
#10564=ORIENTED_EDGE('',*,*,#7562,.T.);
#10565=ORIENTED_EDGE('',*,*,#7558,.F.);
#10566=ORIENTED_EDGE('',*,*,#7563,.T.);
#10567=ORIENTED_EDGE('',*,*,#7564,.T.);
#10568=ORIENTED_EDGE('',*,*,#7565,.T.);
#10569=ORIENTED_EDGE('',*,*,#7561,.F.);
#10570=ORIENTED_EDGE('',*,*,#7566,.T.);
#10571=ORIENTED_EDGE('',*,*,#7567,.T.);
#10572=ORIENTED_EDGE('',*,*,#7568,.T.);
#10573=ORIENTED_EDGE('',*,*,#7564,.F.);
#10574=ORIENTED_EDGE('',*,*,#7569,.T.);
#10575=ORIENTED_EDGE('',*,*,#7570,.F.);
#10576=ORIENTED_EDGE('',*,*,#7571,.T.);
#10577=ORIENTED_EDGE('',*,*,#7572,.F.);
#10578=ORIENTED_EDGE('',*,*,#7573,.T.);
#10579=ORIENTED_EDGE('',*,*,#7574,.T.);
#10580=ORIENTED_EDGE('',*,*,#7575,.T.);
#10581=ORIENTED_EDGE('',*,*,#7576,.F.);
#10582=ORIENTED_EDGE('',*,*,#7577,.F.);
#10583=ORIENTED_EDGE('',*,*,#7578,.T.);
#10584=ORIENTED_EDGE('',*,*,#7579,.T.);
#10585=ORIENTED_EDGE('',*,*,#7574,.F.);
#10586=ORIENTED_EDGE('',*,*,#7580,.F.);
#10587=ORIENTED_EDGE('',*,*,#7581,.T.);
#10588=ORIENTED_EDGE('',*,*,#7582,.T.);
#10589=ORIENTED_EDGE('',*,*,#7578,.F.);
#10590=ORIENTED_EDGE('',*,*,#7583,.F.);
#10591=ORIENTED_EDGE('',*,*,#7584,.T.);
#10592=ORIENTED_EDGE('',*,*,#7585,.T.);
#10593=ORIENTED_EDGE('',*,*,#7581,.F.);
#10594=ORIENTED_EDGE('',*,*,#7586,.F.);
#10595=ORIENTED_EDGE('',*,*,#7587,.T.);
#10596=ORIENTED_EDGE('',*,*,#7588,.T.);
#10597=ORIENTED_EDGE('',*,*,#7584,.F.);
#10598=ORIENTED_EDGE('',*,*,#7589,.F.);
#10599=ORIENTED_EDGE('',*,*,#7590,.T.);
#10600=ORIENTED_EDGE('',*,*,#7591,.T.);
#10601=ORIENTED_EDGE('',*,*,#7587,.F.);
#10602=ORIENTED_EDGE('',*,*,#7592,.F.);
#10603=ORIENTED_EDGE('',*,*,#7593,.F.);
#10604=ORIENTED_EDGE('',*,*,#7594,.F.);
#10605=ORIENTED_EDGE('',*,*,#7595,.F.);
#10606=ORIENTED_EDGE('',*,*,#7596,.T.);
#10607=ORIENTED_EDGE('',*,*,#7597,.T.);
#10608=ORIENTED_EDGE('',*,*,#7598,.T.);
#10609=ORIENTED_EDGE('',*,*,#7599,.T.);
#10610=ORIENTED_EDGE('',*,*,#7600,.T.);
#10611=ORIENTED_EDGE('',*,*,#7601,.F.);
#10612=ORIENTED_EDGE('',*,*,#7600,.F.);
#10613=ORIENTED_EDGE('',*,*,#7602,.T.);
#10614=ORIENTED_EDGE('',*,*,#7603,.T.);
#10615=ORIENTED_EDGE('',*,*,#7604,.T.);
#10616=ORIENTED_EDGE('',*,*,#7605,.T.);
#10617=ORIENTED_EDGE('',*,*,#7597,.F.);
#10618=ORIENTED_EDGE('',*,*,#7606,.T.);
#10619=ORIENTED_EDGE('',*,*,#7607,.T.);
#10620=ORIENTED_EDGE('',*,*,#7608,.T.);
#10621=ORIENTED_EDGE('',*,*,#7604,.F.);
#10622=ORIENTED_EDGE('',*,*,#7609,.T.);
#10623=ORIENTED_EDGE('',*,*,#7610,.T.);
#10624=ORIENTED_EDGE('',*,*,#7611,.T.);
#10625=ORIENTED_EDGE('',*,*,#7607,.F.);
#10626=ORIENTED_EDGE('',*,*,#7612,.T.);
#10627=ORIENTED_EDGE('',*,*,#7613,.T.);
#10628=ORIENTED_EDGE('',*,*,#7614,.T.);
#10629=ORIENTED_EDGE('',*,*,#7610,.F.);
#10630=ORIENTED_EDGE('',*,*,#7615,.T.);
#10631=ORIENTED_EDGE('',*,*,#7616,.T.);
#10632=ORIENTED_EDGE('',*,*,#7617,.T.);
#10633=ORIENTED_EDGE('',*,*,#7613,.F.);
#10634=ORIENTED_EDGE('',*,*,#7618,.T.);
#10635=ORIENTED_EDGE('',*,*,#7619,.F.);
#10636=ORIENTED_EDGE('',*,*,#7620,.T.);
#10637=ORIENTED_EDGE('',*,*,#7621,.F.);
#10638=ORIENTED_EDGE('',*,*,#7622,.T.);
#10639=ORIENTED_EDGE('',*,*,#7623,.T.);
#10640=ORIENTED_EDGE('',*,*,#7624,.T.);
#10641=ORIENTED_EDGE('',*,*,#7625,.F.);
#10642=ORIENTED_EDGE('',*,*,#7626,.F.);
#10643=ORIENTED_EDGE('',*,*,#7627,.T.);
#10644=ORIENTED_EDGE('',*,*,#7628,.T.);
#10645=ORIENTED_EDGE('',*,*,#7623,.F.);
#10646=ORIENTED_EDGE('',*,*,#7629,.F.);
#10647=ORIENTED_EDGE('',*,*,#7630,.T.);
#10648=ORIENTED_EDGE('',*,*,#7631,.T.);
#10649=ORIENTED_EDGE('',*,*,#7627,.F.);
#10650=ORIENTED_EDGE('',*,*,#7632,.F.);
#10651=ORIENTED_EDGE('',*,*,#7633,.T.);
#10652=ORIENTED_EDGE('',*,*,#7634,.T.);
#10653=ORIENTED_EDGE('',*,*,#7630,.F.);
#10654=ORIENTED_EDGE('',*,*,#7635,.F.);
#10655=ORIENTED_EDGE('',*,*,#7636,.T.);
#10656=ORIENTED_EDGE('',*,*,#7637,.T.);
#10657=ORIENTED_EDGE('',*,*,#7633,.F.);
#10658=ORIENTED_EDGE('',*,*,#7638,.F.);
#10659=ORIENTED_EDGE('',*,*,#7639,.T.);
#10660=ORIENTED_EDGE('',*,*,#7640,.T.);
#10661=ORIENTED_EDGE('',*,*,#7636,.F.);
#10662=ORIENTED_EDGE('',*,*,#7641,.F.);
#10663=ORIENTED_EDGE('',*,*,#7642,.F.);
#10664=ORIENTED_EDGE('',*,*,#7643,.F.);
#10665=ORIENTED_EDGE('',*,*,#7644,.F.);
#10666=ORIENTED_EDGE('',*,*,#7645,.T.);
#10667=ORIENTED_EDGE('',*,*,#7646,.T.);
#10668=ORIENTED_EDGE('',*,*,#7647,.T.);
#10669=ORIENTED_EDGE('',*,*,#7648,.T.);
#10670=ORIENTED_EDGE('',*,*,#7649,.T.);
#10671=ORIENTED_EDGE('',*,*,#7650,.T.);
#10672=ORIENTED_EDGE('',*,*,#7651,.T.);
#10673=ORIENTED_EDGE('',*,*,#7650,.F.);
#10674=ORIENTED_EDGE('',*,*,#7652,.T.);
#10675=ORIENTED_EDGE('',*,*,#7653,.T.);
#10676=ORIENTED_EDGE('',*,*,#7654,.T.);
#10677=ORIENTED_EDGE('',*,*,#7646,.F.);
#10678=ORIENTED_EDGE('',*,*,#7655,.T.);
#10679=ORIENTED_EDGE('',*,*,#7656,.T.);
#10680=ORIENTED_EDGE('',*,*,#7657,.T.);
#10681=ORIENTED_EDGE('',*,*,#7653,.F.);
#10682=ORIENTED_EDGE('',*,*,#7658,.T.);
#10683=ORIENTED_EDGE('',*,*,#7659,.F.);
#10684=ORIENTED_EDGE('',*,*,#7660,.T.);
#10685=ORIENTED_EDGE('',*,*,#7661,.F.);
#10686=ORIENTED_EDGE('',*,*,#7662,.T.);
#10687=ORIENTED_EDGE('',*,*,#7663,.T.);
#10688=ORIENTED_EDGE('',*,*,#7664,.T.);
#10689=ORIENTED_EDGE('',*,*,#7665,.F.);
#10690=ORIENTED_EDGE('',*,*,#7666,.F.);
#10691=ORIENTED_EDGE('',*,*,#7667,.T.);
#10692=ORIENTED_EDGE('',*,*,#7668,.T.);
#10693=ORIENTED_EDGE('',*,*,#7663,.F.);
#10694=ORIENTED_EDGE('',*,*,#7669,.F.);
#10695=ORIENTED_EDGE('',*,*,#7670,.T.);
#10696=ORIENTED_EDGE('',*,*,#7671,.T.);
#10697=ORIENTED_EDGE('',*,*,#7667,.F.);
#10698=ORIENTED_EDGE('',*,*,#7672,.F.);
#10699=ORIENTED_EDGE('',*,*,#7673,.T.);
#10700=ORIENTED_EDGE('',*,*,#7674,.T.);
#10701=ORIENTED_EDGE('',*,*,#7670,.F.);
#10702=ORIENTED_EDGE('',*,*,#7675,.F.);
#10703=ORIENTED_EDGE('',*,*,#7676,.F.);
#10704=ORIENTED_EDGE('',*,*,#7677,.F.);
#10705=ORIENTED_EDGE('',*,*,#7678,.F.);
#10706=ORIENTED_EDGE('',*,*,#7679,.T.);
#10707=ORIENTED_EDGE('',*,*,#7680,.T.);
#10708=ORIENTED_EDGE('',*,*,#7681,.T.);
#10709=ORIENTED_EDGE('',*,*,#7682,.T.);
#10710=ORIENTED_EDGE('',*,*,#7683,.T.);
#10711=ORIENTED_EDGE('',*,*,#7684,.T.);
#10712=ORIENTED_EDGE('',*,*,#7685,.T.);
#10713=ORIENTED_EDGE('',*,*,#7684,.F.);
#10714=ORIENTED_EDGE('',*,*,#7686,.T.);
#10715=ORIENTED_EDGE('',*,*,#7687,.T.);
#10716=ORIENTED_EDGE('',*,*,#7688,.T.);
#10717=ORIENTED_EDGE('',*,*,#7680,.F.);
#10718=ORIENTED_EDGE('',*,*,#7689,.T.);
#10719=ORIENTED_EDGE('',*,*,#7690,.T.);
#10720=ORIENTED_EDGE('',*,*,#7691,.T.);
#10721=ORIENTED_EDGE('',*,*,#7687,.F.);
#10722=ORIENTED_EDGE('',*,*,#7692,.T.);
#10723=ORIENTED_EDGE('',*,*,#7693,.F.);
#10724=ORIENTED_EDGE('',*,*,#7694,.T.);
#10725=ORIENTED_EDGE('',*,*,#7695,.F.);
#10726=ORIENTED_EDGE('',*,*,#7696,.T.);
#10727=ORIENTED_EDGE('',*,*,#7697,.T.);
#10728=ORIENTED_EDGE('',*,*,#7698,.T.);
#10729=ORIENTED_EDGE('',*,*,#7699,.F.);
#10730=ORIENTED_EDGE('',*,*,#7700,.F.);
#10731=ORIENTED_EDGE('',*,*,#7701,.T.);
#10732=ORIENTED_EDGE('',*,*,#7702,.T.);
#10733=ORIENTED_EDGE('',*,*,#7697,.F.);
#10734=ORIENTED_EDGE('',*,*,#7703,.F.);
#10735=ORIENTED_EDGE('',*,*,#7704,.T.);
#10736=ORIENTED_EDGE('',*,*,#7705,.T.);
#10737=ORIENTED_EDGE('',*,*,#7701,.F.);
#10738=ORIENTED_EDGE('',*,*,#7706,.F.);
#10739=ORIENTED_EDGE('',*,*,#7707,.T.);
#10740=ORIENTED_EDGE('',*,*,#7708,.T.);
#10741=ORIENTED_EDGE('',*,*,#7704,.F.);
#10742=ORIENTED_EDGE('',*,*,#7709,.F.);
#10743=ORIENTED_EDGE('',*,*,#7710,.F.);
#10744=ORIENTED_EDGE('',*,*,#7711,.F.);
#10745=ORIENTED_EDGE('',*,*,#7712,.F.);
#10746=ORIENTED_EDGE('',*,*,#7713,.T.);
#10747=ORIENTED_EDGE('',*,*,#7714,.T.);
#10748=ORIENTED_EDGE('',*,*,#7715,.T.);
#10749=ORIENTED_EDGE('',*,*,#7716,.T.);
#10750=ORIENTED_EDGE('',*,*,#7717,.T.);
#10751=ORIENTED_EDGE('',*,*,#7718,.T.);
#10752=ORIENTED_EDGE('',*,*,#7719,.T.);
#10753=ORIENTED_EDGE('',*,*,#7718,.F.);
#10754=ORIENTED_EDGE('',*,*,#7720,.T.);
#10755=ORIENTED_EDGE('',*,*,#7721,.T.);
#10756=ORIENTED_EDGE('',*,*,#7722,.T.);
#10757=ORIENTED_EDGE('',*,*,#7714,.F.);
#10758=ORIENTED_EDGE('',*,*,#7723,.T.);
#10759=ORIENTED_EDGE('',*,*,#7724,.T.);
#10760=ORIENTED_EDGE('',*,*,#7725,.T.);
#10761=ORIENTED_EDGE('',*,*,#7721,.F.);
#10762=ORIENTED_EDGE('',*,*,#7726,.T.);
#10763=ORIENTED_EDGE('',*,*,#7727,.F.);
#10764=ORIENTED_EDGE('',*,*,#7728,.T.);
#10765=ORIENTED_EDGE('',*,*,#7729,.F.);
#10766=ORIENTED_EDGE('',*,*,#7730,.T.);
#10767=ORIENTED_EDGE('',*,*,#7731,.T.);
#10768=ORIENTED_EDGE('',*,*,#7732,.T.);
#10769=ORIENTED_EDGE('',*,*,#7733,.F.);
#10770=ORIENTED_EDGE('',*,*,#7734,.F.);
#10771=ORIENTED_EDGE('',*,*,#7735,.T.);
#10772=ORIENTED_EDGE('',*,*,#7736,.T.);
#10773=ORIENTED_EDGE('',*,*,#7731,.F.);
#10774=ORIENTED_EDGE('',*,*,#7737,.F.);
#10775=ORIENTED_EDGE('',*,*,#7738,.T.);
#10776=ORIENTED_EDGE('',*,*,#7739,.T.);
#10777=ORIENTED_EDGE('',*,*,#7735,.F.);
#10778=ORIENTED_EDGE('',*,*,#7740,.F.);
#10779=ORIENTED_EDGE('',*,*,#7741,.T.);
#10780=ORIENTED_EDGE('',*,*,#7742,.T.);
#10781=ORIENTED_EDGE('',*,*,#7738,.F.);
#10782=ORIENTED_EDGE('',*,*,#7743,.F.);
#10783=ORIENTED_EDGE('',*,*,#7744,.F.);
#10784=ORIENTED_EDGE('',*,*,#7745,.F.);
#10785=ORIENTED_EDGE('',*,*,#7746,.F.);
#10786=ORIENTED_EDGE('',*,*,#7747,.T.);
#10787=ORIENTED_EDGE('',*,*,#7748,.T.);
#10788=ORIENTED_EDGE('',*,*,#7749,.T.);
#10789=ORIENTED_EDGE('',*,*,#7750,.T.);
#10790=ORIENTED_EDGE('',*,*,#7751,.T.);
#10791=ORIENTED_EDGE('',*,*,#7752,.T.);
#10792=ORIENTED_EDGE('',*,*,#7753,.T.);
#10793=ORIENTED_EDGE('',*,*,#7752,.F.);
#10794=ORIENTED_EDGE('',*,*,#7754,.T.);
#10795=ORIENTED_EDGE('',*,*,#7755,.T.);
#10796=ORIENTED_EDGE('',*,*,#7756,.T.);
#10797=ORIENTED_EDGE('',*,*,#7748,.F.);
#10798=ORIENTED_EDGE('',*,*,#7757,.T.);
#10799=ORIENTED_EDGE('',*,*,#7758,.T.);
#10800=ORIENTED_EDGE('',*,*,#7759,.T.);
#10801=ORIENTED_EDGE('',*,*,#7755,.F.);
#10802=ORIENTED_EDGE('',*,*,#7760,.T.);
#10803=ORIENTED_EDGE('',*,*,#7761,.F.);
#10804=ORIENTED_EDGE('',*,*,#7762,.T.);
#10805=ORIENTED_EDGE('',*,*,#7763,.F.);
#10806=ORIENTED_EDGE('',*,*,#7764,.T.);
#10807=ORIENTED_EDGE('',*,*,#7765,.T.);
#10808=ORIENTED_EDGE('',*,*,#7766,.T.);
#10809=ORIENTED_EDGE('',*,*,#7767,.F.);
#10810=ORIENTED_EDGE('',*,*,#7768,.F.);
#10811=ORIENTED_EDGE('',*,*,#7769,.T.);
#10812=ORIENTED_EDGE('',*,*,#7770,.T.);
#10813=ORIENTED_EDGE('',*,*,#7765,.F.);
#10814=ORIENTED_EDGE('',*,*,#7771,.F.);
#10815=ORIENTED_EDGE('',*,*,#7772,.T.);
#10816=ORIENTED_EDGE('',*,*,#7773,.T.);
#10817=ORIENTED_EDGE('',*,*,#7769,.F.);
#10818=ORIENTED_EDGE('',*,*,#7774,.F.);
#10819=ORIENTED_EDGE('',*,*,#7775,.T.);
#10820=ORIENTED_EDGE('',*,*,#7776,.T.);
#10821=ORIENTED_EDGE('',*,*,#7772,.F.);
#10822=ORIENTED_EDGE('',*,*,#7777,.F.);
#10823=ORIENTED_EDGE('',*,*,#7778,.F.);
#10824=ORIENTED_EDGE('',*,*,#7779,.F.);
#10825=ORIENTED_EDGE('',*,*,#7780,.F.);
#10826=ORIENTED_EDGE('',*,*,#7781,.T.);
#10827=ORIENTED_EDGE('',*,*,#7750,.F.);
#10828=ORIENTED_EDGE('',*,*,#7782,.T.);
#10829=ORIENTED_EDGE('',*,*,#7767,.T.);
#10830=ORIENTED_EDGE('',*,*,#7783,.T.);
#10831=ORIENTED_EDGE('',*,*,#7778,.T.);
#10832=ORIENTED_EDGE('',*,*,#7784,.T.);
#10833=ORIENTED_EDGE('',*,*,#7775,.F.);
#10834=ORIENTED_EDGE('',*,*,#7785,.F.);
#10835=ORIENTED_EDGE('',*,*,#7783,.F.);
#10836=ORIENTED_EDGE('',*,*,#7766,.F.);
#10837=ORIENTED_EDGE('',*,*,#7770,.F.);
#10838=ORIENTED_EDGE('',*,*,#7773,.F.);
#10839=ORIENTED_EDGE('',*,*,#7776,.F.);
#10840=ORIENTED_EDGE('',*,*,#7784,.F.);
#10841=ORIENTED_EDGE('',*,*,#7781,.F.);
#10842=ORIENTED_EDGE('',*,*,#7786,.F.);
#10843=ORIENTED_EDGE('',*,*,#7762,.F.);
#10844=ORIENTED_EDGE('',*,*,#7787,.F.);
#10845=ORIENTED_EDGE('',*,*,#7760,.F.);
#10846=ORIENTED_EDGE('',*,*,#7757,.F.);
#10847=ORIENTED_EDGE('',*,*,#7754,.F.);
#10848=ORIENTED_EDGE('',*,*,#7751,.F.);
#10849=ORIENTED_EDGE('',*,*,#7782,.F.);
#10850=ORIENTED_EDGE('',*,*,#7749,.F.);
#10851=ORIENTED_EDGE('',*,*,#7756,.F.);
#10852=ORIENTED_EDGE('',*,*,#7759,.F.);
#10853=ORIENTED_EDGE('',*,*,#7788,.F.);
#10854=ORIENTED_EDGE('',*,*,#7764,.F.);
#10855=ORIENTED_EDGE('',*,*,#7789,.F.);
#10856=ORIENTED_EDGE('',*,*,#7779,.T.);
#10857=ORIENTED_EDGE('',*,*,#7785,.T.);
#10858=ORIENTED_EDGE('',*,*,#7777,.T.);
#10859=ORIENTED_EDGE('',*,*,#7774,.T.);
#10860=ORIENTED_EDGE('',*,*,#7771,.T.);
#10861=ORIENTED_EDGE('',*,*,#7768,.T.);
#10862=ORIENTED_EDGE('',*,*,#7761,.T.);
#10863=ORIENTED_EDGE('',*,*,#7788,.T.);
#10864=ORIENTED_EDGE('',*,*,#7758,.F.);
#10865=ORIENTED_EDGE('',*,*,#7787,.T.);
#10866=ORIENTED_EDGE('',*,*,#7716,.F.);
#10867=ORIENTED_EDGE('',*,*,#7790,.T.);
#10868=ORIENTED_EDGE('',*,*,#7733,.T.);
#10869=ORIENTED_EDGE('',*,*,#7791,.T.);
#10870=ORIENTED_EDGE('',*,*,#7744,.T.);
#10871=ORIENTED_EDGE('',*,*,#7792,.T.);
#10872=ORIENTED_EDGE('',*,*,#7741,.F.);
#10873=ORIENTED_EDGE('',*,*,#7793,.F.);
#10874=ORIENTED_EDGE('',*,*,#7791,.F.);
#10875=ORIENTED_EDGE('',*,*,#7732,.F.);
#10876=ORIENTED_EDGE('',*,*,#7736,.F.);
#10877=ORIENTED_EDGE('',*,*,#7739,.F.);
#10878=ORIENTED_EDGE('',*,*,#7742,.F.);
#10879=ORIENTED_EDGE('',*,*,#7792,.F.);
#10880=ORIENTED_EDGE('',*,*,#7747,.F.);
#10881=ORIENTED_EDGE('',*,*,#7794,.F.);
#10882=ORIENTED_EDGE('',*,*,#7728,.F.);
#10883=ORIENTED_EDGE('',*,*,#7795,.F.);
#10884=ORIENTED_EDGE('',*,*,#7726,.F.);
#10885=ORIENTED_EDGE('',*,*,#7723,.F.);
#10886=ORIENTED_EDGE('',*,*,#7720,.F.);
#10887=ORIENTED_EDGE('',*,*,#7717,.F.);
#10888=ORIENTED_EDGE('',*,*,#7790,.F.);
#10889=ORIENTED_EDGE('',*,*,#7715,.F.);
#10890=ORIENTED_EDGE('',*,*,#7722,.F.);
#10891=ORIENTED_EDGE('',*,*,#7725,.F.);
#10892=ORIENTED_EDGE('',*,*,#7796,.F.);
#10893=ORIENTED_EDGE('',*,*,#7730,.F.);
#10894=ORIENTED_EDGE('',*,*,#7797,.F.);
#10895=ORIENTED_EDGE('',*,*,#7745,.T.);
#10896=ORIENTED_EDGE('',*,*,#7793,.T.);
#10897=ORIENTED_EDGE('',*,*,#7743,.T.);
#10898=ORIENTED_EDGE('',*,*,#7740,.T.);
#10899=ORIENTED_EDGE('',*,*,#7737,.T.);
#10900=ORIENTED_EDGE('',*,*,#7734,.T.);
#10901=ORIENTED_EDGE('',*,*,#7727,.T.);
#10902=ORIENTED_EDGE('',*,*,#7796,.T.);
#10903=ORIENTED_EDGE('',*,*,#7724,.F.);
#10904=ORIENTED_EDGE('',*,*,#7795,.T.);
#10905=ORIENTED_EDGE('',*,*,#7682,.F.);
#10906=ORIENTED_EDGE('',*,*,#7798,.T.);
#10907=ORIENTED_EDGE('',*,*,#7699,.T.);
#10908=ORIENTED_EDGE('',*,*,#7799,.T.);
#10909=ORIENTED_EDGE('',*,*,#7710,.T.);
#10910=ORIENTED_EDGE('',*,*,#7800,.T.);
#10911=ORIENTED_EDGE('',*,*,#7707,.F.);
#10912=ORIENTED_EDGE('',*,*,#7801,.F.);
#10913=ORIENTED_EDGE('',*,*,#7799,.F.);
#10914=ORIENTED_EDGE('',*,*,#7698,.F.);
#10915=ORIENTED_EDGE('',*,*,#7702,.F.);
#10916=ORIENTED_EDGE('',*,*,#7705,.F.);
#10917=ORIENTED_EDGE('',*,*,#7708,.F.);
#10918=ORIENTED_EDGE('',*,*,#7800,.F.);
#10919=ORIENTED_EDGE('',*,*,#7713,.F.);
#10920=ORIENTED_EDGE('',*,*,#7802,.F.);
#10921=ORIENTED_EDGE('',*,*,#7694,.F.);
#10922=ORIENTED_EDGE('',*,*,#7803,.F.);
#10923=ORIENTED_EDGE('',*,*,#7692,.F.);
#10924=ORIENTED_EDGE('',*,*,#7689,.F.);
#10925=ORIENTED_EDGE('',*,*,#7686,.F.);
#10926=ORIENTED_EDGE('',*,*,#7683,.F.);
#10927=ORIENTED_EDGE('',*,*,#7798,.F.);
#10928=ORIENTED_EDGE('',*,*,#7681,.F.);
#10929=ORIENTED_EDGE('',*,*,#7688,.F.);
#10930=ORIENTED_EDGE('',*,*,#7691,.F.);
#10931=ORIENTED_EDGE('',*,*,#7804,.F.);
#10932=ORIENTED_EDGE('',*,*,#7696,.F.);
#10933=ORIENTED_EDGE('',*,*,#7805,.F.);
#10934=ORIENTED_EDGE('',*,*,#7711,.T.);
#10935=ORIENTED_EDGE('',*,*,#7801,.T.);
#10936=ORIENTED_EDGE('',*,*,#7709,.T.);
#10937=ORIENTED_EDGE('',*,*,#7706,.T.);
#10938=ORIENTED_EDGE('',*,*,#7703,.T.);
#10939=ORIENTED_EDGE('',*,*,#7700,.T.);
#10940=ORIENTED_EDGE('',*,*,#7693,.T.);
#10941=ORIENTED_EDGE('',*,*,#7804,.T.);
#10942=ORIENTED_EDGE('',*,*,#7690,.F.);
#10943=ORIENTED_EDGE('',*,*,#7803,.T.);
#10944=ORIENTED_EDGE('',*,*,#7648,.F.);
#10945=ORIENTED_EDGE('',*,*,#7806,.T.);
#10946=ORIENTED_EDGE('',*,*,#7665,.T.);
#10947=ORIENTED_EDGE('',*,*,#7807,.T.);
#10948=ORIENTED_EDGE('',*,*,#7676,.T.);
#10949=ORIENTED_EDGE('',*,*,#7808,.T.);
#10950=ORIENTED_EDGE('',*,*,#7673,.F.);
#10951=ORIENTED_EDGE('',*,*,#7809,.F.);
#10952=ORIENTED_EDGE('',*,*,#7807,.F.);
#10953=ORIENTED_EDGE('',*,*,#7664,.F.);
#10954=ORIENTED_EDGE('',*,*,#7668,.F.);
#10955=ORIENTED_EDGE('',*,*,#7671,.F.);
#10956=ORIENTED_EDGE('',*,*,#7674,.F.);
#10957=ORIENTED_EDGE('',*,*,#7808,.F.);
#10958=ORIENTED_EDGE('',*,*,#7679,.F.);
#10959=ORIENTED_EDGE('',*,*,#7810,.F.);
#10960=ORIENTED_EDGE('',*,*,#7660,.F.);
#10961=ORIENTED_EDGE('',*,*,#7811,.F.);
#10962=ORIENTED_EDGE('',*,*,#7658,.F.);
#10963=ORIENTED_EDGE('',*,*,#7655,.F.);
#10964=ORIENTED_EDGE('',*,*,#7652,.F.);
#10965=ORIENTED_EDGE('',*,*,#7649,.F.);
#10966=ORIENTED_EDGE('',*,*,#7806,.F.);
#10967=ORIENTED_EDGE('',*,*,#7647,.F.);
#10968=ORIENTED_EDGE('',*,*,#7654,.F.);
#10969=ORIENTED_EDGE('',*,*,#7657,.F.);
#10970=ORIENTED_EDGE('',*,*,#7812,.F.);
#10971=ORIENTED_EDGE('',*,*,#7662,.F.);
#10972=ORIENTED_EDGE('',*,*,#7813,.F.);
#10973=ORIENTED_EDGE('',*,*,#7677,.T.);
#10974=ORIENTED_EDGE('',*,*,#7809,.T.);
#10975=ORIENTED_EDGE('',*,*,#7675,.T.);
#10976=ORIENTED_EDGE('',*,*,#7672,.T.);
#10977=ORIENTED_EDGE('',*,*,#7669,.T.);
#10978=ORIENTED_EDGE('',*,*,#7666,.T.);
#10979=ORIENTED_EDGE('',*,*,#7659,.T.);
#10980=ORIENTED_EDGE('',*,*,#7812,.T.);
#10981=ORIENTED_EDGE('',*,*,#7656,.F.);
#10982=ORIENTED_EDGE('',*,*,#7811,.T.);
#10983=ORIENTED_EDGE('',*,*,#7651,.F.);
#10984=ORIENTED_EDGE('',*,*,#7685,.F.);
#10985=ORIENTED_EDGE('',*,*,#7753,.F.);
#10986=ORIENTED_EDGE('',*,*,#7719,.F.);
#10987=ORIENTED_EDGE('',*,*,#7599,.F.);
#10988=ORIENTED_EDGE('',*,*,#7814,.T.);
#10989=ORIENTED_EDGE('',*,*,#7625,.T.);
#10990=ORIENTED_EDGE('',*,*,#7815,.T.);
#10991=ORIENTED_EDGE('',*,*,#7602,.F.);
#10992=ORIENTED_EDGE('',*,*,#7642,.T.);
#10993=ORIENTED_EDGE('',*,*,#7816,.T.);
#10994=ORIENTED_EDGE('',*,*,#7639,.F.);
#10995=ORIENTED_EDGE('',*,*,#7817,.F.);
#10996=ORIENTED_EDGE('',*,*,#7815,.F.);
#10997=ORIENTED_EDGE('',*,*,#7624,.F.);
#10998=ORIENTED_EDGE('',*,*,#7628,.F.);
#10999=ORIENTED_EDGE('',*,*,#7631,.F.);
#11000=ORIENTED_EDGE('',*,*,#7634,.F.);
#11001=ORIENTED_EDGE('',*,*,#7637,.F.);
#11002=ORIENTED_EDGE('',*,*,#7640,.F.);
#11003=ORIENTED_EDGE('',*,*,#7816,.F.);
#11004=ORIENTED_EDGE('',*,*,#7645,.F.);
#11005=ORIENTED_EDGE('',*,*,#7818,.F.);
#11006=ORIENTED_EDGE('',*,*,#7620,.F.);
#11007=ORIENTED_EDGE('',*,*,#7819,.F.);
#11008=ORIENTED_EDGE('',*,*,#7618,.F.);
#11009=ORIENTED_EDGE('',*,*,#7615,.F.);
#11010=ORIENTED_EDGE('',*,*,#7612,.F.);
#11011=ORIENTED_EDGE('',*,*,#7609,.F.);
#11012=ORIENTED_EDGE('',*,*,#7606,.F.);
#11013=ORIENTED_EDGE('',*,*,#7603,.F.);
#11014=ORIENTED_EDGE('',*,*,#7814,.F.);
#11015=ORIENTED_EDGE('',*,*,#7598,.F.);
#11016=ORIENTED_EDGE('',*,*,#7605,.F.);
#11017=ORIENTED_EDGE('',*,*,#7608,.F.);
#11018=ORIENTED_EDGE('',*,*,#7611,.F.);
#11019=ORIENTED_EDGE('',*,*,#7614,.F.);
#11020=ORIENTED_EDGE('',*,*,#7617,.F.);
#11021=ORIENTED_EDGE('',*,*,#7820,.F.);
#11022=ORIENTED_EDGE('',*,*,#7622,.F.);
#11023=ORIENTED_EDGE('',*,*,#7821,.F.);
#11024=ORIENTED_EDGE('',*,*,#7643,.T.);
#11025=ORIENTED_EDGE('',*,*,#7817,.T.);
#11026=ORIENTED_EDGE('',*,*,#7641,.T.);
#11027=ORIENTED_EDGE('',*,*,#7638,.T.);
#11028=ORIENTED_EDGE('',*,*,#7635,.T.);
#11029=ORIENTED_EDGE('',*,*,#7632,.T.);
#11030=ORIENTED_EDGE('',*,*,#7629,.T.);
#11031=ORIENTED_EDGE('',*,*,#7626,.T.);
#11032=ORIENTED_EDGE('',*,*,#7619,.T.);
#11033=ORIENTED_EDGE('',*,*,#7820,.T.);
#11034=ORIENTED_EDGE('',*,*,#7616,.F.);
#11035=ORIENTED_EDGE('',*,*,#7819,.T.);
#11036=ORIENTED_EDGE('',*,*,#7550,.F.);
#11037=ORIENTED_EDGE('',*,*,#7822,.T.);
#11038=ORIENTED_EDGE('',*,*,#7576,.T.);
#11039=ORIENTED_EDGE('',*,*,#7823,.T.);
#11040=ORIENTED_EDGE('',*,*,#7553,.F.);
#11041=ORIENTED_EDGE('',*,*,#7593,.T.);
#11042=ORIENTED_EDGE('',*,*,#7824,.T.);
#11043=ORIENTED_EDGE('',*,*,#7590,.F.);
#11044=ORIENTED_EDGE('',*,*,#7825,.F.);
#11045=ORIENTED_EDGE('',*,*,#7823,.F.);
#11046=ORIENTED_EDGE('',*,*,#7575,.F.);
#11047=ORIENTED_EDGE('',*,*,#7579,.F.);
#11048=ORIENTED_EDGE('',*,*,#7582,.F.);
#11049=ORIENTED_EDGE('',*,*,#7585,.F.);
#11050=ORIENTED_EDGE('',*,*,#7588,.F.);
#11051=ORIENTED_EDGE('',*,*,#7591,.F.);
#11052=ORIENTED_EDGE('',*,*,#7824,.F.);
#11053=ORIENTED_EDGE('',*,*,#7596,.F.);
#11054=ORIENTED_EDGE('',*,*,#7826,.F.);
#11055=ORIENTED_EDGE('',*,*,#7571,.F.);
#11056=ORIENTED_EDGE('',*,*,#7827,.F.);
#11057=ORIENTED_EDGE('',*,*,#7569,.F.);
#11058=ORIENTED_EDGE('',*,*,#7566,.F.);
#11059=ORIENTED_EDGE('',*,*,#7563,.F.);
#11060=ORIENTED_EDGE('',*,*,#7560,.F.);
#11061=ORIENTED_EDGE('',*,*,#7557,.F.);
#11062=ORIENTED_EDGE('',*,*,#7554,.F.);
#11063=ORIENTED_EDGE('',*,*,#7822,.F.);
#11064=ORIENTED_EDGE('',*,*,#7549,.F.);
#11065=ORIENTED_EDGE('',*,*,#7556,.F.);
#11066=ORIENTED_EDGE('',*,*,#7559,.F.);
#11067=ORIENTED_EDGE('',*,*,#7562,.F.);
#11068=ORIENTED_EDGE('',*,*,#7565,.F.);
#11069=ORIENTED_EDGE('',*,*,#7568,.F.);
#11070=ORIENTED_EDGE('',*,*,#7828,.F.);
#11071=ORIENTED_EDGE('',*,*,#7573,.F.);
#11072=ORIENTED_EDGE('',*,*,#7829,.F.);
#11073=ORIENTED_EDGE('',*,*,#7594,.T.);
#11074=ORIENTED_EDGE('',*,*,#7825,.T.);
#11075=ORIENTED_EDGE('',*,*,#7592,.T.);
#11076=ORIENTED_EDGE('',*,*,#7589,.T.);
#11077=ORIENTED_EDGE('',*,*,#7586,.T.);
#11078=ORIENTED_EDGE('',*,*,#7583,.T.);
#11079=ORIENTED_EDGE('',*,*,#7580,.T.);
#11080=ORIENTED_EDGE('',*,*,#7577,.T.);
#11081=ORIENTED_EDGE('',*,*,#7570,.T.);
#11082=ORIENTED_EDGE('',*,*,#7828,.T.);
#11083=ORIENTED_EDGE('',*,*,#7567,.F.);
#11084=ORIENTED_EDGE('',*,*,#7827,.T.);
#11085=ORIENTED_EDGE('',*,*,#7501,.F.);
#11086=ORIENTED_EDGE('',*,*,#7830,.T.);
#11087=ORIENTED_EDGE('',*,*,#7527,.T.);
#11088=ORIENTED_EDGE('',*,*,#7831,.T.);
#11089=ORIENTED_EDGE('',*,*,#7504,.F.);
#11090=ORIENTED_EDGE('',*,*,#7544,.T.);
#11091=ORIENTED_EDGE('',*,*,#7832,.T.);
#11092=ORIENTED_EDGE('',*,*,#7541,.F.);
#11093=ORIENTED_EDGE('',*,*,#7833,.F.);
#11094=ORIENTED_EDGE('',*,*,#7831,.F.);
#11095=ORIENTED_EDGE('',*,*,#7526,.F.);
#11096=ORIENTED_EDGE('',*,*,#7530,.F.);
#11097=ORIENTED_EDGE('',*,*,#7533,.F.);
#11098=ORIENTED_EDGE('',*,*,#7536,.F.);
#11099=ORIENTED_EDGE('',*,*,#7539,.F.);
#11100=ORIENTED_EDGE('',*,*,#7542,.F.);
#11101=ORIENTED_EDGE('',*,*,#7832,.F.);
#11102=ORIENTED_EDGE('',*,*,#7547,.F.);
#11103=ORIENTED_EDGE('',*,*,#7834,.F.);
#11104=ORIENTED_EDGE('',*,*,#7522,.F.);
#11105=ORIENTED_EDGE('',*,*,#7835,.F.);
#11106=ORIENTED_EDGE('',*,*,#7520,.F.);
#11107=ORIENTED_EDGE('',*,*,#7517,.F.);
#11108=ORIENTED_EDGE('',*,*,#7514,.F.);
#11109=ORIENTED_EDGE('',*,*,#7511,.F.);
#11110=ORIENTED_EDGE('',*,*,#7508,.F.);
#11111=ORIENTED_EDGE('',*,*,#7505,.F.);
#11112=ORIENTED_EDGE('',*,*,#7830,.F.);
#11113=ORIENTED_EDGE('',*,*,#7500,.F.);
#11114=ORIENTED_EDGE('',*,*,#7507,.F.);
#11115=ORIENTED_EDGE('',*,*,#7510,.F.);
#11116=ORIENTED_EDGE('',*,*,#7513,.F.);
#11117=ORIENTED_EDGE('',*,*,#7516,.F.);
#11118=ORIENTED_EDGE('',*,*,#7519,.F.);
#11119=ORIENTED_EDGE('',*,*,#7836,.F.);
#11120=ORIENTED_EDGE('',*,*,#7524,.F.);
#11121=ORIENTED_EDGE('',*,*,#7837,.F.);
#11122=ORIENTED_EDGE('',*,*,#7545,.T.);
#11123=ORIENTED_EDGE('',*,*,#7833,.T.);
#11124=ORIENTED_EDGE('',*,*,#7543,.T.);
#11125=ORIENTED_EDGE('',*,*,#7540,.T.);
#11126=ORIENTED_EDGE('',*,*,#7537,.T.);
#11127=ORIENTED_EDGE('',*,*,#7534,.T.);
#11128=ORIENTED_EDGE('',*,*,#7531,.T.);
#11129=ORIENTED_EDGE('',*,*,#7528,.T.);
#11130=ORIENTED_EDGE('',*,*,#7521,.T.);
#11131=ORIENTED_EDGE('',*,*,#7836,.T.);
#11132=ORIENTED_EDGE('',*,*,#7518,.F.);
#11133=ORIENTED_EDGE('',*,*,#7835,.T.);
#11134=ORIENTED_EDGE('',*,*,#7452,.F.);
#11135=ORIENTED_EDGE('',*,*,#7838,.T.);
#11136=ORIENTED_EDGE('',*,*,#7478,.T.);
#11137=ORIENTED_EDGE('',*,*,#7839,.T.);
#11138=ORIENTED_EDGE('',*,*,#7455,.F.);
#11139=ORIENTED_EDGE('',*,*,#7495,.T.);
#11140=ORIENTED_EDGE('',*,*,#7840,.T.);
#11141=ORIENTED_EDGE('',*,*,#7492,.F.);
#11142=ORIENTED_EDGE('',*,*,#7841,.F.);
#11143=ORIENTED_EDGE('',*,*,#7839,.F.);
#11144=ORIENTED_EDGE('',*,*,#7477,.F.);
#11145=ORIENTED_EDGE('',*,*,#7481,.F.);
#11146=ORIENTED_EDGE('',*,*,#7484,.F.);
#11147=ORIENTED_EDGE('',*,*,#7487,.F.);
#11148=ORIENTED_EDGE('',*,*,#7490,.F.);
#11149=ORIENTED_EDGE('',*,*,#7493,.F.);
#11150=ORIENTED_EDGE('',*,*,#7840,.F.);
#11151=ORIENTED_EDGE('',*,*,#7498,.F.);
#11152=ORIENTED_EDGE('',*,*,#7842,.F.);
#11153=ORIENTED_EDGE('',*,*,#7473,.F.);
#11154=ORIENTED_EDGE('',*,*,#7843,.F.);
#11155=ORIENTED_EDGE('',*,*,#7471,.F.);
#11156=ORIENTED_EDGE('',*,*,#7468,.F.);
#11157=ORIENTED_EDGE('',*,*,#7465,.F.);
#11158=ORIENTED_EDGE('',*,*,#7462,.F.);
#11159=ORIENTED_EDGE('',*,*,#7459,.F.);
#11160=ORIENTED_EDGE('',*,*,#7456,.F.);
#11161=ORIENTED_EDGE('',*,*,#7838,.F.);
#11162=ORIENTED_EDGE('',*,*,#7451,.F.);
#11163=ORIENTED_EDGE('',*,*,#7458,.F.);
#11164=ORIENTED_EDGE('',*,*,#7461,.F.);
#11165=ORIENTED_EDGE('',*,*,#7464,.F.);
#11166=ORIENTED_EDGE('',*,*,#7467,.F.);
#11167=ORIENTED_EDGE('',*,*,#7470,.F.);
#11168=ORIENTED_EDGE('',*,*,#7844,.F.);
#11169=ORIENTED_EDGE('',*,*,#7475,.F.);
#11170=ORIENTED_EDGE('',*,*,#7845,.F.);
#11171=ORIENTED_EDGE('',*,*,#7496,.T.);
#11172=ORIENTED_EDGE('',*,*,#7841,.T.);
#11173=ORIENTED_EDGE('',*,*,#7494,.T.);
#11174=ORIENTED_EDGE('',*,*,#7491,.T.);
#11175=ORIENTED_EDGE('',*,*,#7488,.T.);
#11176=ORIENTED_EDGE('',*,*,#7485,.T.);
#11177=ORIENTED_EDGE('',*,*,#7482,.T.);
#11178=ORIENTED_EDGE('',*,*,#7479,.T.);
#11179=ORIENTED_EDGE('',*,*,#7472,.T.);
#11180=ORIENTED_EDGE('',*,*,#7844,.T.);
#11181=ORIENTED_EDGE('',*,*,#7469,.F.);
#11182=ORIENTED_EDGE('',*,*,#7843,.T.);
#11183=ORIENTED_EDGE('',*,*,#7846,.F.);
#11184=ORIENTED_EDGE('',*,*,#7847,.T.);
#11185=ORIENTED_EDGE('',*,*,#7848,.F.);
#11186=ORIENTED_EDGE('',*,*,#7847,.F.);
#11187=ORIENTED_EDGE('',*,*,#7846,.T.);
#11188=ORIENTED_EDGE('',*,*,#7849,.T.);
#11189=ORIENTED_EDGE('',*,*,#7849,.F.);
#11190=ORIENTED_EDGE('',*,*,#7850,.T.);
#11191=ORIENTED_EDGE('',*,*,#7851,.T.);
#11192=ORIENTED_EDGE('',*,*,#7850,.F.);
#11193=ORIENTED_EDGE('',*,*,#7852,.F.);
#11194=ORIENTED_EDGE('',*,*,#7853,.T.);
#11195=ORIENTED_EDGE('',*,*,#7854,.T.);
#11196=ORIENTED_EDGE('',*,*,#7853,.F.);
#11197=ORIENTED_EDGE('',*,*,#7852,.T.);
#11198=ORIENTED_EDGE('',*,*,#7821,.T.);
#11199=ORIENTED_EDGE('',*,*,#7621,.T.);
#11200=ORIENTED_EDGE('',*,*,#7818,.T.);
#11201=ORIENTED_EDGE('',*,*,#7644,.T.);
#11202=ORIENTED_EDGE('',*,*,#7829,.T.);
#11203=ORIENTED_EDGE('',*,*,#7572,.T.);
#11204=ORIENTED_EDGE('',*,*,#7826,.T.);
#11205=ORIENTED_EDGE('',*,*,#7595,.T.);
#11206=ORIENTED_EDGE('',*,*,#7837,.T.);
#11207=ORIENTED_EDGE('',*,*,#7523,.T.);
#11208=ORIENTED_EDGE('',*,*,#7834,.T.);
#11209=ORIENTED_EDGE('',*,*,#7546,.T.);
#11210=ORIENTED_EDGE('',*,*,#7845,.T.);
#11211=ORIENTED_EDGE('',*,*,#7474,.T.);
#11212=ORIENTED_EDGE('',*,*,#7842,.T.);
#11213=ORIENTED_EDGE('',*,*,#7497,.T.);
#11214=ORIENTED_EDGE('',*,*,#7848,.T.);
#11215=ORIENTED_EDGE('',*,*,#7854,.F.);
#11216=ORIENTED_EDGE('',*,*,#7797,.T.);
#11217=ORIENTED_EDGE('',*,*,#7729,.T.);
#11218=ORIENTED_EDGE('',*,*,#7794,.T.);
#11219=ORIENTED_EDGE('',*,*,#7746,.T.);
#11220=ORIENTED_EDGE('',*,*,#7813,.T.);
#11221=ORIENTED_EDGE('',*,*,#7661,.T.);
#11222=ORIENTED_EDGE('',*,*,#7810,.T.);
#11223=ORIENTED_EDGE('',*,*,#7678,.T.);
#11224=ORIENTED_EDGE('',*,*,#7503,.T.);
#11225=ORIENTED_EDGE('',*,*,#7454,.T.);
#11226=ORIENTED_EDGE('',*,*,#7552,.T.);
#11227=ORIENTED_EDGE('',*,*,#7601,.T.);
#11228=ORIENTED_EDGE('',*,*,#7851,.F.);
#11229=ORIENTED_EDGE('',*,*,#7805,.T.);
#11230=ORIENTED_EDGE('',*,*,#7695,.T.);
#11231=ORIENTED_EDGE('',*,*,#7802,.T.);
#11232=ORIENTED_EDGE('',*,*,#7712,.T.);
#11233=ORIENTED_EDGE('',*,*,#7789,.T.);
#11234=ORIENTED_EDGE('',*,*,#7763,.T.);
#11235=ORIENTED_EDGE('',*,*,#7786,.T.);
#11236=ORIENTED_EDGE('',*,*,#7780,.T.);
#13540=CYLINDRICAL_SURFACE('',#15194,3.38975);
#13541=CYLINDRICAL_SURFACE('',#15198,3.38975);
#13542=CYLINDRICAL_SURFACE('',#15199,3.38975);
#13543=CYLINDRICAL_SURFACE('',#15200,3.38975);
#13544=CYLINDRICAL_SURFACE('',#15201,3.38975);
#13545=CYLINDRICAL_SURFACE('',#15202,3.38975);
#13546=CYLINDRICAL_SURFACE('',#15203,3.38975);
#13547=CYLINDRICAL_SURFACE('',#15205,4.085);
#13548=CYLINDRICAL_SURFACE('',#15207,4.085);
#13549=CYLINDRICAL_SURFACE('',#15208,4.085);
#13550=CYLINDRICAL_SURFACE('',#15209,4.085);
#13551=CYLINDRICAL_SURFACE('',#15210,4.085);
#13552=CYLINDRICAL_SURFACE('',#15211,4.085);
#13553=CYLINDRICAL_SURFACE('',#15212,4.085);
#13554=CYLINDRICAL_SURFACE('',#15214,3.38975);
#13555=CYLINDRICAL_SURFACE('',#15218,3.38975);
#13556=CYLINDRICAL_SURFACE('',#15219,3.38975);
#13557=CYLINDRICAL_SURFACE('',#15220,3.38975);
#13558=CYLINDRICAL_SURFACE('',#15221,3.38975);
#13559=CYLINDRICAL_SURFACE('',#15222,3.38975);
#13560=CYLINDRICAL_SURFACE('',#15223,3.38975);
#13561=CYLINDRICAL_SURFACE('',#15225,4.085);
#13562=CYLINDRICAL_SURFACE('',#15227,4.085);
#13563=CYLINDRICAL_SURFACE('',#15228,4.085);
#13564=CYLINDRICAL_SURFACE('',#15229,4.085);
#13565=CYLINDRICAL_SURFACE('',#15230,4.085);
#13566=CYLINDRICAL_SURFACE('',#15231,4.085);
#13567=CYLINDRICAL_SURFACE('',#15232,4.085);
#13568=CYLINDRICAL_SURFACE('',#15234,3.38975);
#13569=CYLINDRICAL_SURFACE('',#15238,3.38975);
#13570=CYLINDRICAL_SURFACE('',#15239,3.38975);
#13571=CYLINDRICAL_SURFACE('',#15240,3.38975);
#13572=CYLINDRICAL_SURFACE('',#15241,3.38975);
#13573=CYLINDRICAL_SURFACE('',#15242,3.38975);
#13574=CYLINDRICAL_SURFACE('',#15243,3.38975);
#13575=CYLINDRICAL_SURFACE('',#15245,4.085);
#13576=CYLINDRICAL_SURFACE('',#15247,4.085);
#13577=CYLINDRICAL_SURFACE('',#15248,4.085);
#13578=CYLINDRICAL_SURFACE('',#15249,4.085);
#13579=CYLINDRICAL_SURFACE('',#15250,4.085);
#13580=CYLINDRICAL_SURFACE('',#15251,4.085);
#13581=CYLINDRICAL_SURFACE('',#15252,4.085);
#13582=CYLINDRICAL_SURFACE('',#15254,3.38975);
#13583=CYLINDRICAL_SURFACE('',#15258,3.38975);
#13584=CYLINDRICAL_SURFACE('',#15259,3.38975);
#13585=CYLINDRICAL_SURFACE('',#15260,3.38975);
#13586=CYLINDRICAL_SURFACE('',#15261,3.38975);
#13587=CYLINDRICAL_SURFACE('',#15262,3.38975);
#13588=CYLINDRICAL_SURFACE('',#15263,3.38975);
#13589=CYLINDRICAL_SURFACE('',#15265,4.085);
#13590=CYLINDRICAL_SURFACE('',#15267,4.085);
#13591=CYLINDRICAL_SURFACE('',#15268,4.085);
#13592=CYLINDRICAL_SURFACE('',#15269,4.085);
#13593=CYLINDRICAL_SURFACE('',#15270,4.085);
#13594=CYLINDRICAL_SURFACE('',#15271,4.085);
#13595=CYLINDRICAL_SURFACE('',#15272,4.085);
#13596=CYLINDRICAL_SURFACE('',#15274,4.263);
#13597=CYLINDRICAL_SURFACE('',#15277,4.263);
#13598=CYLINDRICAL_SURFACE('',#15278,4.263);
#13599=CYLINDRICAL_SURFACE('',#15279,4.263);
#13600=CYLINDRICAL_SURFACE('',#15281,5.099);
#13601=CYLINDRICAL_SURFACE('',#15283,5.099);
#13602=CYLINDRICAL_SURFACE('',#15284,5.099);
#13603=CYLINDRICAL_SURFACE('',#15285,5.099);
#13604=CYLINDRICAL_SURFACE('',#15286,5.099);
#13605=CYLINDRICAL_SURFACE('',#15288,4.263);
#13606=CYLINDRICAL_SURFACE('',#15291,4.263);
#13607=CYLINDRICAL_SURFACE('',#15292,4.263);
#13608=CYLINDRICAL_SURFACE('',#15293,4.263);
#13609=CYLINDRICAL_SURFACE('',#15295,5.099);
#13610=CYLINDRICAL_SURFACE('',#15297,5.099);
#13611=CYLINDRICAL_SURFACE('',#15298,5.099);
#13612=CYLINDRICAL_SURFACE('',#15299,5.099);
#13613=CYLINDRICAL_SURFACE('',#15300,5.099);
#13614=CYLINDRICAL_SURFACE('',#15302,4.263);
#13615=CYLINDRICAL_SURFACE('',#15305,4.263);
#13616=CYLINDRICAL_SURFACE('',#15306,4.263);
#13617=CYLINDRICAL_SURFACE('',#15307,4.263);
#13618=CYLINDRICAL_SURFACE('',#15309,5.099);
#13619=CYLINDRICAL_SURFACE('',#15311,5.099);
#13620=CYLINDRICAL_SURFACE('',#15312,5.099);
#13621=CYLINDRICAL_SURFACE('',#15313,5.099);
#13622=CYLINDRICAL_SURFACE('',#15314,5.099);
#13623=CYLINDRICAL_SURFACE('',#15316,4.263);
#13624=CYLINDRICAL_SURFACE('',#15319,4.263);
#13625=CYLINDRICAL_SURFACE('',#15320,4.263);
#13626=CYLINDRICAL_SURFACE('',#15321,4.263);
#13627=CYLINDRICAL_SURFACE('',#15323,5.099);
#13628=CYLINDRICAL_SURFACE('',#15325,5.099);
#13629=CYLINDRICAL_SURFACE('',#15326,5.099);
#13630=CYLINDRICAL_SURFACE('',#15327,5.099);
#13631=CYLINDRICAL_SURFACE('',#15328,5.099);
#13632=CYLINDRICAL_SURFACE('',#15331,5.099);
#13633=CYLINDRICAL_SURFACE('',#15332,4.263);
#13634=CYLINDRICAL_SURFACE('',#15334,5.099);
#13635=CYLINDRICAL_SURFACE('',#15335,4.263);
#13636=CYLINDRICAL_SURFACE('',#15337,5.099);
#13637=CYLINDRICAL_SURFACE('',#15338,4.263);
#13638=CYLINDRICAL_SURFACE('',#15340,5.099);
#13639=CYLINDRICAL_SURFACE('',#15341,4.263);
#13640=CYLINDRICAL_SURFACE('',#15347,4.085);
#13641=CYLINDRICAL_SURFACE('',#15348,3.38975);
#13642=CYLINDRICAL_SURFACE('',#15350,4.085);
#13643=CYLINDRICAL_SURFACE('',#15351,3.38975);
#13644=CYLINDRICAL_SURFACE('',#15353,4.085);
#13645=CYLINDRICAL_SURFACE('',#15354,3.38975);
#13646=CYLINDRICAL_SURFACE('',#15356,4.085);
#13647=CYLINDRICAL_SURFACE('',#15357,3.38975);
#13648=CYLINDRICAL_SURFACE('',#15358,40.);
#13649=CYLINDRICAL_SURFACE('',#15363,20.);
#13650=CYLINDRICAL_SURFACE('',#15365,110.);
#14207=ADVANCED_FACE('',(#779),#13540,.F.);
#14208=ADVANCED_FACE('',(#780),#13541,.F.);
#14209=ADVANCED_FACE('',(#781),#13542,.F.);
#14210=ADVANCED_FACE('',(#782),#13543,.F.);
#14211=ADVANCED_FACE('',(#783),#13544,.F.);
#14212=ADVANCED_FACE('',(#784),#13545,.F.);
#14213=ADVANCED_FACE('',(#785),#13546,.F.);
#14214=ADVANCED_FACE('',(#786),#13547,.F.);
#14215=ADVANCED_FACE('',(#787),#13548,.F.);
#14216=ADVANCED_FACE('',(#788),#13549,.F.);
#14217=ADVANCED_FACE('',(#789),#13550,.F.);
#14218=ADVANCED_FACE('',(#790),#13551,.F.);
#14219=ADVANCED_FACE('',(#791),#13552,.F.);
#14220=ADVANCED_FACE('',(#792),#13553,.F.);
#14221=ADVANCED_FACE('',(#793),#13554,.F.);
#14222=ADVANCED_FACE('',(#794),#13555,.F.);
#14223=ADVANCED_FACE('',(#795),#13556,.F.);
#14224=ADVANCED_FACE('',(#796),#13557,.F.);
#14225=ADVANCED_FACE('',(#797),#13558,.F.);
#14226=ADVANCED_FACE('',(#798),#13559,.F.);
#14227=ADVANCED_FACE('',(#799),#13560,.F.);
#14228=ADVANCED_FACE('',(#800),#13561,.F.);
#14229=ADVANCED_FACE('',(#801),#13562,.F.);
#14230=ADVANCED_FACE('',(#802),#13563,.F.);
#14231=ADVANCED_FACE('',(#803),#13564,.F.);
#14232=ADVANCED_FACE('',(#804),#13565,.F.);
#14233=ADVANCED_FACE('',(#805),#13566,.F.);
#14234=ADVANCED_FACE('',(#806),#13567,.F.);
#14235=ADVANCED_FACE('',(#807),#13568,.F.);
#14236=ADVANCED_FACE('',(#808),#13569,.F.);
#14237=ADVANCED_FACE('',(#809),#13570,.F.);
#14238=ADVANCED_FACE('',(#810),#13571,.F.);
#14239=ADVANCED_FACE('',(#811),#13572,.F.);
#14240=ADVANCED_FACE('',(#812),#13573,.F.);
#14241=ADVANCED_FACE('',(#813),#13574,.F.);
#14242=ADVANCED_FACE('',(#814),#13575,.F.);
#14243=ADVANCED_FACE('',(#815),#13576,.F.);
#14244=ADVANCED_FACE('',(#816),#13577,.F.);
#14245=ADVANCED_FACE('',(#817),#13578,.F.);
#14246=ADVANCED_FACE('',(#818),#13579,.F.);
#14247=ADVANCED_FACE('',(#819),#13580,.F.);
#14248=ADVANCED_FACE('',(#820),#13581,.F.);
#14249=ADVANCED_FACE('',(#821),#13582,.F.);
#14250=ADVANCED_FACE('',(#822),#13583,.F.);
#14251=ADVANCED_FACE('',(#823),#13584,.F.);
#14252=ADVANCED_FACE('',(#824),#13585,.F.);
#14253=ADVANCED_FACE('',(#825),#13586,.F.);
#14254=ADVANCED_FACE('',(#826),#13587,.F.);
#14255=ADVANCED_FACE('',(#827),#13588,.F.);
#14256=ADVANCED_FACE('',(#828),#13589,.F.);
#14257=ADVANCED_FACE('',(#829),#13590,.F.);
#14258=ADVANCED_FACE('',(#830),#13591,.F.);
#14259=ADVANCED_FACE('',(#831),#13592,.F.);
#14260=ADVANCED_FACE('',(#832),#13593,.F.);
#14261=ADVANCED_FACE('',(#833),#13594,.F.);
#14262=ADVANCED_FACE('',(#834),#13595,.F.);
#14263=ADVANCED_FACE('',(#835),#13596,.F.);
#14264=ADVANCED_FACE('',(#836),#13597,.F.);
#14265=ADVANCED_FACE('',(#837),#13598,.F.);
#14266=ADVANCED_FACE('',(#838),#13599,.F.);
#14267=ADVANCED_FACE('',(#839),#13600,.F.);
#14268=ADVANCED_FACE('',(#840),#13601,.F.);
#14269=ADVANCED_FACE('',(#841),#13602,.F.);
#14270=ADVANCED_FACE('',(#842),#13603,.F.);
#14271=ADVANCED_FACE('',(#843),#13604,.F.);
#14272=ADVANCED_FACE('',(#844),#13605,.F.);
#14273=ADVANCED_FACE('',(#845),#13606,.F.);
#14274=ADVANCED_FACE('',(#846),#13607,.F.);
#14275=ADVANCED_FACE('',(#847),#13608,.F.);
#14276=ADVANCED_FACE('',(#848),#13609,.F.);
#14277=ADVANCED_FACE('',(#849),#13610,.F.);
#14278=ADVANCED_FACE('',(#850),#13611,.F.);
#14279=ADVANCED_FACE('',(#851),#13612,.F.);
#14280=ADVANCED_FACE('',(#852),#13613,.F.);
#14281=ADVANCED_FACE('',(#853),#13614,.F.);
#14282=ADVANCED_FACE('',(#854),#13615,.F.);
#14283=ADVANCED_FACE('',(#855),#13616,.F.);
#14284=ADVANCED_FACE('',(#856),#13617,.F.);
#14285=ADVANCED_FACE('',(#857),#13618,.F.);
#14286=ADVANCED_FACE('',(#858),#13619,.F.);
#14287=ADVANCED_FACE('',(#859),#13620,.F.);
#14288=ADVANCED_FACE('',(#860),#13621,.F.);
#14289=ADVANCED_FACE('',(#861),#13622,.F.);
#14290=ADVANCED_FACE('',(#862),#13623,.F.);
#14291=ADVANCED_FACE('',(#863),#13624,.F.);
#14292=ADVANCED_FACE('',(#864),#13625,.F.);
#14293=ADVANCED_FACE('',(#865),#13626,.F.);
#14294=ADVANCED_FACE('',(#866),#13627,.F.);
#14295=ADVANCED_FACE('',(#867),#13628,.F.);
#14296=ADVANCED_FACE('',(#868),#13629,.F.);
#14297=ADVANCED_FACE('',(#869),#13630,.F.);
#14298=ADVANCED_FACE('',(#870),#13631,.F.);
#14299=ADVANCED_FACE('',(#871),#435,.F.);
#14300=ADVANCED_FACE('',(#872),#13632,.F.);
#14301=ADVANCED_FACE('',(#873),#274,.F.);
#14302=ADVANCED_FACE('',(#874),#275,.F.);
#14303=ADVANCED_FACE('',(#875),#13633,.F.);
#14304=ADVANCED_FACE('',(#876),#436,.F.);
#14305=ADVANCED_FACE('',(#877),#13634,.F.);
#14306=ADVANCED_FACE('',(#878),#276,.F.);
#14307=ADVANCED_FACE('',(#879),#277,.F.);
#14308=ADVANCED_FACE('',(#880),#13635,.F.);
#14309=ADVANCED_FACE('',(#881),#437,.F.);
#14310=ADVANCED_FACE('',(#882),#13636,.F.);
#14311=ADVANCED_FACE('',(#883),#278,.F.);
#14312=ADVANCED_FACE('',(#884),#279,.F.);
#14313=ADVANCED_FACE('',(#885),#13637,.F.);
#14314=ADVANCED_FACE('',(#886),#438,.F.);
#14315=ADVANCED_FACE('',(#887),#13638,.F.);
#14316=ADVANCED_FACE('',(#888),#280,.F.);
#14317=ADVANCED_FACE('',(#889),#281,.F.);
#14318=ADVANCED_FACE('',(#890),#13639,.F.);
#14319=ADVANCED_FACE('',(#891),#439,.F.);
#14320=ADVANCED_FACE('',(#892),#440,.F.);
#14321=ADVANCED_FACE('',(#893),#441,.F.);
#14322=ADVANCED_FACE('',(#894),#442,.F.);
#14323=ADVANCED_FACE('',(#895),#443,.T.);
#14324=ADVANCED_FACE('',(#896),#13640,.F.);
#14325=ADVANCED_FACE('',(#897),#282,.F.);
#14326=ADVANCED_FACE('',(#898),#283,.F.);
#14327=ADVANCED_FACE('',(#899),#13641,.F.);
#14328=ADVANCED_FACE('',(#900),#444,.T.);
#14329=ADVANCED_FACE('',(#901),#13642,.F.);
#14330=ADVANCED_FACE('',(#902),#284,.F.);
#14331=ADVANCED_FACE('',(#903),#285,.F.);
#14332=ADVANCED_FACE('',(#904),#13643,.F.);
#14333=ADVANCED_FACE('',(#905),#445,.T.);
#14334=ADVANCED_FACE('',(#906),#13644,.F.);
#14335=ADVANCED_FACE('',(#907),#286,.F.);
#14336=ADVANCED_FACE('',(#908),#287,.F.);
#14337=ADVANCED_FACE('',(#909),#13645,.F.);
#14338=ADVANCED_FACE('',(#910),#446,.T.);
#14339=ADVANCED_FACE('',(#911),#13646,.F.);
#14340=ADVANCED_FACE('',(#912),#288,.F.);
#14341=ADVANCED_FACE('',(#913),#289,.F.);
#14342=ADVANCED_FACE('',(#914),#13647,.F.);
#14343=ADVANCED_FACE('',(#915),#13648,.T.);
#14344=ADVANCED_FACE('',(#916,#328),#447,.T.);
#14345=ADVANCED_FACE('',(#917),#13649,.F.);
#14346=ADVANCED_FACE('',(#918),#13650,.T.);
#14347=ADVANCED_FACE('',(#919,#329,#330,#331,#332,#333),#448,.T.);
#14348=ADVANCED_FACE('',(#920,#334,#335,#336,#337,#338,#339,#340,#341,#342),
#449,.F.);
#14732=CLOSED_SHELL('',(#14207,#14208,#14209,#14210,#14211,#14212,#14213,
#14214,#14215,#14216,#14217,#14218,#14219,#14220,#14221,#14222,#14223,#14224,
#14225,#14226,#14227,#14228,#14229,#14230,#14231,#14232,#14233,#14234,#14235,
#14236,#14237,#14238,#14239,#14240,#14241,#14242,#14243,#14244,#14245,#14246,
#14247,#14248,#14249,#14250,#14251,#14252,#14253,#14254,#14255,#14256,#14257,
#14258,#14259,#14260,#14261,#14262,#14263,#14264,#14265,#14266,#14267,#14268,
#14269,#14270,#14271,#14272,#14273,#14274,#14275,#14276,#14277,#14278,#14279,
#14280,#14281,#14282,#14283,#14284,#14285,#14286,#14287,#14288,#14289,#14290,
#14291,#14292,#14293,#14294,#14295,#14296,#14297,#14298,#14299,#14300,#14301,
#14302,#14303,#14304,#14305,#14306,#14307,#14308,#14309,#14310,#14311,#14312,
#14313,#14314,#14315,#14316,#14317,#14318,#14319,#14320,#14321,#14322,#14323,
#14324,#14325,#14326,#14327,#14328,#14329,#14330,#14331,#14332,#14333,#14334,
#14335,#14336,#14337,#14338,#14339,#14340,#14341,#14342,#14343,#14344,#14345,
#14346,#14347,#14348));
#15193=AXIS2_PLACEMENT_3D('',#31639,#16836,#16837);
#15194=AXIS2_PLACEMENT_3D('',#31640,#16838,#16839);
#15195=AXIS2_PLACEMENT_3D('',#31653,#16841,#16842);
#15196=AXIS2_PLACEMENT_3D('',#31656,#16844,#16845);
#15197=AXIS2_PLACEMENT_3D('',#31658,#16846,#16847);
#15198=AXIS2_PLACEMENT_3D('',#31672,#16848,#16849);
#15199=AXIS2_PLACEMENT_3D('',#31726,#16851,#16852);
#15200=AXIS2_PLACEMENT_3D('',#31774,#16854,#16855);
#15201=AXIS2_PLACEMENT_3D('',#31825,#16857,#16858);
#15202=AXIS2_PLACEMENT_3D('',#31876,#16860,#16861);
#15203=AXIS2_PLACEMENT_3D('',#31924,#16863,#16864);
#15204=AXIS2_PLACEMENT_3D('',#31943,#16866,#16867);
#15205=AXIS2_PLACEMENT_3D('',#31963,#16868,#16869);
#15206=AXIS2_PLACEMENT_3D('',#31978,#16871,#16872);
#15207=AXIS2_PLACEMENT_3D('',#31989,#16873,#16874);
#15208=AXIS2_PLACEMENT_3D('',#32014,#16876,#16877);
#15209=AXIS2_PLACEMENT_3D('',#32039,#16879,#16880);
#15210=AXIS2_PLACEMENT_3D('',#32063,#16882,#16883);
#15211=AXIS2_PLACEMENT_3D('',#32088,#16885,#16886);
#15212=AXIS2_PLACEMENT_3D('',#32113,#16888,#16889);
#15213=AXIS2_PLACEMENT_3D('',#32124,#16891,#16892);
#15214=AXIS2_PLACEMENT_3D('',#32130,#16893,#16894);
#15215=AXIS2_PLACEMENT_3D('',#32143,#16896,#16897);
#15216=AXIS2_PLACEMENT_3D('',#32146,#16899,#16900);
#15217=AXIS2_PLACEMENT_3D('',#32148,#16901,#16902);
#15218=AXIS2_PLACEMENT_3D('',#32162,#16903,#16904);
#15219=AXIS2_PLACEMENT_3D('',#32216,#16906,#16907);
#15220=AXIS2_PLACEMENT_3D('',#32264,#16909,#16910);
#15221=AXIS2_PLACEMENT_3D('',#32315,#16912,#16913);
#15222=AXIS2_PLACEMENT_3D('',#32366,#16915,#16916);
#15223=AXIS2_PLACEMENT_3D('',#32414,#16918,#16919);
#15224=AXIS2_PLACEMENT_3D('',#32433,#16921,#16922);
#15225=AXIS2_PLACEMENT_3D('',#32453,#16923,#16924);
#15226=AXIS2_PLACEMENT_3D('',#32468,#16926,#16927);
#15227=AXIS2_PLACEMENT_3D('',#32479,#16928,#16929);
#15228=AXIS2_PLACEMENT_3D('',#32504,#16931,#16932);
#15229=AXIS2_PLACEMENT_3D('',#32529,#16934,#16935);
#15230=AXIS2_PLACEMENT_3D('',#32553,#16937,#16938);
#15231=AXIS2_PLACEMENT_3D('',#32578,#16940,#16941);
#15232=AXIS2_PLACEMENT_3D('',#32603,#16943,#16944);
#15233=AXIS2_PLACEMENT_3D('',#32614,#16946,#16947);
#15234=AXIS2_PLACEMENT_3D('',#32620,#16948,#16949);
#15235=AXIS2_PLACEMENT_3D('',#32633,#16951,#16952);
#15236=AXIS2_PLACEMENT_3D('',#32636,#16954,#16955);
#15237=AXIS2_PLACEMENT_3D('',#32638,#16956,#16957);
#15238=AXIS2_PLACEMENT_3D('',#32652,#16958,#16959);
#15239=AXIS2_PLACEMENT_3D('',#32706,#16961,#16962);
#15240=AXIS2_PLACEMENT_3D('',#32754,#16964,#16965);
#15241=AXIS2_PLACEMENT_3D('',#32805,#16967,#16968);
#15242=AXIS2_PLACEMENT_3D('',#32856,#16970,#16971);
#15243=AXIS2_PLACEMENT_3D('',#32904,#16973,#16974);
#15244=AXIS2_PLACEMENT_3D('',#32923,#16976,#16977);
#15245=AXIS2_PLACEMENT_3D('',#32943,#16978,#16979);
#15246=AXIS2_PLACEMENT_3D('',#32958,#16981,#16982);
#15247=AXIS2_PLACEMENT_3D('',#32969,#16983,#16984);
#15248=AXIS2_PLACEMENT_3D('',#32994,#16986,#16987);
#15249=AXIS2_PLACEMENT_3D('',#33019,#16989,#16990);
#15250=AXIS2_PLACEMENT_3D('',#33043,#16992,#16993);
#15251=AXIS2_PLACEMENT_3D('',#33068,#16995,#16996);
#15252=AXIS2_PLACEMENT_3D('',#33093,#16998,#16999);
#15253=AXIS2_PLACEMENT_3D('',#33104,#17001,#17002);
#15254=AXIS2_PLACEMENT_3D('',#33110,#17003,#17004);
#15255=AXIS2_PLACEMENT_3D('',#33123,#17006,#17007);
#15256=AXIS2_PLACEMENT_3D('',#33126,#17009,#17010);
#15257=AXIS2_PLACEMENT_3D('',#33128,#17011,#17012);
#15258=AXIS2_PLACEMENT_3D('',#33142,#17013,#17014);
#15259=AXIS2_PLACEMENT_3D('',#33196,#17016,#17017);
#15260=AXIS2_PLACEMENT_3D('',#33244,#17019,#17020);
#15261=AXIS2_PLACEMENT_3D('',#33295,#17022,#17023);
#15262=AXIS2_PLACEMENT_3D('',#33346,#17025,#17026);
#15263=AXIS2_PLACEMENT_3D('',#33394,#17028,#17029);
#15264=AXIS2_PLACEMENT_3D('',#33413,#17031,#17032);
#15265=AXIS2_PLACEMENT_3D('',#33433,#17033,#17034);
#15266=AXIS2_PLACEMENT_3D('',#33448,#17036,#17037);
#15267=AXIS2_PLACEMENT_3D('',#33459,#17038,#17039);
#15268=AXIS2_PLACEMENT_3D('',#33484,#17041,#17042);
#15269=AXIS2_PLACEMENT_3D('',#33509,#17044,#17045);
#15270=AXIS2_PLACEMENT_3D('',#33533,#17047,#17048);
#15271=AXIS2_PLACEMENT_3D('',#33558,#17050,#17051);
#15272=AXIS2_PLACEMENT_3D('',#33583,#17053,#17054);
#15273=AXIS2_PLACEMENT_3D('',#33594,#17056,#17057);
#15274=AXIS2_PLACEMENT_3D('',#33600,#17058,#17059);
#15275=AXIS2_PLACEMENT_3D('',#33640,#17061,#17062);
#15276=AXIS2_PLACEMENT_3D('',#33648,#17064,#17065);
#15277=AXIS2_PLACEMENT_3D('',#33692,#17066,#17067);
#15278=AXIS2_PLACEMENT_3D('',#33776,#17069,#17070);
#15279=AXIS2_PLACEMENT_3D('',#33851,#17072,#17073);
#15280=AXIS2_PLACEMENT_3D('',#33882,#17075,#17076);
#15281=AXIS2_PLACEMENT_3D('',#33920,#17077,#17078);
#15282=AXIS2_PLACEMENT_3D('',#33934,#17080,#17081);
#15283=AXIS2_PLACEMENT_3D('',#33945,#17082,#17083);
#15284=AXIS2_PLACEMENT_3D('',#33982,#17085,#17086);
#15285=AXIS2_PLACEMENT_3D('',#34016,#17088,#17089);
#15286=AXIS2_PLACEMENT_3D('',#34052,#17091,#17092);
#15287=AXIS2_PLACEMENT_3D('',#34064,#17094,#17095);
#15288=AXIS2_PLACEMENT_3D('',#34072,#17096,#17097);
#15289=AXIS2_PLACEMENT_3D('',#34112,#17099,#17100);
#15290=AXIS2_PLACEMENT_3D('',#34120,#17102,#17103);
#15291=AXIS2_PLACEMENT_3D('',#34164,#17104,#17105);
#15292=AXIS2_PLACEMENT_3D('',#34248,#17107,#17108);
#15293=AXIS2_PLACEMENT_3D('',#34323,#17110,#17111);
#15294=AXIS2_PLACEMENT_3D('',#34354,#17113,#17114);
#15295=AXIS2_PLACEMENT_3D('',#34392,#17115,#17116);
#15296=AXIS2_PLACEMENT_3D('',#34406,#17118,#17119);
#15297=AXIS2_PLACEMENT_3D('',#34417,#17120,#17121);
#15298=AXIS2_PLACEMENT_3D('',#34454,#17123,#17124);
#15299=AXIS2_PLACEMENT_3D('',#34488,#17126,#17127);
#15300=AXIS2_PLACEMENT_3D('',#34524,#17129,#17130);
#15301=AXIS2_PLACEMENT_3D('',#34536,#17132,#17133);
#15302=AXIS2_PLACEMENT_3D('',#34544,#17134,#17135);
#15303=AXIS2_PLACEMENT_3D('',#34584,#17137,#17138);
#15304=AXIS2_PLACEMENT_3D('',#34592,#17140,#17141);
#15305=AXIS2_PLACEMENT_3D('',#34636,#17142,#17143);
#15306=AXIS2_PLACEMENT_3D('',#34720,#17145,#17146);
#15307=AXIS2_PLACEMENT_3D('',#34795,#17148,#17149);
#15308=AXIS2_PLACEMENT_3D('',#34826,#17151,#17152);
#15309=AXIS2_PLACEMENT_3D('',#34864,#17153,#17154);
#15310=AXIS2_PLACEMENT_3D('',#34878,#17156,#17157);
#15311=AXIS2_PLACEMENT_3D('',#34889,#17158,#17159);
#15312=AXIS2_PLACEMENT_3D('',#34926,#17161,#17162);
#15313=AXIS2_PLACEMENT_3D('',#34960,#17164,#17165);
#15314=AXIS2_PLACEMENT_3D('',#34996,#17167,#17168);
#15315=AXIS2_PLACEMENT_3D('',#35008,#17170,#17171);
#15316=AXIS2_PLACEMENT_3D('',#35016,#17172,#17173);
#15317=AXIS2_PLACEMENT_3D('',#35056,#17175,#17176);
#15318=AXIS2_PLACEMENT_3D('',#35064,#17178,#17179);
#15319=AXIS2_PLACEMENT_3D('',#35108,#17180,#17181);
#15320=AXIS2_PLACEMENT_3D('',#35192,#17183,#17184);
#15321=AXIS2_PLACEMENT_3D('',#35267,#17186,#17187);
#15322=AXIS2_PLACEMENT_3D('',#35298,#17189,#17190);
#15323=AXIS2_PLACEMENT_3D('',#35336,#17191,#17192);
#15324=AXIS2_PLACEMENT_3D('',#35350,#17194,#17195);
#15325=AXIS2_PLACEMENT_3D('',#35361,#17196,#17197);
#15326=AXIS2_PLACEMENT_3D('',#35398,#17199,#17200);
#15327=AXIS2_PLACEMENT_3D('',#35432,#17202,#17203);
#15328=AXIS2_PLACEMENT_3D('',#35468,#17205,#17206);
#15329=AXIS2_PLACEMENT_3D('',#35480,#17208,#17209);
#15330=AXIS2_PLACEMENT_3D('',#35488,#17210,#17211);
#15331=AXIS2_PLACEMENT_3D('',#35710,#17212,#17213);
#15332=AXIS2_PLACEMENT_3D('',#36552,#17214,#17215);
#15333=AXIS2_PLACEMENT_3D('',#36553,#17216,#17217);
#15334=AXIS2_PLACEMENT_3D('',#36775,#17218,#17219);
#15335=AXIS2_PLACEMENT_3D('',#37617,#17220,#17221);
#15336=AXIS2_PLACEMENT_3D('',#37618,#17222,#17223);
#15337=AXIS2_PLACEMENT_3D('',#37840,#17224,#17225);
#15338=AXIS2_PLACEMENT_3D('',#38682,#17226,#17227);
#15339=AXIS2_PLACEMENT_3D('',#38683,#17228,#17229);
#15340=AXIS2_PLACEMENT_3D('',#38905,#17230,#17231);
#15341=AXIS2_PLACEMENT_3D('',#39747,#17232,#17233);
#15342=AXIS2_PLACEMENT_3D('',#39748,#17234,#17235);
#15343=AXIS2_PLACEMENT_3D('',#39749,#17236,#17237);
#15344=AXIS2_PLACEMENT_3D('',#39750,#17238,#17239);
#15345=AXIS2_PLACEMENT_3D('',#39751,#17240,#17241);
#15346=AXIS2_PLACEMENT_3D('',#39752,#17242,#17243);
#15347=AXIS2_PLACEMENT_3D('',#39953,#17244,#17245);
#15348=AXIS2_PLACEMENT_3D('',#40624,#17246,#17247);
#15349=AXIS2_PLACEMENT_3D('',#40625,#17248,#17249);
#15350=AXIS2_PLACEMENT_3D('',#40826,#17250,#17251);
#15351=AXIS2_PLACEMENT_3D('',#41497,#17252,#17253);
#15352=AXIS2_PLACEMENT_3D('',#41498,#17254,#17255);
#15353=AXIS2_PLACEMENT_3D('',#41699,#17256,#17257);
#15354=AXIS2_PLACEMENT_3D('',#42370,#17258,#17259);
#15355=AXIS2_PLACEMENT_3D('',#42371,#17260,#17261);
#15356=AXIS2_PLACEMENT_3D('',#42572,#17262,#17263);
#15357=AXIS2_PLACEMENT_3D('',#43243,#17264,#17265);
#15358=AXIS2_PLACEMENT_3D('',#43244,#17266,#17267);
#15359=AXIS2_PLACEMENT_3D('',#43246,#17268,#17269);
#15360=AXIS2_PLACEMENT_3D('',#43249,#17271,#17272);
#15361=AXIS2_PLACEMENT_3D('',#43250,#17273,#17274);
#15362=AXIS2_PLACEMENT_3D('',#43252,#17275,#17276);
#15363=AXIS2_PLACEMENT_3D('',#43253,#17277,#17278);
#15364=AXIS2_PLACEMENT_3D('',#43256,#17280,#17281);
#15365=AXIS2_PLACEMENT_3D('',#43257,#17282,#17283);
#15366=AXIS2_PLACEMENT_3D('',#43259,#17284,#17285);
#15367=AXIS2_PLACEMENT_3D('',#43262,#17287,#17288);
#15368=AXIS2_PLACEMENT_3D('',#43263,#17289,#17290);
#15369=AXIS2_PLACEMENT_3D('',#43264,#17291,#17292);
#16836=DIRECTION('axis',(0.,0.,1.));
#16837=DIRECTION('refdir',(1.,0.,0.));
#16838=DIRECTION('center_axis',(0.,0.,-1.));
#16839=DIRECTION('ref_axis',(1.,0.,0.));
#16840=DIRECTION('',(0.,0.,-1.));
#16841=DIRECTION('center_axis',(0.,0.,1.));
#16842=DIRECTION('ref_axis',(1.,0.,0.));
#16843=DIRECTION('',(0.,0.,-1.));
#16844=DIRECTION('center_axis',(0.,0.,-1.));
#16845=DIRECTION('ref_axis',(1.,0.,0.));
#16846=DIRECTION('center_axis',(0.,0.,1.));
#16847=DIRECTION('ref_axis',(1.,0.,0.));
#16848=DIRECTION('center_axis',(0.,0.,-1.));
#16849=DIRECTION('ref_axis',(1.,0.,0.));
#16850=DIRECTION('',(0.,0.,-1.));
#16851=DIRECTION('center_axis',(0.,0.,-1.));
#16852=DIRECTION('ref_axis',(1.,0.,0.));
#16853=DIRECTION('',(0.,0.,-1.));
#16854=DIRECTION('center_axis',(0.,0.,-1.));
#16855=DIRECTION('ref_axis',(1.,0.,0.));
#16856=DIRECTION('',(0.,0.,-1.));
#16857=DIRECTION('center_axis',(0.,0.,-1.));
#16858=DIRECTION('ref_axis',(1.,0.,0.));
#16859=DIRECTION('',(0.,0.,-1.));
#16860=DIRECTION('center_axis',(0.,0.,-1.));
#16861=DIRECTION('ref_axis',(1.,0.,0.));
#16862=DIRECTION('',(0.,0.,-1.));
#16863=DIRECTION('center_axis',(0.,0.,-1.));
#16864=DIRECTION('ref_axis',(0.937752260636195,-0.347304905913675,0.));
#16865=DIRECTION('',(0.,0.,-1.));
#16866=DIRECTION('center_axis',(0.,0.,-1.));
#16867=DIRECTION('ref_axis',(1.,0.,0.));
#16868=DIRECTION('center_axis',(0.,0.,-1.));
#16869=DIRECTION('ref_axis',(0.999651918108172,0.0263826197079016,0.));
#16870=DIRECTION('',(1.22464679914735E-16,-1.61260571350473E-30,-1.));
#16871=DIRECTION('center_axis',(0.,0.,1.));
#16872=DIRECTION('ref_axis',(1.,-1.30454602648733E-14,0.));
#16873=DIRECTION('center_axis',(0.,0.,-1.));
#16874=DIRECTION('ref_axis',(1.,-1.30454602648733E-14,0.));
#16875=DIRECTION('',(1.22464679914735E-16,-1.61260571350473E-30,-1.));
#16876=DIRECTION('center_axis',(0.,0.,-1.));
#16877=DIRECTION('ref_axis',(1.,-1.30454602648733E-14,0.));
#16878=DIRECTION('',(1.22464679914735E-16,-1.61260571350473E-30,-1.));
#16879=DIRECTION('center_axis',(0.,0.,-1.));
#16880=DIRECTION('ref_axis',(1.,-1.30454602648733E-14,0.));
#16881=DIRECTION('',(1.22464679914735E-16,-1.61260571350473E-30,-1.));
#16882=DIRECTION('center_axis',(0.,0.,-1.));
#16883=DIRECTION('ref_axis',(1.,-1.30454602648733E-14,0.));
#16884=DIRECTION('',(1.22464679914735E-16,-1.61260571350473E-30,-1.));
#16885=DIRECTION('center_axis',(0.,0.,-1.));
#16886=DIRECTION('ref_axis',(1.,-1.30454602648733E-14,0.));
#16887=DIRECTION('',(1.22464679914735E-16,-1.61260571350473E-30,-1.));
#16888=DIRECTION('center_axis',(0.,0.,-1.));
#16889=DIRECTION('ref_axis',(-0.608776360854994,-0.793341882459353,0.));
#16890=DIRECTION('',(1.22464679914735E-16,-1.61260571350473E-30,-1.));
#16891=DIRECTION('center_axis',(0.,0.,-1.));
#16892=DIRECTION('ref_axis',(1.,-1.30454602648733E-14,0.));
#16893=DIRECTION('center_axis',(0.,0.,-1.));
#16894=DIRECTION('ref_axis',(1.,0.,0.));
#16895=DIRECTION('',(0.,0.,-1.));
#16896=DIRECTION('center_axis',(0.,0.,1.));
#16897=DIRECTION('ref_axis',(1.,0.,0.));
#16898=DIRECTION('',(0.,0.,-1.));
#16899=DIRECTION('center_axis',(0.,0.,-1.));
#16900=DIRECTION('ref_axis',(1.,0.,0.));
#16901=DIRECTION('center_axis',(0.,0.,1.));
#16902=DIRECTION('ref_axis',(1.,0.,0.));
#16903=DIRECTION('center_axis',(0.,0.,-1.));
#16904=DIRECTION('ref_axis',(1.,0.,0.));
#16905=DIRECTION('',(0.,0.,-1.));
#16906=DIRECTION('center_axis',(0.,0.,-1.));
#16907=DIRECTION('ref_axis',(1.,0.,0.));
#16908=DIRECTION('',(0.,0.,-1.));
#16909=DIRECTION('center_axis',(0.,0.,-1.));
#16910=DIRECTION('ref_axis',(1.,0.,0.));
#16911=DIRECTION('',(0.,0.,-1.));
#16912=DIRECTION('center_axis',(0.,0.,-1.));
#16913=DIRECTION('ref_axis',(1.,0.,0.));
#16914=DIRECTION('',(0.,0.,-1.));
#16915=DIRECTION('center_axis',(0.,0.,-1.));
#16916=DIRECTION('ref_axis',(1.,0.,0.));
#16917=DIRECTION('',(0.,0.,-1.));
#16918=DIRECTION('center_axis',(0.,0.,-1.));
#16919=DIRECTION('ref_axis',(0.93775225635851,-0.347304917463781,0.));
#16920=DIRECTION('',(0.,0.,-1.));
#16921=DIRECTION('center_axis',(0.,0.,-1.));
#16922=DIRECTION('ref_axis',(1.,0.,0.));
#16923=DIRECTION('center_axis',(0.,0.,-1.));
#16924=DIRECTION('ref_axis',(0.99965191776215,0.0263826328188801,0.));
#16925=DIRECTION('',(1.22464679914735E-16,-2.1451417520641E-30,-1.));
#16926=DIRECTION('center_axis',(0.,0.,1.));
#16927=DIRECTION('ref_axis',(1.,-1.73939470198311E-14,0.));
#16928=DIRECTION('center_axis',(0.,0.,-1.));
#16929=DIRECTION('ref_axis',(1.,-1.73939470198311E-14,0.));
#16930=DIRECTION('',(1.22464679914735E-16,-2.1451417520641E-30,-1.));
#16931=DIRECTION('center_axis',(0.,0.,-1.));
#16932=DIRECTION('ref_axis',(1.,-1.73939470198311E-14,0.));
#16933=DIRECTION('',(1.22464679914735E-16,-2.1451417520641E-30,-1.));
#16934=DIRECTION('center_axis',(0.,0.,-1.));
#16935=DIRECTION('ref_axis',(1.,-1.73939470198311E-14,0.));
#16936=DIRECTION('',(1.22464679914735E-16,-2.1451417520641E-30,-1.));
#16937=DIRECTION('center_axis',(0.,0.,-1.));
#16938=DIRECTION('ref_axis',(1.,-1.73939470198311E-14,0.));
#16939=DIRECTION('',(1.22464679914735E-16,-2.1451417520641E-30,-1.));
#16940=DIRECTION('center_axis',(0.,0.,-1.));
#16941=DIRECTION('ref_axis',(1.,-1.73939470198311E-14,0.));
#16942=DIRECTION('',(1.22464679914735E-16,-2.1451417520641E-30,-1.));
#16943=DIRECTION('center_axis',(0.,0.,-1.));
#16944=DIRECTION('ref_axis',(-0.608776367541345,-0.793341877328536,0.));
#16945=DIRECTION('',(1.22464679914735E-16,-2.1451417520641E-30,-1.));
#16946=DIRECTION('center_axis',(0.,0.,-1.));
#16947=DIRECTION('ref_axis',(1.,-1.73939470198311E-14,0.));
#16948=DIRECTION('center_axis',(0.,0.,-1.));
#16949=DIRECTION('ref_axis',(1.,0.,0.));
#16950=DIRECTION('',(0.,0.,-1.));
#16951=DIRECTION('center_axis',(0.,0.,1.));
#16952=DIRECTION('ref_axis',(1.,0.,0.));
#16953=DIRECTION('',(0.,0.,-1.));
#16954=DIRECTION('center_axis',(0.,0.,-1.));
#16955=DIRECTION('ref_axis',(1.,0.,0.));
#16956=DIRECTION('center_axis',(0.,0.,1.));
#16957=DIRECTION('ref_axis',(1.,0.,0.));
#16958=DIRECTION('center_axis',(0.,0.,-1.));
#16959=DIRECTION('ref_axis',(1.,0.,0.));
#16960=DIRECTION('',(0.,0.,-1.));
#16961=DIRECTION('center_axis',(0.,0.,-1.));
#16962=DIRECTION('ref_axis',(1.,0.,0.));
#16963=DIRECTION('',(0.,0.,-1.));
#16964=DIRECTION('center_axis',(0.,0.,-1.));
#16965=DIRECTION('ref_axis',(1.,0.,0.));
#16966=DIRECTION('',(0.,0.,-1.));
#16967=DIRECTION('center_axis',(0.,0.,-1.));
#16968=DIRECTION('ref_axis',(1.,0.,0.));
#16969=DIRECTION('',(0.,0.,-1.));
#16970=DIRECTION('center_axis',(0.,0.,-1.));
#16971=DIRECTION('ref_axis',(1.,0.,0.));
#16972=DIRECTION('',(0.,0.,-1.));
#16973=DIRECTION('center_axis',(0.,0.,-1.));
#16974=DIRECTION('ref_axis',(0.937752268704685,-0.347304884128077,0.));
#16975=DIRECTION('',(0.,0.,-1.));
#16976=DIRECTION('center_axis',(0.,0.,-1.));
#16977=DIRECTION('ref_axis',(1.,0.,0.));
#16978=DIRECTION('center_axis',(0.,0.,-1.));
#16979=DIRECTION('ref_axis',(0.999651918695003,0.0263825974725584,0.));
#16980=DIRECTION('',(1.22464679914735E-16,-1.61260571350473E-30,-1.));
#16981=DIRECTION('center_axis',(0.,0.,1.));
#16982=DIRECTION('ref_axis',(1.,-1.30454602648733E-14,0.));
#16983=DIRECTION('center_axis',(0.,0.,-1.));
#16984=DIRECTION('ref_axis',(1.,-1.30454602648733E-14,0.));
#16985=DIRECTION('',(1.22464679914735E-16,-1.61260571350473E-30,-1.));
#16986=DIRECTION('center_axis',(0.,0.,-1.));
#16987=DIRECTION('ref_axis',(1.,-1.30454602648733E-14,0.));
#16988=DIRECTION('',(1.22464679914735E-16,-1.61260571350473E-30,-1.));
#16989=DIRECTION('center_axis',(0.,0.,-1.));
#16990=DIRECTION('ref_axis',(1.,-1.30454602648733E-14,0.));
#16991=DIRECTION('',(1.22464679914735E-16,-1.61260571350473E-30,-1.));
#16992=DIRECTION('center_axis',(0.,0.,-1.));
#16993=DIRECTION('ref_axis',(1.,-1.30454602648733E-14,0.));
#16994=DIRECTION('',(1.22464679914735E-16,-1.61260571350473E-30,-1.));
#16995=DIRECTION('center_axis',(0.,0.,-1.));
#16996=DIRECTION('ref_axis',(1.,-1.30454602648733E-14,0.));
#16997=DIRECTION('',(1.22464679914735E-16,-1.61260571350473E-30,-1.));
#16998=DIRECTION('center_axis',(0.,0.,-1.));
#16999=DIRECTION('ref_axis',(-0.608776376626888,-0.793341870356681,0.));
#17000=DIRECTION('',(1.22464679914735E-16,-1.61260571350473E-30,-1.));
#17001=DIRECTION('center_axis',(0.,0.,-1.));
#17002=DIRECTION('ref_axis',(1.,-1.30454602648733E-14,0.));
#17003=DIRECTION('center_axis',(0.,0.,-1.));
#17004=DIRECTION('ref_axis',(1.,0.,0.));
#17005=DIRECTION('',(0.,0.,-1.));
#17006=DIRECTION('center_axis',(0.,0.,1.));
#17007=DIRECTION('ref_axis',(1.,0.,0.));
#17008=DIRECTION('',(0.,0.,-1.));
#17009=DIRECTION('center_axis',(0.,0.,-1.));
#17010=DIRECTION('ref_axis',(1.,0.,0.));
#17011=DIRECTION('center_axis',(0.,0.,1.));
#17012=DIRECTION('ref_axis',(1.,0.,0.));
#17013=DIRECTION('center_axis',(0.,0.,-1.));
#17014=DIRECTION('ref_axis',(1.,0.,0.));
#17015=DIRECTION('',(0.,0.,-1.));
#17016=DIRECTION('center_axis',(0.,0.,-1.));
#17017=DIRECTION('ref_axis',(1.,0.,0.));
#17018=DIRECTION('',(0.,0.,-1.));
#17019=DIRECTION('center_axis',(0.,0.,-1.));
#17020=DIRECTION('ref_axis',(1.,0.,0.));
#17021=DIRECTION('',(0.,0.,-1.));
#17022=DIRECTION('center_axis',(0.,0.,-1.));
#17023=DIRECTION('ref_axis',(1.,0.,0.));
#17024=DIRECTION('',(0.,0.,-1.));
#17025=DIRECTION('center_axis',(0.,0.,-1.));
#17026=DIRECTION('ref_axis',(1.,0.,0.));
#17027=DIRECTION('',(0.,0.,-1.));
#17028=DIRECTION('center_axis',(0.,0.,-1.));
#17029=DIRECTION('ref_axis',(0.937752266106258,-0.347304891144047,0.));
#17030=DIRECTION('',(0.,0.,-1.));
#17031=DIRECTION('center_axis',(0.,0.,-1.));
#17032=DIRECTION('ref_axis',(1.,0.,0.));
#17033=DIRECTION('center_axis',(0.,0.,-1.));
#17034=DIRECTION('ref_axis',(0.999651918505729,0.026382604644274,0.));
#17035=DIRECTION('',(1.22464679914735E-16,-2.1451417520641E-30,-1.));
#17036=DIRECTION('center_axis',(0.,0.,1.));
#17037=DIRECTION('ref_axis',(1.,-1.73939470198311E-14,0.));
#17038=DIRECTION('center_axis',(0.,0.,-1.));
#17039=DIRECTION('ref_axis',(1.,-1.73939470198311E-14,0.));
#17040=DIRECTION('',(1.22464679914735E-16,-2.1451417520641E-30,-1.));
#17041=DIRECTION('center_axis',(0.,0.,-1.));
#17042=DIRECTION('ref_axis',(1.,-1.73939470198311E-14,0.));
#17043=DIRECTION('',(1.22464679914735E-16,-2.1451417520641E-30,-1.));
#17044=DIRECTION('center_axis',(0.,0.,-1.));
#17045=DIRECTION('ref_axis',(1.,-1.73939470198311E-14,0.));
#17046=DIRECTION('',(1.22464679914735E-16,-2.1451417520641E-30,-1.));
#17047=DIRECTION('center_axis',(0.,0.,-1.));
#17048=DIRECTION('ref_axis',(1.,-1.73939470198311E-14,0.));
#17049=DIRECTION('',(1.22464679914735E-16,-2.1451417520641E-30,-1.));
#17050=DIRECTION('center_axis',(0.,0.,-1.));
#17051=DIRECTION('ref_axis',(1.,-1.73939470198311E-14,0.));
#17052=DIRECTION('',(1.22464679914735E-16,-2.1451417520641E-30,-1.));
#17053=DIRECTION('center_axis',(0.,0.,-1.));
#17054=DIRECTION('ref_axis',(-0.60877637156726,-0.793341874239222,0.));
#17055=DIRECTION('',(1.22464679914735E-16,-2.1451417520641E-30,-1.));
#17056=DIRECTION('center_axis',(0.,0.,-1.));
#17057=DIRECTION('ref_axis',(1.,-1.73939470198311E-14,0.));
#17058=DIRECTION('center_axis',(0.,0.,1.));
#17059=DIRECTION('ref_axis',(-1.,0.,0.));
#17060=DIRECTION('',(0.,0.,1.));
#17061=DIRECTION('center_axis',(0.,0.,-1.));
#17062=DIRECTION('ref_axis',(-1.,0.,0.));
#17063=DIRECTION('',(0.,0.,1.));
#17064=DIRECTION('center_axis',(0.,0.,-1.));
#17065=DIRECTION('ref_axis',(-1.,0.,0.));
#17066=DIRECTION('center_axis',(0.,0.,1.));
#17067=DIRECTION('ref_axis',(-1.,0.,0.));
#17068=DIRECTION('',(0.,0.,1.));
#17069=DIRECTION('center_axis',(0.,0.,1.));
#17070=DIRECTION('ref_axis',(-1.,0.,0.));
#17071=DIRECTION('',(0.,0.,1.));
#17072=DIRECTION('center_axis',(0.,0.,1.));
#17073=DIRECTION('ref_axis',(-0.937049331551953,-0.349197007773604,0.));
#17074=DIRECTION('',(0.,0.,1.));
#17075=DIRECTION('center_axis',(0.,0.,-1.));
#17076=DIRECTION('ref_axis',(-1.,0.,0.));
#17077=DIRECTION('center_axis',(0.,0.,1.));
#17078=DIRECTION('ref_axis',(0.130209904811036,0.991486450078417,0.));
#17079=DIRECTION('',(-1.22464679914735E-16,1.05158884927822E-30,1.));
#17080=DIRECTION('center_axis',(0.,0.,-1.));
#17081=DIRECTION('ref_axis',(-1.,8.70933927927167E-15,0.));
#17082=DIRECTION('center_axis',(0.,0.,1.));
#17083=DIRECTION('ref_axis',(-1.,8.70933927927167E-15,0.));
#17084=DIRECTION('',(-1.22464679914735E-16,1.05158884927822E-30,1.));
#17085=DIRECTION('center_axis',(0.,0.,1.));
#17086=DIRECTION('ref_axis',(-1.,8.70933927927167E-15,0.));
#17087=DIRECTION('',(-1.22464679914735E-16,1.05158884927822E-30,1.));
#17088=DIRECTION('center_axis',(0.,0.,1.));
#17089=DIRECTION('ref_axis',(-1.,8.70933927927167E-15,0.));
#17090=DIRECTION('',(-1.22464679914735E-16,1.05158884927822E-30,1.));
#17091=DIRECTION('center_axis',(0.,0.,1.));
#17092=DIRECTION('ref_axis',(0.608508670823076,-0.793547224513534,0.));
#17093=DIRECTION('',(-1.22464679914735E-16,1.05158884927822E-30,1.));
#17094=DIRECTION('center_axis',(0.,0.,1.));
#17095=DIRECTION('ref_axis',(-1.,8.70933927927167E-15,0.));
#17096=DIRECTION('center_axis',(0.,0.,1.));
#17097=DIRECTION('ref_axis',(-1.,0.,0.));
#17098=DIRECTION('',(0.,0.,1.));
#17099=DIRECTION('center_axis',(0.,0.,-1.));
#17100=DIRECTION('ref_axis',(-1.,0.,0.));
#17101=DIRECTION('',(0.,0.,1.));
#17102=DIRECTION('center_axis',(0.,0.,-1.));
#17103=DIRECTION('ref_axis',(-1.,0.,0.));
#17104=DIRECTION('center_axis',(0.,0.,1.));
#17105=DIRECTION('ref_axis',(-1.,0.,0.));
#17106=DIRECTION('',(0.,0.,1.));
#17107=DIRECTION('center_axis',(0.,0.,1.));
#17108=DIRECTION('ref_axis',(-1.,0.,0.));
#17109=DIRECTION('',(0.,0.,1.));
#17110=DIRECTION('center_axis',(0.,0.,1.));
#17111=DIRECTION('ref_axis',(-0.937049332084929,-0.349197006343393,0.));
#17112=DIRECTION('',(0.,0.,1.));
#17113=DIRECTION('center_axis',(0.,0.,-1.));
#17114=DIRECTION('ref_axis',(-1.,0.,0.));
#17115=DIRECTION('center_axis',(0.,0.,1.));
#17116=DIRECTION('ref_axis',(0.130209903589588,0.991486450238827,0.));
#17117=DIRECTION('',(-1.22464679914735E-16,8.38271559857251E-31,1.));
#17118=DIRECTION('center_axis',(0.,0.,-1.));
#17119=DIRECTION('ref_axis',(-1.,6.96747142341734E-15,0.));
#17120=DIRECTION('center_axis',(0.,0.,1.));
#17121=DIRECTION('ref_axis',(-1.,6.96747142341734E-15,0.));
#17122=DIRECTION('',(-1.22464679914735E-16,8.38271559857251E-31,1.));
#17123=DIRECTION('center_axis',(0.,0.,1.));
#17124=DIRECTION('ref_axis',(-1.,6.96747142341734E-15,0.));
#17125=DIRECTION('',(-1.22464679914735E-16,8.38271559857251E-31,1.));
#17126=DIRECTION('center_axis',(0.,0.,1.));
#17127=DIRECTION('ref_axis',(-1.,6.96747142341734E-15,0.));
#17128=DIRECTION('',(-1.22464679914735E-16,8.38271559857251E-31,1.));
#17129=DIRECTION('center_axis',(0.,0.,1.));
#17130=DIRECTION('ref_axis',(0.608508660191718,-0.793547232665882,0.));
#17131=DIRECTION('',(-1.22464679914735E-16,8.38271559857251E-31,1.));
#17132=DIRECTION('center_axis',(0.,0.,1.));
#17133=DIRECTION('ref_axis',(-1.,6.96747142341734E-15,0.));
#17134=DIRECTION('center_axis',(0.,0.,1.));
#17135=DIRECTION('ref_axis',(-1.,0.,0.));
#17136=DIRECTION('',(0.,0.,1.));
#17137=DIRECTION('center_axis',(0.,0.,-1.));
#17138=DIRECTION('ref_axis',(-1.,0.,0.));
#17139=DIRECTION('',(0.,0.,1.));
#17140=DIRECTION('center_axis',(0.,0.,-1.));
#17141=DIRECTION('ref_axis',(-1.,0.,0.));
#17142=DIRECTION('center_axis',(0.,0.,1.));
#17143=DIRECTION('ref_axis',(-1.,0.,0.));
#17144=DIRECTION('',(0.,0.,1.));
#17145=DIRECTION('center_axis',(0.,0.,1.));
#17146=DIRECTION('ref_axis',(-1.,0.,0.));
#17147=DIRECTION('',(0.,0.,1.));
#17148=DIRECTION('center_axis',(0.,0.,1.));
#17149=DIRECTION('ref_axis',(-0.937049331749067,-0.34919700724466,0.));
#17150=DIRECTION('',(0.,0.,1.));
#17151=DIRECTION('center_axis',(0.,0.,-1.));
#17152=DIRECTION('ref_axis',(-1.,0.,0.));
#17153=DIRECTION('center_axis',(0.,0.,1.));
#17154=DIRECTION('ref_axis',(0.130209904005025,0.991486450184269,0.));
#17155=DIRECTION('',(-1.22464679914735E-16,1.47822342812015E-30,1.));
#17156=DIRECTION('center_axis',(0.,0.,-1.));
#17157=DIRECTION('ref_axis',(-1.,1.21930749909803E-14,0.));
#17158=DIRECTION('center_axis',(0.,0.,1.));
#17159=DIRECTION('ref_axis',(-1.,1.21930749909803E-14,0.));
#17160=DIRECTION('',(-1.22464679914735E-16,1.47822342812015E-30,1.));
#17161=DIRECTION('center_axis',(0.,0.,1.));
#17162=DIRECTION('ref_axis',(-1.,1.21930749909803E-14,0.));
#17163=DIRECTION('',(-1.22464679914735E-16,1.47822342812015E-30,1.));
#17164=DIRECTION('center_axis',(0.,0.,1.));
#17165=DIRECTION('ref_axis',(-1.,1.21930749909803E-14,0.));
#17166=DIRECTION('',(-1.22464679914735E-16,1.47822342812015E-30,1.));
#17167=DIRECTION('center_axis',(0.,0.,1.));
#17168=DIRECTION('ref_axis',(0.608508666431814,-0.793547227880846,0.));
#17169=DIRECTION('',(-1.22464679914735E-16,1.47822342812015E-30,1.));
#17170=DIRECTION('center_axis',(0.,0.,1.));
#17171=DIRECTION('ref_axis',(-1.,1.21930749909803E-14,0.));
#17172=DIRECTION('center_axis',(0.,0.,1.));
#17173=DIRECTION('ref_axis',(-1.,0.,0.));
#17174=DIRECTION('',(0.,0.,1.));
#17175=DIRECTION('center_axis',(0.,0.,-1.));
#17176=DIRECTION('ref_axis',(-1.,0.,0.));
#17177=DIRECTION('',(0.,0.,1.));
#17178=DIRECTION('center_axis',(0.,0.,-1.));
#17179=DIRECTION('ref_axis',(-1.,0.,0.));
#17180=DIRECTION('center_axis',(0.,0.,1.));
#17181=DIRECTION('ref_axis',(-1.,0.,0.));
#17182=DIRECTION('',(0.,0.,1.));
#17183=DIRECTION('center_axis',(0.,0.,1.));
#17184=DIRECTION('ref_axis',(-1.,0.,0.));
#17185=DIRECTION('',(0.,0.,1.));
#17186=DIRECTION('center_axis',(0.,0.,1.));
#17187=DIRECTION('ref_axis',(-0.937049331905873,-0.349197006823879,0.));
#17188=DIRECTION('',(0.,0.,1.));
#17189=DIRECTION('center_axis',(0.,0.,-1.));
#17190=DIRECTION('ref_axis',(-1.,0.,0.));
#17191=DIRECTION('center_axis',(0.,0.,1.));
#17192=DIRECTION('ref_axis',(0.130209904338333,0.991486450140496,0.));
#17193=DIRECTION('',(-1.22464679914735E-16,1.26490613869919E-30,1.));
#17194=DIRECTION('center_axis',(0.,0.,-1.));
#17195=DIRECTION('ref_axis',(-1.,1.0451207135126E-14,0.));
#17196=DIRECTION('center_axis',(0.,0.,1.));
#17197=DIRECTION('ref_axis',(-1.,1.0451207135126E-14,0.));
#17198=DIRECTION('',(-1.22464679914735E-16,1.26490613869919E-30,1.));
#17199=DIRECTION('center_axis',(0.,0.,1.));
#17200=DIRECTION('ref_axis',(-1.,1.0451207135126E-14,0.));
#17201=DIRECTION('',(-1.22464679914735E-16,1.26490613869919E-30,1.));
#17202=DIRECTION('center_axis',(0.,0.,1.));
#17203=DIRECTION('ref_axis',(-1.,1.0451207135126E-14,0.));
#17204=DIRECTION('',(-1.22464679914735E-16,1.26490613869919E-30,1.));
#17205=DIRECTION('center_axis',(0.,0.,1.));
#17206=DIRECTION('ref_axis',(0.608508664268565,-0.79354722953967,0.));
#17207=DIRECTION('',(-1.22464679914735E-16,1.26490613869919E-30,1.));
#17208=DIRECTION('center_axis',(0.,0.,1.));
#17209=DIRECTION('ref_axis',(-1.,1.0451207135126E-14,0.));
#17210=DIRECTION('center_axis',(0.,0.,1.));
#17211=DIRECTION('ref_axis',(1.,0.,0.));
#17212=DIRECTION('center_axis',(0.,0.,1.));
#17213=DIRECTION('ref_axis',(-1.,1.0451207135126E-14,0.));
#17214=DIRECTION('center_axis',(0.,0.,1.));
#17215=DIRECTION('ref_axis',(-1.,0.,0.));
#17216=DIRECTION('center_axis',(0.,0.,1.));
#17217=DIRECTION('ref_axis',(1.,0.,0.));
#17218=DIRECTION('center_axis',(0.,0.,1.));
#17219=DIRECTION('ref_axis',(-1.,1.21930749909803E-14,0.));
#17220=DIRECTION('center_axis',(0.,0.,1.));
#17221=DIRECTION('ref_axis',(-1.,0.,0.));
#17222=DIRECTION('center_axis',(0.,0.,1.));
#17223=DIRECTION('ref_axis',(1.,0.,0.));
#17224=DIRECTION('center_axis',(0.,0.,1.));
#17225=DIRECTION('ref_axis',(-1.,6.96747142341734E-15,0.));
#17226=DIRECTION('center_axis',(0.,0.,1.));
#17227=DIRECTION('ref_axis',(-1.,0.,0.));
#17228=DIRECTION('center_axis',(0.,0.,1.));
#17229=DIRECTION('ref_axis',(1.,0.,0.));
#17230=DIRECTION('center_axis',(0.,0.,1.));
#17231=DIRECTION('ref_axis',(-1.,8.70933927927167E-15,0.));
#17232=DIRECTION('center_axis',(0.,0.,1.));
#17233=DIRECTION('ref_axis',(-1.,0.,0.));
#17234=DIRECTION('center_axis',(0.,0.,1.));
#17235=DIRECTION('ref_axis',(-1.,0.,0.));
#17236=DIRECTION('center_axis',(0.,0.,1.));
#17237=DIRECTION('ref_axis',(-1.,0.,0.));
#17238=DIRECTION('center_axis',(0.,0.,1.));
#17239=DIRECTION('ref_axis',(-1.,0.,0.));
#17240=DIRECTION('center_axis',(0.,0.,1.));
#17241=DIRECTION('ref_axis',(-1.,0.,0.));
#17242=DIRECTION('center_axis',(0.,0.,1.));
#17243=DIRECTION('ref_axis',(1.,0.,0.));
#17244=DIRECTION('center_axis',(0.,0.,-1.));
#17245=DIRECTION('ref_axis',(1.,-1.73939470198311E-14,0.));
#17246=DIRECTION('center_axis',(0.,0.,-1.));
#17247=DIRECTION('ref_axis',(1.,0.,0.));
#17248=DIRECTION('center_axis',(0.,0.,1.));
#17249=DIRECTION('ref_axis',(1.,0.,0.));
#17250=DIRECTION('center_axis',(0.,0.,-1.));
#17251=DIRECTION('ref_axis',(1.,-1.30454602648733E-14,0.));
#17252=DIRECTION('center_axis',(0.,0.,-1.));
#17253=DIRECTION('ref_axis',(1.,0.,0.));
#17254=DIRECTION('center_axis',(0.,0.,1.));
#17255=DIRECTION('ref_axis',(1.,0.,0.));
#17256=DIRECTION('center_axis',(0.,0.,-1.));
#17257=DIRECTION('ref_axis',(1.,-1.73939470198311E-14,0.));
#17258=DIRECTION('center_axis',(0.,0.,-1.));
#17259=DIRECTION('ref_axis',(1.,0.,0.));
#17260=DIRECTION('center_axis',(0.,0.,1.));
#17261=DIRECTION('ref_axis',(1.,0.,0.));
#17262=DIRECTION('center_axis',(0.,0.,-1.));
#17263=DIRECTION('ref_axis',(1.,-1.30454602648733E-14,0.));
#17264=DIRECTION('center_axis',(0.,0.,-1.));
#17265=DIRECTION('ref_axis',(1.,0.,0.));
#17266=DIRECTION('center_axis',(0.,0.,1.));
#17267=DIRECTION('ref_axis',(1.,0.,0.));
#17268=DIRECTION('center_axis',(0.,0.,1.));
#17269=DIRECTION('ref_axis',(1.,0.,0.));
#17270=DIRECTION('',(0.,0.,-1.));
#17271=DIRECTION('center_axis',(0.,0.,-1.));
#17272=DIRECTION('ref_axis',(1.,0.,0.));
#17273=DIRECTION('center_axis',(0.,0.,1.));
#17274=DIRECTION('ref_axis',(1.,0.,0.));
#17275=DIRECTION('center_axis',(0.,0.,-1.));
#17276=DIRECTION('ref_axis',(1.,0.,0.));
#17277=DIRECTION('center_axis',(0.,0.,1.));
#17278=DIRECTION('ref_axis',(1.,0.,0.));
#17279=DIRECTION('',(0.,0.,-1.));
#17280=DIRECTION('center_axis',(0.,0.,-1.));
#17281=DIRECTION('ref_axis',(1.,0.,0.));
#17282=DIRECTION('center_axis',(0.,0.,1.));
#17283=DIRECTION('ref_axis',(1.,0.,0.));
#17284=DIRECTION('center_axis',(0.,0.,-1.));
#17285=DIRECTION('ref_axis',(1.,0.,0.));
#17286=DIRECTION('',(0.,0.,-1.));
#17287=DIRECTION('center_axis',(0.,0.,-1.));
#17288=DIRECTION('ref_axis',(1.,0.,0.));
#17289=DIRECTION('center_axis',(0.,0.,1.));
#17290=DIRECTION('ref_axis',(1.,0.,0.));
#17291=DIRECTION('center_axis',(0.,0.,1.));
#17292=DIRECTION('ref_axis',(1.,0.,0.));
#31639=CARTESIAN_POINT('',(0.,0.,0.));
#31640=CARTESIAN_POINT('Origin',(-46.,-46.,-5.));
#31641=CARTESIAN_POINT('',(-49.3908050820932,-46.0028114959068,-8.26601780324957));
#31642=CARTESIAN_POINT('',(-49.3955875711091,-46.0001574069683,-8.60898219675042));
#31643=CARTESIAN_POINT('',(-49.38975,-46.,-5.));
#31644=CARTESIAN_POINT('',(-44.696617959125,-42.8708467090881,-9.));
#31645=CARTESIAN_POINT('Ctrl Pts',(-49.3955875711091,-46.0001574069683,
-8.60898219675042));
#31646=CARTESIAN_POINT('Ctrl Pts',(-49.3946782964034,-44.8964214045499,
-8.67403394523185));
#31647=CARTESIAN_POINT('Ctrl Pts',(-48.8034217891345,-43.7921194509379,
-8.73908569371328));
#31648=CARTESIAN_POINT('Ctrl Pts',(-47.8878787982433,-43.1790120886306,
-8.80413744219471));
#31649=CARTESIAN_POINT('Ctrl Pts',(-46.9690175523237,-42.5636826061082,
-8.86942496146314));
#31650=CARTESIAN_POINT('Ctrl Pts',(-45.723514902722,-42.4431146967252,-8.93471248073157));
#31651=CARTESIAN_POINT('Ctrl Pts',(-44.696617959125,-42.8708467090881,-9.));
#31652=CARTESIAN_POINT('',(-49.38975,-46.,-9.));
#31653=CARTESIAN_POINT('Origin',(-46.,-46.,-9.));
#31654=CARTESIAN_POINT('',(-49.38975,-46.,-10.));
#31655=CARTESIAN_POINT('',(-49.38975,-46.,-5.));
#31656=CARTESIAN_POINT('Origin',(-46.,-46.,-10.));
#31657=CARTESIAN_POINT('',(-43.1019982053025,-47.7690579931343,-9.));
#31658=CARTESIAN_POINT('Origin',(-46.,-46.,-9.));
#31659=CARTESIAN_POINT('Ctrl Pts',(-43.1019720879323,-47.7690801693092,
-9.));
#31660=CARTESIAN_POINT('Ctrl Pts',(-42.5564934135711,-46.8680833947406,
-8.9379383670794));
#31661=CARTESIAN_POINT('Ctrl Pts',(-42.4589272462208,-45.6899359380158,
-8.87587673415881));
#31662=CARTESIAN_POINT('Ctrl Pts',(-42.857579160951,-44.7152009935522,-8.81381510123821));
#31663=CARTESIAN_POINT('Ctrl Pts',(-43.2769525054721,-43.6898005412357,
-8.74852758196978));
#31664=CARTESIAN_POINT('Ctrl Pts',(-44.2454702047504,-42.8895084371012,
-8.68324006270134));
#31665=CARTESIAN_POINT('Ctrl Pts',(-45.3313096516499,-42.6714409964239,
-8.61795254343291));
#31666=CARTESIAN_POINT('Ctrl Pts',(-46.4171490985494,-42.4533735557466,
-8.55266502416448));
#31667=CARTESIAN_POINT('Ctrl Pts',(-47.6203102930703,-42.8175307785264,
-8.48737750489605));
#31668=CARTESIAN_POINT('Ctrl Pts',(-48.4028923648305,-43.6014277710615,
-8.42208998562762));
#31669=CARTESIAN_POINT('Ctrl Pts',(-49.0264893054514,-44.2260725002811,
-8.37006592483494));
#31670=CARTESIAN_POINT('Ctrl Pts',(-49.3830342221214,-45.1172362956638,
-8.31804186404226));
#31671=CARTESIAN_POINT('Ctrl Pts',(-49.3908050820932,-46.0028114959068,
-8.26601780324957));
#31672=CARTESIAN_POINT('Origin',(-46.,-46.,-5.));
#31673=CARTESIAN_POINT('',(-49.3915791156511,-45.9973272796015,-7.01601780324957));
#31674=CARTESIAN_POINT('',(-49.3858576553579,-45.9980711564067,-7.35898219675043));
#31675=CARTESIAN_POINT('',(-49.38975,-46.,-5.));
#31676=CARTESIAN_POINT('Ctrl Pts',(-49.3858576553579,-45.9980711564067,
-7.35898219675043));
#31677=CARTESIAN_POINT('Ctrl Pts',(-49.3881113941792,-45.5759581157443,
-7.3836879770195));
#31678=CARTESIAN_POINT('Ctrl Pts',(-49.3147699482676,-45.154598996582,-7.40839375728857));
#31679=CARTESIAN_POINT('Ctrl Pts',(-49.1621982248071,-44.7642017499235,
-7.43309953755765));
#31680=CARTESIAN_POINT('Ctrl Pts',(-48.7590120381433,-43.7325376014544,
-7.49838705682608));
#31681=CARTESIAN_POINT('Ctrl Pts',(-47.8025338878601,-42.9170907346222,
-7.56367457609451));
#31682=CARTESIAN_POINT('Ctrl Pts',(-46.7201047416051,-42.6821547425348,
-7.62896209536294));
#31683=CARTESIAN_POINT('Ctrl Pts',(-45.63767559535,-42.4472187504474,-7.69424961463137));
#31684=CARTESIAN_POINT('Ctrl Pts',(-44.4292954531231,-42.7927936331048,
-7.7595371338998));
#31685=CARTESIAN_POINT('Ctrl Pts',(-43.6346772179205,-43.5644833691861,
-7.82482465316823));
#31686=CARTESIAN_POINT('Ctrl Pts',(-42.840058982718,-44.3361731052674,-7.89011217243666));
#31687=CARTESIAN_POINT('Ctrl Pts',(-42.4592026545397,-45.5339776947726,
-7.9553996917051));
#31688=CARTESIAN_POINT('Ctrl Pts',(-42.6624687214266,-46.622835827247,-8.02068721097353));
#31689=CARTESIAN_POINT('Ctrl Pts',(-42.8657347883135,-47.7116939597214,
-8.08597473024196));
#31690=CARTESIAN_POINT('Ctrl Pts',(-43.6531232502656,-48.691605635165,-8.15126224951039));
#31691=CARTESIAN_POINT('Ctrl Pts',(-44.6724331904996,-49.1247427427676,
-8.21654976877882));
#31692=CARTESIAN_POINT('Ctrl Pts',(-45.6917431307337,-49.5578798503701,
-8.28183728804725));
#31693=CARTESIAN_POINT('Ctrl Pts',(-46.9429745492497,-49.4442423901316,
-8.34712480731569));
#31694=CARTESIAN_POINT('Ctrl Pts',(-47.8680858853197,-48.8347434521096,
-8.41241232658412));
#31695=CARTESIAN_POINT('Ctrl Pts',(-48.7931972213897,-48.2252445140876,
-8.47769984585255));
#31696=CARTESIAN_POINT('Ctrl Pts',(-49.3921884750137,-47.1198840982822,
-8.54298736512098));
#31697=CARTESIAN_POINT('Ctrl Pts',(-49.395574180707,-46.0121583625486,-8.60827488438941));
#31698=CARTESIAN_POINT('Ctrl Pts',(-49.3955864074006,-46.0081580670644,
-8.60851065517641));
#31699=CARTESIAN_POINT('Ctrl Pts',(-49.3955908666456,-46.0041577407335,
-8.60874642596342));
#31700=CARTESIAN_POINT('Ctrl Pts',(-49.3955875711091,-46.0001574069683,
-8.60898219675042));
#31701=CARTESIAN_POINT('Ctrl Pts',(-49.3908050820932,-46.0028114959068,
-8.26601780324957));
#31702=CARTESIAN_POINT('Ctrl Pts',(-49.3927862515173,-46.2285876025122,
-8.25275434477382));
#31703=CARTESIAN_POINT('Ctrl Pts',(-49.3720975399661,-46.4540004573671,
-8.23949088629807));
#31704=CARTESIAN_POINT('Ctrl Pts',(-49.3273847039345,-46.6745408721824,
-8.22622742782233));
#31705=CARTESIAN_POINT('Ctrl Pts',(-49.1072920222784,-47.7601202184779,
-8.1609399085539));
#31706=CARTESIAN_POINT('Ctrl Pts',(-48.3051037099665,-48.7276421487786,
-8.09565238928547));
#31707=CARTESIAN_POINT('Ctrl Pts',(-47.2790835032418,-49.1449315523856,
-8.03036487001703));
#31708=CARTESIAN_POINT('Ctrl Pts',(-46.2530632965171,-49.5622209559926,
-7.9650773507486));
#31709=CARTESIAN_POINT('Ctrl Pts',(-45.0032111953795,-49.4292778329058,
-7.89978983148017));
#31710=CARTESIAN_POINT('Ctrl Pts',(-44.0879228271742,-48.805469104904,-7.83450231221174));
#31711=CARTESIAN_POINT('Ctrl Pts',(-43.1726344589688,-48.1816603769021,
-7.76921479294331));
#31712=CARTESIAN_POINT('Ctrl Pts',(-42.5919098236955,-47.0669860439851,
-7.70392727367488));
#31713=CARTESIAN_POINT('Ctrl Pts',(-42.6051529380119,-45.9594166616959,
-7.63863975440645));
#31714=CARTESIAN_POINT('Ctrl Pts',(-42.6183960523284,-44.8518472794067,
-7.57335223513802));
#31715=CARTESIAN_POINT('Ctrl Pts',(-43.2256069162345,-43.7513828477454,
-7.50806471586959));
#31716=CARTESIAN_POINT('Ctrl Pts',(-44.155537258283,-43.149629262965,-7.44277719660115));
#31717=CARTESIAN_POINT('Ctrl Pts',(-45.0854676003314,-42.5478756781846,
-7.37748967733272));
#31718=CARTESIAN_POINT('Ctrl Pts',(-46.3381174205223,-42.4448329402852,
-7.31220215806429));
#31719=CARTESIAN_POINT('Ctrl Pts',(-47.3538838078074,-42.8865360920784,
-7.24691463879586));
#31720=CARTESIAN_POINT('Ctrl Pts',(-48.3696501950926,-43.3282392438716,
-7.18162711952743));
#31721=CARTESIAN_POINT('Ctrl Pts',(-49.1485331494721,-44.3146882853574,
-7.116339600259));
#31722=CARTESIAN_POINT('Ctrl Pts',(-49.3425844160128,-45.4052047263581,
-7.05105208099057));
#31723=CARTESIAN_POINT('Ctrl Pts',(-49.3772947049224,-45.6002673064819,
-7.03937398841023));
#31724=CARTESIAN_POINT('Ctrl Pts',(-49.3932932445553,-45.7986595336273,
-7.0276958958299));
#31725=CARTESIAN_POINT('Ctrl Pts',(-49.3915791156511,-45.9973272796015,
-7.01601780324957));
#31726=CARTESIAN_POINT('Origin',(-46.,-46.,-5.));
#31727=CARTESIAN_POINT('',(-49.3849269836833,-46.0010327956957,-5.76601780324957));
#31728=CARTESIAN_POINT('',(-49.3896326160374,-46.0028925919798,-6.10898219675042));
#31729=CARTESIAN_POINT('',(-49.38975,-46.,-5.));
#31730=CARTESIAN_POINT('Ctrl Pts',(-49.3896326160374,-46.0028925919798,
-6.10898219675042));
#31731=CARTESIAN_POINT('Ctrl Pts',(-49.3822316042023,-45.1570406462268,
-6.15862952807558));
#31732=CARTESIAN_POINT('Ctrl Pts',(-49.0605617986376,-44.3061622980437,
-6.20827685940073));
#31733=CARTESIAN_POINT('Ctrl Pts',(-48.4872408503176,-43.6890939238723,
-6.25792419072589));
#31734=CARTESIAN_POINT('Ctrl Pts',(-47.7333090384487,-42.8776331203741,
-6.32321170999432));
#31735=CARTESIAN_POINT('Ctrl Pts',(-46.5441987345435,-42.470498205483,-6.38849922926275));
#31736=CARTESIAN_POINT('Ctrl Pts',(-45.4511228720662,-42.6495690045761,
-6.45378674853118));
#31737=CARTESIAN_POINT('Ctrl Pts',(-44.3580470095889,-42.8286398036693,
-6.51907426779961));
#31738=CARTESIAN_POINT('Ctrl Pts',(-43.3610055885394,-43.5939163167467,
-6.58436178706804));
#31739=CARTESIAN_POINT('Ctrl Pts',(-42.9054062548915,-44.6035257121301,
-6.64964930633647));
#31740=CARTESIAN_POINT('Ctrl Pts',(-42.4498069212435,-45.6131351075136,
-6.71493682560491));
#31741=CARTESIAN_POINT('Ctrl Pts',(-42.5356496749971,-46.8670773852031,
-6.78022434487333));
#31742=CARTESIAN_POINT('Ctrl Pts',(-43.1245889322668,-47.8051783725204,
-6.84551186414177));
#31743=CARTESIAN_POINT('Ctrl Pts',(-43.7135281895365,-48.7432793598376,
-6.9107993834102));
#31744=CARTESIAN_POINT('Ctrl Pts',(-44.8055639503223,-49.3655390567825,
-6.97608690267863));
#31745=CARTESIAN_POINT('Ctrl Pts',(-45.9128440217905,-49.3939739060678,
-7.04137442194706));
#31746=CARTESIAN_POINT('Ctrl Pts',(-47.0201240932587,-49.4224087553532,
-7.10666194121549));
#31747=CARTESIAN_POINT('Ctrl Pts',(-48.1426484754094,-48.857018756979,-7.17194946048392));
#31748=CARTESIAN_POINT('Ctrl Pts',(-48.7789635549624,-47.9503830427389,
-7.23723697975236));
#31749=CARTESIAN_POINT('Ctrl Pts',(-49.174487427965,-47.3868319331997,-7.27781871875171));
#31750=CARTESIAN_POINT('Ctrl Pts',(-49.3821556617506,-46.6914344526808,
-7.31840045775107));
#31751=CARTESIAN_POINT('Ctrl Pts',(-49.3858576553579,-45.9980711564067,
-7.35898219675043));
#31752=CARTESIAN_POINT('Ctrl Pts',(-49.3915791156511,-45.9973272796015,
-7.01601780324957));
#31753=CARTESIAN_POINT('Ctrl Pts',(-49.3837102391892,-46.909331007079,-6.96240837656147));
#31754=CARTESIAN_POINT('Ctrl Pts',(-49.0025718726505,-47.8271409050093,
-6.90879894987337));
#31755=CARTESIAN_POINT('Ctrl Pts',(-48.3448154570193,-48.4552994801616,
-6.85518952318527));
#31756=CARTESIAN_POINT('Ctrl Pts',(-47.5437756527831,-49.2202939524488,
-6.78990200391684));
#31757=CARTESIAN_POINT('Ctrl Pts',(-46.3324764656086,-49.5556990565077,
-6.72461448464841));
#31758=CARTESIAN_POINT('Ctrl Pts',(-45.2520432244852,-49.3116786847004,
-6.65932696537998));
#31759=CARTESIAN_POINT('Ctrl Pts',(-44.1716099833619,-49.0676583128931,
-6.59403944611155));
#31760=CARTESIAN_POINT('Ctrl Pts',(-43.2220426882898,-48.2442124652195,
-6.52875192684312));
#31761=CARTESIAN_POINT('Ctrl Pts',(-42.8275419844485,-47.209199926625,-6.46346440757469));
#31762=CARTESIAN_POINT('Ctrl Pts',(-42.4330412806072,-46.1741873880306,
-6.39817688830626));
#31763=CARTESIAN_POINT('Ctrl Pts',(-42.5936071679967,-44.9276081585153,
-6.33288936903782));
#31764=CARTESIAN_POINT('Ctrl Pts',(-43.2375100754716,-44.026347513733,-6.26760184976939));
#31765=CARTESIAN_POINT('Ctrl Pts',(-43.8814129829466,-43.1250868689506,
-6.20231433050096));
#31766=CARTESIAN_POINT('Ctrl Pts',(-45.008652910507,-42.5691448089011,-6.13702681123253));
#31767=CARTESIAN_POINT('Ctrl Pts',(-46.1156569734068,-42.6068778178316,
-6.0717392919641));
#31768=CARTESIAN_POINT('Ctrl Pts',(-47.2226610363066,-42.6446108267621,
-6.00645177269567));
#31769=CARTESIAN_POINT('Ctrl Pts',(-48.3094292345459,-43.2760189046725,
-5.94116425342724));
#31770=CARTESIAN_POINT('Ctrl Pts',(-48.8904687669622,-44.2190325906619,
-5.87587673415881));
#31771=CARTESIAN_POINT('Ctrl Pts',(-49.2163727200328,-44.7479671483254,
-5.83925709052239));
#31772=CARTESIAN_POINT('Ctrl Pts',(-49.383171073577,-45.3749349013358,-5.80263744688598));
#31773=CARTESIAN_POINT('Ctrl Pts',(-49.3849269836833,-46.0010327956957,
-5.76601780324957));
#31774=CARTESIAN_POINT('Origin',(-46.,-46.,-5.));
#31775=CARTESIAN_POINT('',(-49.3946337481228,-46.0010845676627,-4.51601780324957));
#31776=CARTESIAN_POINT('',(-49.3926793474262,-45.9976551524526,-4.85898219675043));
#31777=CARTESIAN_POINT('',(-49.38975,-46.,-5.));
#31778=CARTESIAN_POINT('Ctrl Pts',(-49.3926793474262,-45.9976551524526,
-4.85898219675043));
#31779=CARTESIAN_POINT('Ctrl Pts',(-49.3939351810614,-45.8395538986053,
-4.86828355986323));
#31780=CARTESIAN_POINT('Ctrl Pts',(-49.3838123532219,-45.6816141300476,
-4.87758492297603));
#31781=CARTESIAN_POINT('Ctrl Pts',(-49.3617510816055,-45.5253599306122,
-4.88688628608883));
#31782=CARTESIAN_POINT('Ctrl Pts',(-49.206900047593,-44.4285906794074,-4.95217380535726));
#31783=CARTESIAN_POINT('Ctrl Pts',(-48.4638627815182,-43.4148664690314,
-5.0174613246257));
#31784=CARTESIAN_POINT('Ctrl Pts',(-47.4645769192664,-42.9370491377502,
-5.08274884389413));
#31785=CARTESIAN_POINT('Ctrl Pts',(-46.4652910570147,-42.459231806469,-5.14803636316256));
#31786=CARTESIAN_POINT('Ctrl Pts',(-45.2097565985859,-42.5173213542825,
-5.21332388243099));
#31787=CARTESIAN_POINT('Ctrl Pts',(-44.2588594812185,-43.0853673919219,
-5.27861140169942));
#31788=CARTESIAN_POINT('Ctrl Pts',(-43.307962363851,-43.6534134295613,-5.34389892096785));
#31789=CARTESIAN_POINT('Ctrl Pts',(-42.6617025875449,-44.7314159570266,
-5.40918644023628));
#31790=CARTESIAN_POINT('Ctrl Pts',(-42.6087842862726,-45.8377980273576,
-5.47447395950471));
#31791=CARTESIAN_POINT('Ctrl Pts',(-42.5558659850004,-46.9441800976885,
-5.53976147877314));
#31792=CARTESIAN_POINT('Ctrl Pts',(-43.0962891587621,-48.0789417108851,
-5.60504899804157));
#31793=CARTESIAN_POINT('Ctrl Pts',(-43.9886301660516,-48.7351498973253,
-5.67033651731001));
#31794=CARTESIAN_POINT('Ctrl Pts',(-44.8809711733411,-49.3913580837655,
-5.73562403657844));
#31795=CARTESIAN_POINT('Ctrl Pts',(-46.1252300141585,-49.5690128434493,
-5.80091155584687));
#31796=CARTESIAN_POINT('Ctrl Pts',(-47.1655578423799,-49.1887503080326,
-5.8661990751153));
#31797=CARTESIAN_POINT('Ctrl Pts',(-48.2058856706013,-48.8084877726158,
-5.93148659438373));
#31798=CARTESIAN_POINT('Ctrl Pts',(-49.0422824862267,-47.8703079420985,
-5.99677411365216));
#31799=CARTESIAN_POINT('Ctrl Pts',(-49.3011042341231,-46.7933246807872,
-6.06206163292059));
#31800=CARTESIAN_POINT('Ctrl Pts',(-49.3631072145742,-46.5353240581962,
-6.07770182086387));
#31801=CARTESIAN_POINT('Ctrl Pts',(-49.3919641253649,-46.2693577382557,
-6.09334200880715));
#31802=CARTESIAN_POINT('Ctrl Pts',(-49.3896326160374,-46.0028925919798,
-6.10898219675042));
#31803=CARTESIAN_POINT('Ctrl Pts',(-49.3849269836833,-46.0010327956957,
-5.76601780324957));
#31804=CARTESIAN_POINT('Ctrl Pts',(-49.3863016069059,-46.4911767399457,
-5.73734992761755));
#31805=CARTESIAN_POINT('Ctrl Pts',(-49.2865279643948,-46.980787580758,-5.70868205198553));
#31806=CARTESIAN_POINT('Ctrl Pts',(-49.0827576637059,-47.4224133864494,
-5.68001417635351));
#31807=CARTESIAN_POINT('Ctrl Pts',(-48.61869616144,-48.428161202179,-5.61472665708508));
#31808=CARTESIAN_POINT('Ctrl Pts',(-47.6152622903149,-49.1850375395698,
-5.54943913781665));
#31809=CARTESIAN_POINT('Ctrl Pts',(-46.5207208867884,-49.354922414,-5.48415161854822));
#31810=CARTESIAN_POINT('Ctrl Pts',(-45.426179483262,-49.5248072884302,-5.41886409927979));
#31811=CARTESIAN_POINT('Ctrl Pts',(-44.2405305473341,-49.1077006998998,
-5.35357658001135));
#31812=CARTESIAN_POINT('Ctrl Pts',(-43.4934399857245,-48.2899370152651,
-5.28828906074292));
#31813=CARTESIAN_POINT('Ctrl Pts',(-42.7463494241149,-47.4721733306304,
-5.22300154147449));
#31814=CARTESIAN_POINT('Ctrl Pts',(-42.4378172368234,-46.2537525498914,
-5.15771402220606));
#31815=CARTESIAN_POINT('Ctrl Pts',(-42.7056742603893,-45.1789807759279,
-5.09242650293763));
#31816=CARTESIAN_POINT('Ctrl Pts',(-42.9735312839552,-44.1042090019644,
-5.0271389836692));
#31817=CARTESIAN_POINT('Ctrl Pts',(-43.8177775183786,-43.1730862347763,
-4.96185146440077));
#31818=CARTESIAN_POINT('Ctrl Pts',(-44.8612621572759,-42.801573704276,-4.89656394513234));
#31819=CARTESIAN_POINT('Ctrl Pts',(-45.9047467961732,-42.4300611737756,
-4.83127642586391));
#31820=CARTESIAN_POINT('Ctrl Pts',(-47.1474698395444,-42.618158879963,-4.76598890659548));
#31821=CARTESIAN_POINT('Ctrl Pts',(-48.0342686144742,-43.2818377814125,
-4.70070138732704));
#31822=CARTESIAN_POINT('Ctrl Pts',(-48.8704528139696,-43.9076368089027,
-4.63914019263455));
#31823=CARTESIAN_POINT('Ctrl Pts',(-49.3901824623747,-44.9562781289759,
-4.57757899794206));
#31824=CARTESIAN_POINT('Ctrl Pts',(-49.3946337481228,-46.0010845676627,
-4.51601780324957));
#31825=CARTESIAN_POINT('Origin',(-46.,-46.,-5.));
#31826=CARTESIAN_POINT('',(-49.3870908106244,-45.9974837229373,-3.26601780324957));
#31827=CARTESIAN_POINT('',(-49.3846593199306,-46.0004230001441,-3.60898219675043));
#31828=CARTESIAN_POINT('',(-49.38975,-46.,-5.));
#31829=CARTESIAN_POINT('Ctrl Pts',(-49.3846593199306,-46.0004230001441,
-3.60898219675043));
#31830=CARTESIAN_POINT('Ctrl Pts',(-49.3839900131623,-45.4148448050876,
-3.64322511091931));
#31831=CARTESIAN_POINT('Ctrl Pts',(-49.2392620998284,-44.8289567285941,
-3.67746802508819));
#31832=CARTESIAN_POINT('Ctrl Pts',(-48.9524290200888,-44.3237492993344,
-3.71171093925707));
#31833=CARTESIAN_POINT('Ctrl Pts',(-48.4055532452068,-43.3605211228516,
-3.7769984585255));
#31834=CARTESIAN_POINT('Ctrl Pts',(-47.3421079624348,-42.6905768803167,
-3.84228597779393));
#31835=CARTESIAN_POINT('Ctrl Pts',(-46.2371669440815,-42.6132013085067,
-3.90757349706236));
#31836=CARTESIAN_POINT('Ctrl Pts',(-45.1322259257282,-42.5358257366966,
-3.97286101633079));
#31837=CARTESIAN_POINT('Ctrl Pts',(-43.9857891717937,-43.0510188356115,
-4.03814853559923));
#31838=CARTESIAN_POINT('Ctrl Pts',(-43.3100053044936,-43.9286279733269,
-4.10343605486766));
#31839=CARTESIAN_POINT('Ctrl Pts',(-42.6342214371935,-44.8062371110423,
-4.16872357413609));
#31840=CARTESIAN_POINT('Ctrl Pts',(-42.4290904565277,-46.0462622875582,
-4.23401109340452));
#31841=CARTESIAN_POINT('Ctrl Pts',(-42.7862506912548,-47.0947460500201,
-4.29929861267295));
#31842=CARTESIAN_POINT('Ctrl Pts',(-43.1434109259818,-48.143229812482,-4.36458613194138));
#31843=CARTESIAN_POINT('Ctrl Pts',(-44.0628623761017,-49.0001721608899,
-4.42987365120981));
#31844=CARTESIAN_POINT('Ctrl Pts',(-45.1338577500445,-49.2827505445249,
-4.49516117047825));
#31845=CARTESIAN_POINT('Ctrl Pts',(-46.2048531239873,-49.56532892816,-4.56044868974668));
#31846=CARTESIAN_POINT('Ctrl Pts',(-47.427392421753,-49.2735433470222,-4.62573620901511));
#31847=CARTESIAN_POINT('Ctrl Pts',(-48.2553296696607,-48.5377434104365,
-4.69102372828354));
#31848=CARTESIAN_POINT('Ctrl Pts',(-48.9653125969923,-47.9067712030286,
-4.74700988443917));
#31849=CARTESIAN_POINT('Ctrl Pts',(-49.3851203157927,-46.9492878732649,
-4.8029960405948));
#31850=CARTESIAN_POINT('Ctrl Pts',(-49.3926793474262,-45.9976551524526,
-4.85898219675043));
#31851=CARTESIAN_POINT('Ctrl Pts',(-49.3946337481228,-46.0010845676627,
-4.51601780324957));
#31852=CARTESIAN_POINT('Ctrl Pts',(-49.3949031862901,-46.0643271335198,
-4.51229147867363));
#31853=CARTESIAN_POINT('Ctrl Pts',(-49.3932846801065,-46.1275556486361,
-4.50856515409769));
#31854=CARTESIAN_POINT('Ctrl Pts',(-49.3897341345749,-46.1906754848652,
-4.50483882952175));
#31855=CARTESIAN_POINT('Ctrl Pts',(-49.3275263732576,-47.2965741901566,
-4.43955131025332));
#31856=CARTESIAN_POINT('Ctrl Pts',(-48.6722363441346,-48.3691115040278,
-4.37426379098489));
#31857=CARTESIAN_POINT('Ctrl Pts',(-47.7166022939084,-48.9291519608081,
-4.30897627171646));
#31858=CARTESIAN_POINT('Ctrl Pts',(-46.7609682436823,-49.4891924175884,
-4.24368875244803));
#31859=CARTESIAN_POINT('Ctrl Pts',(-45.504990172353,-49.5367360172778,-4.1784012331796));
#31860=CARTESIAN_POINT('Ctrl Pts',(-44.5097521823566,-49.0505435714074,
-4.11311371391116));
#31861=CARTESIAN_POINT('Ctrl Pts',(-43.5145141923602,-48.564351125537,-4.04782619464273));
#31862=CARTESIAN_POINT('Ctrl Pts',(-42.7800162836966,-47.5444226341068,
-3.9825386753743));
#31863=CARTESIAN_POINT('Ctrl Pts',(-42.6343813038521,-46.4463915747831,
-3.91725115610587));
#31864=CARTESIAN_POINT('Ctrl Pts',(-42.4887463240076,-45.3483605154594,
-3.85196363683744));
#31865=CARTESIAN_POINT('Ctrl Pts',(-42.9319742729821,-44.1722268882422,
-3.78667611756901));
#31866=CARTESIAN_POINT('Ctrl Pts',(-43.766061567924,-43.4434058326004,-3.72138859830058));
#31867=CARTESIAN_POINT('Ctrl Pts',(-44.6001488628658,-42.7145847769586,
-3.65610107903215));
#31868=CARTESIAN_POINT('Ctrl Pts',(-45.8250955037749,-42.4330762928922,
-3.59081355976371));
#31869=CARTESIAN_POINT('Ctrl Pts',(-46.8936800870826,-42.724638873672,-3.52552604049528));
#31870=CARTESIAN_POINT('Ctrl Pts',(-47.9622646703903,-43.0162014544519,
-3.46023852122685));
#31871=CARTESIAN_POINT('Ctrl Pts',(-48.8744871960966,-43.880835100078,-3.39495100195842));
#31872=CARTESIAN_POINT('Ctrl Pts',(-49.2228297485814,-44.9322813618375,
-3.32966348268999));
#31873=CARTESIAN_POINT('Ctrl Pts',(-49.3360239122814,-45.2739495830363,
-3.30844825620985));
#31874=CARTESIAN_POINT('Ctrl Pts',(-49.3896763141562,-45.6353439034476,
-3.28723302972971));
#31875=CARTESIAN_POINT('Ctrl Pts',(-49.3870908106244,-45.9974837229373,
-3.26601780324957));
#31876=CARTESIAN_POINT('Origin',(-46.,-46.,-5.));
#31877=CARTESIAN_POINT('',(-49.3879806100937,-46.0027475395409,-2.01601780324957));
#31878=CARTESIAN_POINT('',(-49.393944259473,-46.0016943208402,-2.35898219675043));
#31879=CARTESIAN_POINT('',(-49.38975,-46.,-5.));
#31880=CARTESIAN_POINT('Ctrl Pts',(-49.393944259473,-46.0016943208402,-2.35898219675043));
#31881=CARTESIAN_POINT('Ctrl Pts',(-49.3877066726979,-44.9966831864109,
-2.41816666197539));
#31882=CARTESIAN_POINT('Ctrl Pts',(-48.9121874363056,-43.9865344276296,
-2.47735112720035));
#31883=CARTESIAN_POINT('Ctrl Pts',(-48.1303608079629,-43.3564765857691,
-2.53653559242531));
#31884=CARTESIAN_POINT('Ctrl Pts',(-47.2679128519243,-42.6614476903598,
-2.60182311169374));
#31885=CARTESIAN_POINT('Ctrl Pts',(-46.0327280241684,-42.4289407681851,
-2.66711063096217));
#31886=CARTESIAN_POINT('Ctrl Pts',(-44.9766013247455,-42.7628239525169,
-2.7323981502306));
#31887=CARTESIAN_POINT('Ctrl Pts',(-43.9204746253226,-43.0967071368487,
-2.79768566949903));
#31888=CARTESIAN_POINT('Ctrl Pts',(-43.0434060542328,-43.9969804276871,
-2.86297318876746));
#31889=CARTESIAN_POINT('Ctrl Pts',(-42.7372092246985,-45.0614639450911,
-2.9282607080359));
#31890=CARTESIAN_POINT('Ctrl Pts',(-42.4310123951642,-46.1259474624951,
-2.99354822730433));
#31891=CARTESIAN_POINT('Ctrl Pts',(-42.6956873071853,-47.3546412064646,
-3.05883574657276));
#31892=CARTESIAN_POINT('Ctrl Pts',(-43.4129954937812,-48.1986498542888,
-3.12412326584119));
#31893=CARTESIAN_POINT('Ctrl Pts',(-44.1303036803771,-49.0426585021129,
-3.18941078510962));
#31894=CARTESIAN_POINT('Ctrl Pts',(-45.3002451415477,-49.5019820537916,
-3.25469830437805));
#31895=CARTESIAN_POINT('Ctrl Pts',(-46.4001709931723,-49.371426511499,-3.31998582364648));
#31896=CARTESIAN_POINT('Ctrl Pts',(-47.500096844797,-49.2408709692064,-3.38527334291492));
#31897=CARTESIAN_POINT('Ctrl Pts',(-48.5300070868757,-48.5204363329426,
-3.45056086218335));
#31898=CARTESIAN_POINT('Ctrl Pts',(-49.0298090744191,-47.5319629595953,
-3.51584838145178));
#31899=CARTESIAN_POINT('Ctrl Pts',(-49.2674679027085,-47.0619379705799,
-3.54689298655133));
#31900=CARTESIAN_POINT('Ctrl Pts',(-49.3852661130384,-46.5313078346175,
-3.57793759165088));
#31901=CARTESIAN_POINT('Ctrl Pts',(-49.3846593199306,-46.0004230001441,
-3.60898219675043));
#31902=CARTESIAN_POINT('Ctrl Pts',(-49.3870908106244,-45.9974837229373,
-3.26601780324957));
#31903=CARTESIAN_POINT('Ctrl Pts',(-49.3817197122406,-46.749789250752,-3.22194551046128));
#31904=CARTESIAN_POINT('Ctrl Pts',(-49.1336512376201,-47.5053120155708,
-3.17787321767299));
#31905=CARTESIAN_POINT('Ctrl Pts',(-48.6725047066197,-48.0938895178028,
-3.1338009248847));
#31906=CARTESIAN_POINT('Ctrl Pts',(-47.9893745329099,-48.9657925341156,
-3.06851340561626));
#31907=CARTESIAN_POINT('Ctrl Pts',(-46.838651606227,-49.4713396888484,-3.00322588634783));
#31908=CARTESIAN_POINT('Ctrl Pts',(-45.734399285881,-49.38468766412,-2.9379383670794));
#31909=CARTESIAN_POINT('Ctrl Pts',(-44.630146965535,-49.2980356393917,-2.87265084781097));
#31910=CARTESIAN_POINT('Ctrl Pts',(-43.572365251526,-48.6191844352022,-2.80736332854254));
#31911=CARTESIAN_POINT('Ctrl Pts',(-43.0335978832048,-47.651397447682,-2.74207580927411));
#31912=CARTESIAN_POINT('Ctrl Pts',(-42.4948305148836,-46.6836104601617,
-2.67678829000568));
#31913=CARTESIAN_POINT('Ctrl Pts',(-42.4750774922503,-45.4268876893108,
-2.61150077073725));
#31914=CARTESIAN_POINT('Ctrl Pts',(-42.9831629846654,-44.4426466400763,
-2.54621325146882));
#31915=CARTESIAN_POINT('Ctrl Pts',(-43.4912484770806,-43.4584055908418,
-2.48092573220038));
#31916=CARTESIAN_POINT('Ctrl Pts',(-44.5271724845442,-42.7466462632239,
-2.41563821293195));
#31917=CARTESIAN_POINT('Ctrl Pts',(-45.6281560686778,-42.6253320035213,
-2.35035069366352));
#31918=CARTESIAN_POINT('Ctrl Pts',(-46.7291396528114,-42.5040177438187,
-2.28506317439509));
#31919=CARTESIAN_POINT('Ctrl Pts',(-47.895182813615,-42.9731485520315,-2.21977565512666));
#31920=CARTESIAN_POINT('Ctrl Pts',(-48.6053776654248,-43.8231522580853,
-2.15448813585823));
#31921=CARTESIAN_POINT('Ctrl Pts',(-49.1074691240937,-44.4240853675818,
-2.10833135832201));
#31922=CARTESIAN_POINT('Ctrl Pts',(-49.38172005634,-45.2153850526079,-2.06217458078579));
#31923=CARTESIAN_POINT('Ctrl Pts',(-49.3879806100937,-46.0027475395409,
-2.01601780324957));
#31924=CARTESIAN_POINT('Origin',(-46.,-46.,-5.));
#31925=CARTESIAN_POINT('',(-49.3940299756876,-45.9984545908008,-0.766017803249567));
#31926=CARTESIAN_POINT('',(-49.3881103126091,-45.9972329022571,-1.10898219675043));
#31927=CARTESIAN_POINT('',(-49.38975,-46.,-5.));
#31928=CARTESIAN_POINT('',(-43.4267655729853,-43.7934484719077,0.));
#31929=CARTESIAN_POINT('Ctrl Pts',(-49.3940299756876,-45.9984545908008,
-0.766017803249567));
#31930=CARTESIAN_POINT('Ctrl Pts',(-49.3879993454613,-47.0081806098787,
-0.706541093305005));
#31931=CARTESIAN_POINT('Ctrl Pts',(-48.9072380108242,-48.0226965014984,
-0.647064383360443));
#31932=CARTESIAN_POINT('Ctrl Pts',(-48.1187311062663,-48.6526393867237,
-0.58758767341588));
#31933=CARTESIAN_POINT('Ctrl Pts',(-47.253187942016,-49.3441270008755,-0.522300154147449));
#31934=CARTESIAN_POINT('Ctrl Pts',(-46.0168289438377,-49.5722261083817,
-0.457012634879018));
#31935=CARTESIAN_POINT('Ctrl Pts',(-44.9622730887946,-49.2331401883368,
-0.391725115610587));
#31936=CARTESIAN_POINT('Ctrl Pts',(-43.9077172337516,-48.8940542682919,
-0.326437596342156));
#31937=CARTESIAN_POINT('Ctrl Pts',(-43.0349645218439,-47.9877833206959,
-0.261150077073725));
#31938=CARTESIAN_POINT('Ctrl Pts',(-42.7336951254951,-46.9237470138282,
-0.195862557805293));
#31939=CARTESIAN_POINT('Ctrl Pts',(-42.4324257291462,-45.8597107069604,
-0.130575038536862));
#31940=CARTESIAN_POINT('Ctrl Pts',(-42.7026396483563,-44.6379090408209,
-0.0652875192684313));
#31941=CARTESIAN_POINT('Ctrl Pts',(-43.4267655729853,-43.7934484719077,
0.));
#31942=CARTESIAN_POINT('',(-48.5780058196814,-43.790505499672,-2.89031293644395E-15));
#31943=CARTESIAN_POINT('Origin',(-46.,-46.,0.));
#31944=CARTESIAN_POINT('Ctrl Pts',(-48.5780349767683,-43.7904875157198,
-1.87350135405495E-15));
#31945=CARTESIAN_POINT('Ctrl Pts',(-47.8896982724427,-42.9932829946826,
-0.0620616329205986));
#31946=CARTESIAN_POINT('Ctrl Pts',(-46.7993631439962,-42.5364248278905,
-0.124123265841195));
#31947=CARTESIAN_POINT('Ctrl Pts',(-45.7491449767911,-42.6143557375973,
-0.186184898761792));
#31948=CARTESIAN_POINT('Ctrl Pts',(-44.6443377778701,-42.6963373988856,
-0.251472418030223));
#31949=CARTESIAN_POINT('Ctrl Pts',(-43.5839263871456,-43.3701483645673,
-0.316759937298654));
#31950=CARTESIAN_POINT('Ctrl Pts',(-43.0409891061667,-44.3354564071969,
-0.382047456567084));
#31951=CARTESIAN_POINT('Ctrl Pts',(-42.4980518251879,-45.3007644498266,
-0.447334975835515));
#31952=CARTESIAN_POINT('Ctrl Pts',(-42.4725886539547,-46.5575695694043,
-0.512622495103946));
#31953=CARTESIAN_POINT('Ctrl Pts',(-42.9762878118604,-47.5440868195973,
-0.577910014372377));
#31954=CARTESIAN_POINT('Ctrl Pts',(-43.4799869697661,-48.5306040697903,
-0.643197533640808));
#31955=CARTESIAN_POINT('Ctrl Pts',(-44.5128484568107,-49.2468334505987,
-0.708485052909239));
#31956=CARTESIAN_POINT('Ctrl Pts',(-45.6133080961662,-49.3729753177135,
-0.773772572177669));
#31957=CARTESIAN_POINT('Ctrl Pts',(-46.7137677355217,-49.4991171848283,
-0.8390600914461));
#31958=CARTESIAN_POINT('Ctrl Pts',(-47.8818255271881,-49.0351715382496,
-0.904347610714531));
#31959=CARTESIAN_POINT('Ctrl Pts',(-48.5957489780033,-48.1883179007084,
-0.969635129982962));
#31960=CARTESIAN_POINT('Ctrl Pts',(-49.1036721864121,-47.5858210697928,
-1.01608415223878));
#31961=CARTESIAN_POINT('Ctrl Pts',(-49.3817281116383,-46.7895092998299,
-1.06253317449461));
#31962=CARTESIAN_POINT('Ctrl Pts',(-49.3881103126091,-45.9972329022571,
-1.10898219675043));
#31963=CARTESIAN_POINT('Origin',(-46.,-46.,2.76038497140452));
#31964=CARTESIAN_POINT('',(-50.0803093213768,-45.997675543601,-7.76038497140452));
#31965=CARTESIAN_POINT('',(-50.0862714832512,-46.0033881438983,-7.86461502859548));
#31966=CARTESIAN_POINT('',(-50.085,-45.9999999999999,2.76038497140452));
#31967=CARTESIAN_POINT('',(-49.4256147683784,-48.2253962475631,-9.));
#31968=CARTESIAN_POINT('Ctrl Pts',(-50.0862714832512,-46.0033881438983,
-7.86461502859548));
#31969=CARTESIAN_POINT('Ctrl Pts',(-50.0769067917592,-44.9361782632308,
-7.91663908938817));
#31970=CARTESIAN_POINT('Ctrl Pts',(-49.1080150008643,-42.5144881890784,
-8.03395066944929));
#31971=CARTESIAN_POINT('Ctrl Pts',(-45.0527739768292,-41.2871004410853,
-8.21654976877883));
#31972=CARTESIAN_POINT('Ctrl Pts',(-41.5512814170077,-44.1804051792425,
-8.41241232658412));
#31973=CARTESIAN_POINT('Ctrl Pts',(-42.020443960099,-48.7013832307533,-8.60827488438941));
#31974=CARTESIAN_POINT('Ctrl Pts',(-46.0536368602338,-50.8047688779136,
-8.80413744219471));
#31975=CARTESIAN_POINT('Ctrl Pts',(-48.6953045558515,-49.3495832107922,
-8.93471248073157));
#31976=CARTESIAN_POINT('Ctrl Pts',(-49.4256147683784,-48.2253962475631,
-9.));
#31977=CARTESIAN_POINT('',(-50.0861550027666,-46.2124414226054,-9.));
#31978=CARTESIAN_POINT('Origin',(-46.,-46.,-9.));
#31979=CARTESIAN_POINT('Ctrl Pts',(-50.0803093213768,-45.997675543601,-7.76038497140452));
#31980=CARTESIAN_POINT('Ctrl Pts',(-50.0830253101917,-45.4889855897383,
-7.78509075167359));
#31981=CARTESIAN_POINT('Ctrl Pts',(-49.761077511572,-43.6393405608411,-7.8750840512111));
#31982=CARTESIAN_POINT('Ctrl Pts',(-47.0195848331003,-41.3020769083036,
-8.03036487001704));
#31983=CARTESIAN_POINT('Ctrl Pts',(-42.6509149775089,-42.5514375357737,
-8.22622742782233));
#31984=CARTESIAN_POINT('Ctrl Pts',(-41.2740009567628,-46.8818734807212,
-8.42208998562762));
#31985=CARTESIAN_POINT('Ctrl Pts',(-44.1206550171574,-50.4245588063534,
-8.61795254343291));
#31986=CARTESIAN_POINT('Ctrl Pts',(-48.5697413278868,-50.0204905730501,
-8.81058921489038));
#31987=CARTESIAN_POINT('Ctrl Pts',(-50.0156455888524,-47.4797542540496,
-8.9379383670794));
#31988=CARTESIAN_POINT('Ctrl Pts',(-50.0861960634202,-46.2124371387131,
-9.));
#31989=CARTESIAN_POINT('Origin',(-46.,-46.,2.76038497140452));
#31990=CARTESIAN_POINT('',(-50.0848585401616,-46.0034858730695,-6.51038497140452));
#31991=CARTESIAN_POINT('',(-50.0872042738947,-45.9967790949693,-6.61461502859548));
#31992=CARTESIAN_POINT('',(-50.085,-45.9999999999999,2.76038497140452));
#31993=CARTESIAN_POINT('Ctrl Pts',(-50.0872042738947,-45.9967790949692,
-6.61461502859548));
#31994=CARTESIAN_POINT('Ctrl Pts',(-50.0892699768444,-45.757363874878,-6.62629312117581));
#31995=CARTESIAN_POINT('Ctrl Pts',(-49.9622039222413,-44.1816627080423,
-6.70325873302458));
#31996=CARTESIAN_POINT('Ctrl Pts',(-47.9170393622873,-41.5914781257455,
-6.84551186414177));
#31997=CARTESIAN_POINT('Ctrl Pts',(-43.3883208590233,-41.9640096554919,
-7.04137442194707));
#31998=CARTESIAN_POINT('Ctrl Pts',(-41.1930648262276,-45.9425306703187,
-7.23723697975236));
#31999=CARTESIAN_POINT('Ctrl Pts',(-43.2925649089103,-49.9724248955266,
-7.43309953755766));
#32000=CARTESIAN_POINT('Ctrl Pts',(-47.8111687880873,-50.4530556126673,
-7.62896209536294));
#32001=CARTESIAN_POINT('Ctrl Pts',(-49.9410024707322,-47.8842562868416,
-7.77280059237556));
#32002=CARTESIAN_POINT('Ctrl Pts',(-50.0886589976984,-46.2754717475514,
-7.85135157011974));
#32003=CARTESIAN_POINT('Ctrl Pts',(-50.0862714832512,-46.0033881438983,
-7.86461502859548));
#32004=CARTESIAN_POINT('Ctrl Pts',(-50.0848585401615,-46.0034858730695,
-6.51038497140452));
#32005=CARTESIAN_POINT('Ctrl Pts',(-50.0759395539985,-44.9841466302342,
-6.56003230272967));
#32006=CARTESIAN_POINT('Ctrl Pts',(-49.1785303598923,-42.6103271435563,
-6.67496715332326));
#32007=CARTESIAN_POINT('Ctrl Pts',(-45.2228147324014,-41.2559448461001,
-6.85518952318528));
#32008=CARTESIAN_POINT('Ctrl Pts',(-41.6182000513892,-44.022657337512,-7.05105208099056));
#32009=CARTESIAN_POINT('Ctrl Pts',(-41.9285482915987,-48.5560484764118,
-7.24691463879586));
#32010=CARTESIAN_POINT('Ctrl Pts',(-45.8765970410433,-50.8057107187776,
-7.44277719660115));
#32011=CARTESIAN_POINT('Ctrl Pts',(-49.4229675651535,-49.0194845514499,
-7.61393397413737));
#32012=CARTESIAN_POINT('Ctrl Pts',(-50.075848035475,-46.8332501627557,-7.71980323240516));
#32013=CARTESIAN_POINT('Ctrl Pts',(-50.0803093213768,-45.997675543601,-7.76038497140452));
#32014=CARTESIAN_POINT('Origin',(-46.,-46.,2.76038497140452));
#32015=CARTESIAN_POINT('',(-50.0885301671912,-45.9971742157295,-5.26038497140452));
#32016=CARTESIAN_POINT('',(-50.0791877655715,-46.0012446258329,-5.36461502859548));
#32017=CARTESIAN_POINT('',(-50.085,-45.9999999999999,2.76038497140452));
#32018=CARTESIAN_POINT('Ctrl Pts',(-50.0791877655715,-46.0012446258329,
-5.36461502859548));
#32019=CARTESIAN_POINT('Ctrl Pts',(-50.0770717119439,-45.2467317861072,
-5.40123467223189));
#32020=CARTESIAN_POINT('Ctrl Pts',(-49.5176919519867,-43.1441146815151,
-5.50314183513674));
#32021=CARTESIAN_POINT('Ctrl Pts',(-46.1637649512516,-41.195496195607,-5.67033651731001));
#32022=CARTESIAN_POINT('Ctrl Pts',(-42.0884421952216,-43.2053995648544,
-5.86619907511531));
#32023=CARTESIAN_POINT('Ctrl Pts',(-41.5079465982135,-47.7121709957002,
-6.0620616329206));
#32024=CARTESIAN_POINT('Ctrl Pts',(-44.9409275558383,-50.6891837144081,
-6.25792419072589));
#32025=CARTESIAN_POINT('Ctrl Pts',(-49.0590442379987,-49.5488895831714,
-6.44210865595085));
#32026=CARTESIAN_POINT('Ctrl Pts',(-50.0777214623756,-47.0958380895104,
-6.56100560190738));
#32027=CARTESIAN_POINT('Ctrl Pts',(-50.0872042738947,-45.9967790949692,
-6.61461502859548));
#32028=CARTESIAN_POINT('Ctrl Pts',(-50.0885301671911,-45.9971742157295,
-5.26038497140452));
#32029=CARTESIAN_POINT('Ctrl Pts',(-50.0900435768525,-45.8066458222,-5.26968633451732));
#32030=CARTESIAN_POINT('Ctrl Pts',(-49.9922177014,-44.2803335729962,-5.34427521689855));
#32031=CARTESIAN_POINT('Ctrl Pts',(-48.0737730601331,-41.6630035036824,
-5.48415161854822));
#32032=CARTESIAN_POINT('Ctrl Pts',(-43.5346256929101,-41.8730152769562,
-5.68001417635351));
#32033=CARTESIAN_POINT('Ctrl Pts',(-41.1981957029014,-45.7703295255252,
-5.87587673415881));
#32034=CARTESIAN_POINT('Ctrl Pts',(-43.1519934739611,-49.8728455133488,
-6.0717392919641));
#32035=CARTESIAN_POINT('Ctrl Pts',(-47.6503759783394,-50.5151226960096,
-6.26760184976939));
#32036=CARTESIAN_POINT('Ctrl Pts',(-49.9077275125445,-47.9830689624062,
-6.41381707624954));
#32037=CARTESIAN_POINT('Ctrl Pts',(-50.087668250495,-46.3246039857731,-6.49474478346124));
#32038=CARTESIAN_POINT('Ctrl Pts',(-50.0848585401615,-46.0034858730695,
-6.51038497140452));
#32039=CARTESIAN_POINT('Origin',(-46.,-46.,2.76038497140452));
#32040=CARTESIAN_POINT('',(-50.0788652030139,-46.0005097590054,-4.01038497140452));
#32041=CARTESIAN_POINT('',(-50.0908854225478,-46.0013070164178,-4.11461502859548));
#32042=CARTESIAN_POINT('',(-50.085,-45.9999999999999,2.76038497140452));
#32043=CARTESIAN_POINT('Ctrl Pts',(-50.0908854225478,-46.0013070164178,
-4.11461502859548));
#32044=CARTESIAN_POINT('Ctrl Pts',(-50.0855211619739,-44.7422069936917,
-4.17617622328797));
#32045=CARTESIAN_POINT('Ctrl Pts',(-48.7949531014785,-42.1382705071838,
-4.3030249372489));
#32046=CARTESIAN_POINT('Ctrl Pts',(-44.3875999794073,-41.4711765661473,
-4.49516117047825));
#32047=CARTESIAN_POINT('Ctrl Pts',(-41.3353873965154,-44.8374748217385,
-4.69102372828354));
#32048=CARTESIAN_POINT('Ctrl Pts',(-42.4508271650107,-49.2424447068201,
-4.88688628608884));
#32049=CARTESIAN_POINT('Ctrl Pts',(-46.7373166435254,-50.7504146876272,
-5.08274884389413));
#32050=CARTESIAN_POINT('Ctrl Pts',(-49.6867806300422,-48.5256746587921,
-5.24199175806301));
#32051=CARTESIAN_POINT('Ctrl Pts',(-50.080844328995,-46.5919188679631,-5.33594715296346));
#32052=CARTESIAN_POINT('Ctrl Pts',(-50.0791877655715,-46.0012446258329,
-5.36461502859548));
#32053=CARTESIAN_POINT('Ctrl Pts',(-50.0788652030139,-46.0005097590054,
-4.01038497140452));
#32054=CARTESIAN_POINT('Ctrl Pts',(-50.0780586190038,-45.2948273556406,
-4.0446278855734));
#32055=CARTESIAN_POINT('Ctrl Pts',(-49.5711124212075,-43.2426058741684,
-4.14415831901071));
#32056=CARTESIAN_POINT('Ctrl Pts',(-46.3358174043579,-41.204449981662,-4.30897627171646));
#32057=CARTESIAN_POINT('Ctrl Pts',(-42.1910921533903,-43.0670331890375,
-4.50483882952175));
#32058=CARTESIAN_POINT('Ctrl Pts',(-41.4494798905217,-47.5501096808741,
-4.70070138732705));
#32059=CARTESIAN_POINT('Ctrl Pts',(-44.7735827067234,-50.6482226625802,
-4.89656394513233));
#32060=CARTESIAN_POINT('Ctrl Pts',(-48.9835465579835,-49.6434232658214,
-5.08312513982483));
#32061=CARTESIAN_POINT('Ctrl Pts',(-50.0794207507967,-47.1439902536432,
-5.20439881524889));
#32062=CARTESIAN_POINT('Ctrl Pts',(-50.0885301671911,-45.9971742157295,
-5.26038497140452));
#32063=CARTESIAN_POINT('Origin',(-46.,-46.,2.76038497140452));
#32064=CARTESIAN_POINT('',(-50.0900545172792,-46.0020418321801,-2.76038497140452));
#32065=CARTESIAN_POINT('',(-50.081795401254,-45.9969676253998,-2.86461502859548));
#32066=CARTESIAN_POINT('',(-50.085,-45.9999999999999,2.76038497140452));
#32067=CARTESIAN_POINT('Ctrl Pts',(-50.081795401254,-45.9969676253998,-2.86461502859548));
#32068=CARTESIAN_POINT('Ctrl Pts',(-50.0849112009229,-45.560551617548,-2.88583025507562));
#32069=CARTESIAN_POINT('Ctrl Pts',(-49.8212806234326,-43.7847766277542,
-2.97233300082419));
#32070=CARTESIAN_POINT('Ctrl Pts',(-47.2654095909828,-41.362240430431,-3.1241232658412));
#32071=CARTESIAN_POINT('Ctrl Pts',(-42.8368466927335,-42.379981111081,-3.31998582364649));
#32072=CARTESIAN_POINT('Ctrl Pts',(-41.2344398737399,-46.6320697906436,
-3.51584838145178));
#32073=CARTESIAN_POINT('Ctrl Pts',(-43.8898781422471,-50.3194283458399,
-3.71171093925708));
#32074=CARTESIAN_POINT('Ctrl Pts',(-48.4306293080085,-50.1475434533866,
-3.90757349706237));
#32075=CARTESIAN_POINT('Ctrl Pts',(-50.0550862518107,-47.4887349722982,
-4.04187486017517));
#32076=CARTESIAN_POINT('Ctrl Pts',(-50.091210123459,-46.0775208615468,-4.11088870401954));
#32077=CARTESIAN_POINT('Ctrl Pts',(-50.0908854225478,-46.0013070164178,
-4.11461502859548));
#32078=CARTESIAN_POINT('Ctrl Pts',(-50.0900545172792,-46.0020418321801,
-2.76038497140452));
#32079=CARTESIAN_POINT('Ctrl Pts',(-50.0825375788689,-44.7908992747219,
-2.81956943662948));
#32080=CARTESIAN_POINT('Ctrl Pts',(-48.8773452250357,-42.2307009333171,
-2.94404142112287));
#32081=CARTESIAN_POINT('Ctrl Pts',(-44.5509149516467,-41.4163086543115,
-3.1338009248847));
#32082=CARTESIAN_POINT('Ctrl Pts',(-41.3800394184348,-44.6710764629181,
-3.32966348268999));
#32083=CARTESIAN_POINT('Ctrl Pts',(-42.3369215031958,-49.1131863035692,
-3.52552604049529));
#32084=CARTESIAN_POINT('Ctrl Pts',(-46.5666235775808,-50.7737837298756,
-3.72138859830058));
#32085=CARTESIAN_POINT('Ctrl Pts',(-49.6390942515875,-48.6245534357952,
-3.88300824193699));
#32086=CARTESIAN_POINT('Ctrl Pts',(-50.0795964515855,-46.6402809954754,
-3.97934036630497));
#32087=CARTESIAN_POINT('Ctrl Pts',(-50.0788652030139,-46.0005097590054,
-4.01038497140452));
#32088=CARTESIAN_POINT('Origin',(-46.,-46.,2.76038497140452));
#32089=CARTESIAN_POINT('',(-50.0830240067876,-45.9966653604899,-1.51038497140452));
#32090=CARTESIAN_POINT('',(-50.0828677018166,-46.0033110698502,-1.61461502859548));
#32091=CARTESIAN_POINT('',(-50.085,-45.9999999999999,2.76038497140452));
#32092=CARTESIAN_POINT('Ctrl Pts',(-50.0828677018166,-46.0033110698502,
-1.61461502859548));
#32093=CARTESIAN_POINT('Ctrl Pts',(-50.0753230858173,-45.0544576856415,
-1.6607718061317));
#32094=CARTESIAN_POINT('Ctrl Pts',(-49.2773378217668,-42.7520207060235,
-1.77221610293635));
#32095=CARTESIAN_POINT('Ctrl Pts',(-45.4734860003987,-41.2216278875877,
-1.94894791900943));
#32096=CARTESIAN_POINT('Ctrl Pts',(-41.7282986823175,-43.794859117017,-2.14481047681473));
#32097=CARTESIAN_POINT('Ctrl Pts',(-41.7997119996332,-48.3383026030494,
-2.34067303462002));
#32098=CARTESIAN_POINT('Ctrl Pts',(-45.6239217216425,-50.7925607363461,
-2.53653559242531));
#32099=CARTESIAN_POINT('Ctrl Pts',(-49.3335205372955,-49.1628225231174,
-2.71118292375047));
#32100=CARTESIAN_POINT('Ctrl Pts',(-50.0753226711417,-46.9035737412263,
-2.82054273580719));
#32101=CARTESIAN_POINT('Ctrl Pts',(-50.081795401254,-45.9969676253998,-2.86461502859548));
#32102=CARTESIAN_POINT('Ctrl Pts',(-50.0830240067876,-45.9966653604899,
-1.51038497140452));
#32103=CARTESIAN_POINT('Ctrl Pts',(-50.0861433599091,-45.6094337666882,
-1.52922346841713));
#32104=CARTESIAN_POINT('Ctrl Pts',(-49.8595841509064,-43.8837675877116,
-1.61334948469817));
#32105=CARTESIAN_POINT('Ctrl Pts',(-47.4307680051951,-41.41057421285,-1.76276302024764));
#32106=CARTESIAN_POINT('Ctrl Pts',(-42.9685984702712,-42.2689561020525,
-1.95862557805293));
#32107=CARTESIAN_POINT('Ctrl Pts',(-41.2148490309835,-46.4609045794214,
-2.15448813585823));
#32108=CARTESIAN_POINT('Ctrl Pts',(-43.7364585340961,-50.2410417148001,
-2.35035069366352));
#32109=CARTESIAN_POINT('Ctrl Pts',(-48.2804504821097,-50.2319761154881,
-2.54621325146882));
#32110=CARTESIAN_POINT('Ctrl Pts',(-50.0295523051546,-47.5870903820588,
-2.68289134404915));
#32111=CARTESIAN_POINT('Ctrl Pts',(-50.0908296578703,-46.1269338702245,
-2.75428191736105));
#32112=CARTESIAN_POINT('Ctrl Pts',(-50.0900545172792,-46.0020418321801,
-2.76038497140452));
#32113=CARTESIAN_POINT('Origin',(-46.,-46.,2.76038497140452));
#32114=CARTESIAN_POINT('',(-50.0805802565567,-46.0038346370175,-0.260384971404518));
#32115=CARTESIAN_POINT('',(-50.0901578141997,-45.9981376217778,-0.364615028595479));
#32116=CARTESIAN_POINT('',(-50.085,-45.9999999999999,2.76038497140452));
#32117=CARTESIAN_POINT('',(-47.057904422973,-49.9456385074984,0.));
#32118=CARTESIAN_POINT('Ctrl Pts',(-47.0579044229729,-49.9456385074984,
5.55111512312578E-16));
#32119=CARTESIAN_POINT('Ctrl Pts',(-48.3527480267224,-49.5984650974504,
-0.0652875192684306));
#32120=CARTESIAN_POINT('Ctrl Pts',(-49.8153067462896,-48.2273633419822,
-0.152082509736604));
#32121=CARTESIAN_POINT('Ctrl Pts',(-50.0835490595066,-46.4463082039673,
-0.238877500204776));
#32122=CARTESIAN_POINT('Ctrl Pts',(-50.0805802565567,-46.0038346370175,
-0.260384971404518));
#32123=CARTESIAN_POINT('',(-44.9393523503947,-49.9518124380696,-3.33880900068018E-15));
#32124=CARTESIAN_POINT('Origin',(-46.,-46.,0.));
#32125=CARTESIAN_POINT('Ctrl Pts',(-44.9393355849193,-49.9518501705994,
6.45100292628875E-17));
#32126=CARTESIAN_POINT('Ctrl Pts',(-46.166426942727,-50.2763750719212,-0.0620616329205977));
#32127=CARTESIAN_POINT('Ctrl Pts',(-48.8989758948986,-49.7132910486246,
-0.183599975785757));
#32128=CARTESIAN_POINT('Ctrl Pts',(-50.0828902798758,-47.2149621037996,
-0.305138318650917));
#32129=CARTESIAN_POINT('Ctrl Pts',(-50.0901578141997,-45.9981376217778,
-0.364615028595479));
#32130=CARTESIAN_POINT('Origin',(46.,-46.,-5.));
#32131=CARTESIAN_POINT('',(42.6091952652934,-46.0028114996479,-8.26601780324956));
#32132=CARTESIAN_POINT('',(42.6044125646165,-46.0001574521336,-8.60898219675043));
#32133=CARTESIAN_POINT('',(42.61025,-46.,-5.));
#32134=CARTESIAN_POINT('',(47.303382040875,-42.8708467090881,-9.));
#32135=CARTESIAN_POINT('Ctrl Pts',(42.6044125646165,-46.0001574521336,-8.60898219675043));
#32136=CARTESIAN_POINT('Ctrl Pts',(42.6053219601772,-44.8964212032941,-8.67403394523185));
#32137=CARTESIAN_POINT('Ctrl Pts',(43.1965789016692,-43.7921183414524,-8.73908569371328));
#32138=CARTESIAN_POINT('Ctrl Pts',(44.1121218294326,-43.1790110276343,-8.80413744219471));
#32139=CARTESIAN_POINT('Ctrl Pts',(45.0309830119955,-42.5636815937768,-8.86942496146314));
#32140=CARTESIAN_POINT('Ctrl Pts',(46.2764850972779,-42.4431146967252,-8.93471248073157));
#32141=CARTESIAN_POINT('Ctrl Pts',(47.3033820408749,-42.8708467090881,-9.));
#32142=CARTESIAN_POINT('',(42.61025,-46.,-9.));
#32143=CARTESIAN_POINT('Origin',(46.,-46.,-9.));
#32144=CARTESIAN_POINT('',(42.61025,-46.,-10.));
#32145=CARTESIAN_POINT('',(42.61025,-46.,-5.));
#32146=CARTESIAN_POINT('Origin',(46.,-46.,-10.));
#32147=CARTESIAN_POINT('',(48.8980017072691,-47.7690577679613,-9.));
#32148=CARTESIAN_POINT('Origin',(46.,-46.,-9.));
#32149=CARTESIAN_POINT('Ctrl Pts',(48.8980278172144,-47.7690799369094,-9.));
#32150=CARTESIAN_POINT('Ctrl Pts',(49.4435067823307,-46.8680830001505,-8.9379383670794));
#32151=CARTESIAN_POINT('Ctrl Pts',(49.5410722981907,-45.6899359369109,-8.8758767341588));
#32152=CARTESIAN_POINT('Ctrl Pts',(49.1424202878046,-44.7152011753849,-8.81381510123821));
#32153=CARTESIAN_POINT('Ctrl Pts',(48.7230468426555,-43.689800915515,-8.74852758196978));
#32154=CARTESIAN_POINT('Ctrl Pts',(47.7545296578687,-42.8895087708225,-8.68324006270134));
#32155=CARTESIAN_POINT('Ctrl Pts',(46.6686904094295,-42.6714413128456,-8.61795254343291));
#32156=CARTESIAN_POINT('Ctrl Pts',(45.5828511609903,-42.4533738548687,-8.55266502416448));
#32157=CARTESIAN_POINT('Ctrl Pts',(44.3796898488986,-42.8175310836074,-8.48737750489605));
#32158=CARTESIAN_POINT('Ctrl Pts',(43.5971078026617,-43.6014280129255,-8.42208998562762));
#32159=CARTESIAN_POINT('Ctrl Pts',(42.973510882379,-44.2260726917709,-8.37006592483494));
#32160=CARTESIAN_POINT('Ctrl Pts',(42.6169660769066,-45.1172363928553,-8.31804186404225));
#32161=CARTESIAN_POINT('Ctrl Pts',(42.6091952652934,-46.0028114996479,-8.26601780324956));
#32162=CARTESIAN_POINT('Origin',(46.,-46.,-5.));
#32163=CARTESIAN_POINT('',(42.6084212224847,-45.9973272800439,-7.01601780324956));
#32164=CARTESIAN_POINT('',(42.6141425307955,-45.9980711599138,-7.35898219675043));
#32165=CARTESIAN_POINT('',(42.61025,-46.,-5.));
#32166=CARTESIAN_POINT('Ctrl Pts',(42.6141425307955,-45.9980711599138,-7.35898219675043));
#32167=CARTESIAN_POINT('Ctrl Pts',(42.6118887907293,-45.575958143871,-7.3836879770195));
#32168=CARTESIAN_POINT('Ctrl Pts',(42.6852302319893,-45.154599048709,-7.40839375728858));
#32169=CARTESIAN_POINT('Ctrl Pts',(42.8378019484186,-44.7642018229609,-7.43309953755765));
#32170=CARTESIAN_POINT('Ctrl Pts',(43.2409881165019,-43.7325377297497,-7.49838705682608));
#32171=CARTESIAN_POINT('Ctrl Pts',(44.197466231587,-42.9170908965982,-7.56367457609451));
#32172=CARTESIAN_POINT('Ctrl Pts',(45.2798953093061,-42.6821549238822,-7.62896209536294));
#32173=CARTESIAN_POINT('Ctrl Pts',(46.3623243870251,-42.4472189511661,-7.69424961463137));
#32174=CARTESIAN_POINT('Ctrl Pts',(47.570704427378,-42.7927938388857,-7.7595371338998));
#32175=CARTESIAN_POINT('Ctrl Pts',(48.3653226299911,-43.5644835193059,-7.82482465316823));
#32176=CARTESIAN_POINT('Ctrl Pts',(49.1599408326043,-44.3361731997261,-7.89011217243666));
#32177=CARTESIAN_POINT('Ctrl Pts',(49.5407971974777,-45.5339776728469,-7.95539969170509));
#32178=CARTESIAN_POINT('Ctrl Pts',(49.3375311222527,-46.6228357674574,-8.02068721097353));
#32179=CARTESIAN_POINT('Ctrl Pts',(49.1342650470278,-47.7116938620679,-8.08597473024196));
#32180=CARTESIAN_POINT('Ctrl Pts',(48.3468765317045,-48.6916055781681,-8.15126224951039));
#32181=CARTESIAN_POINT('Ctrl Pts',(47.3275666791222,-49.1247426138568,-8.21654976877882));
#32182=CARTESIAN_POINT('Ctrl Pts',(46.3082568265399,-49.5578796495455,-8.28183728804725));
#32183=CARTESIAN_POINT('Ctrl Pts',(45.0570256366986,-49.4442420048227,-8.34712480731568));
#32184=CARTESIAN_POINT('Ctrl Pts',(44.1319143151655,-48.8347431895811,-8.41241232658411));
#32185=CARTESIAN_POINT('Ctrl Pts',(43.2068029936325,-48.2252443743394,-8.47769984585254));
#32186=CARTESIAN_POINT('Ctrl Pts',(42.6078115404076,-47.119884388579,-8.54298736512097));
#32187=CARTESIAN_POINT('Ctrl Pts',(42.604425953717,-46.0121584103671,-8.60827488438941));
#32188=CARTESIAN_POINT('Ctrl Pts',(42.6044137274531,-46.0081581140073,-8.60851065517642));
#32189=CARTESIAN_POINT('Ctrl Pts',(42.6044092686419,-46.004157786792,-8.60874642596342));
#32190=CARTESIAN_POINT('Ctrl Pts',(42.6044125646165,-46.0001574521336,-8.60898219675043));
#32191=CARTESIAN_POINT('Ctrl Pts',(42.6091952652934,-46.0028114996479,-8.26601780324956));
#32192=CARTESIAN_POINT('Ctrl Pts',(42.6072141081983,-46.2285875824282,-8.25275434477382));
#32193=CARTESIAN_POINT('Ctrl Pts',(42.6279028279941,-46.4540004135131,-8.23949088629807));
#32194=CARTESIAN_POINT('Ctrl Pts',(42.6726156656388,-46.6745408053554,-8.22622742782233));
#32195=CARTESIAN_POINT('Ctrl Pts',(42.8927083552351,-47.7601200385699,-8.16093990855389));
#32196=CARTESIAN_POINT('Ctrl Pts',(43.6948965148099,-48.7276418751015,-8.09565238928547));
#32197=CARTESIAN_POINT('Ctrl Pts',(44.7209166029033,-49.1449312387884,-8.03036487001703));
#32198=CARTESIAN_POINT('Ctrl Pts',(45.7469366909968,-49.5622206024753,-7.9650773507486));
#32199=CARTESIAN_POINT('Ctrl Pts',(46.9967887076088,-49.4292774933176,-7.89978983148017));
#32200=CARTESIAN_POINT('Ctrl Pts',(47.9120769940113,-48.8054688270359,-7.83450231221174));
#32201=CARTESIAN_POINT('Ctrl Pts',(48.8273652804138,-48.1816601607542,-7.76921479294331));
#32202=CARTESIAN_POINT('Ctrl Pts',(49.4080898366068,-47.0669859373486,-7.70392727367488));
#32203=CARTESIAN_POINT('Ctrl Pts',(49.3948467186262,-45.959416665038,-7.63863975440645));
#32204=CARTESIAN_POINT('Ctrl Pts',(49.3816036006456,-44.8518473927274,-7.57335223513801));
#32205=CARTESIAN_POINT('Ctrl Pts',(48.7743928084915,-43.7513830715118,-7.50806471586958));
#32206=CARTESIAN_POINT('Ctrl Pts',(47.8444625615455,-43.1496295467018,-7.44277719660115));
#32207=CARTESIAN_POINT('Ctrl Pts',(46.9145323145995,-42.5478760218918,-7.37748967733272));
#32208=CARTESIAN_POINT('Ctrl Pts',(45.6618826128616,-42.4448332934873,-7.31220215806429));
#32209=CARTESIAN_POINT('Ctrl Pts',(44.6461163251007,-42.8865364012444,-7.24691463879586));
#32210=CARTESIAN_POINT('Ctrl Pts',(43.6303500373398,-43.3282395090014,-7.18162711952743));
#32211=CARTESIAN_POINT('Ctrl Pts',(42.8514671635558,-44.3146884529201,-7.116339600259));
#32212=CARTESIAN_POINT('Ctrl Pts',(42.6574159170588,-45.405204785632,-7.05105208099057));
#32213=CARTESIAN_POINT('Ctrl Pts',(42.6227056317345,-45.600267346386,-7.03937398841023));
#32214=CARTESIAN_POINT('Ctrl Pts',(42.6067070937495,-45.7986595538186,-7.0276958958299));
#32215=CARTESIAN_POINT('Ctrl Pts',(42.6084212224847,-45.9973272800439,-7.01601780324956));
#32216=CARTESIAN_POINT('Origin',(46.,-46.,-5.));
#32217=CARTESIAN_POINT('',(42.6150733527443,-46.0010327955954,-5.76601780324956));
#32218=CARTESIAN_POINT('',(42.610367575631,-46.0028925918188,-6.10898219675042));
#32219=CARTESIAN_POINT('',(42.61025,-46.,-5.));
#32220=CARTESIAN_POINT('Ctrl Pts',(42.610367575631,-46.0028925918188,-6.10898219675042));
#32221=CARTESIAN_POINT('Ctrl Pts',(42.6177685869596,-45.1570406939323,-6.15862952807558));
#32222=CARTESIAN_POINT('Ctrl Pts',(42.9394383742148,-44.3061623939123,-6.20827685940073));
#32223=CARTESIAN_POINT('Ctrl Pts',(43.5127592901994,-43.6890940545951,-6.25792419072588));
#32224=CARTESIAN_POINT('Ctrl Pts',(44.2666910595466,-42.877633296931,-6.32321170999432));
#32225=CARTESIAN_POINT('Ctrl Pts',(45.4558012966754,-42.4704984048589,-6.38849922926275));
#32226=CARTESIAN_POINT('Ctrl Pts',(46.5488770971372,-42.6495691939267,-6.45378674853118));
#32227=CARTESIAN_POINT('Ctrl Pts',(47.641952897599,-42.8286399829945,-6.51907426779961));
#32228=CARTESIAN_POINT('Ctrl Pts',(48.6389942613939,-43.5939164532021,-6.58436178706804));
#32229=CARTESIAN_POINT('Ctrl Pts',(49.0945935696661,-44.6035257912972,-6.64964930633647));
#32230=CARTESIAN_POINT('Ctrl Pts',(49.5501928779384,-45.6131351293924,-6.7149368256049));
#32231=CARTESIAN_POINT('Ctrl Pts',(49.4643501306881,-46.8670773353749,-6.78022434487333));
#32232=CARTESIAN_POINT('Ctrl Pts',(48.8754109060044,-47.8051782700423,-6.84551186414176));
#32233=CARTESIAN_POINT('Ctrl Pts',(48.2864716813207,-48.7432792047097,-6.91079938341019));
#32234=CARTESIAN_POINT('Ctrl Pts',(47.1944359792037,-49.3655388680619,-6.97608690267863));
#32235=CARTESIAN_POINT('Ctrl Pts',(46.0871559716595,-49.3939737149546,-7.04137442194706));
#32236=CARTESIAN_POINT('Ctrl Pts',(44.9798759641153,-49.4224085618473,-7.10666194121549));
#32237=CARTESIAN_POINT('Ctrl Pts',(43.8573516511439,-48.8570185922806,-7.17194946048392));
#32238=CARTESIAN_POINT('Ctrl Pts',(43.221036605199,-47.9503829308618,-7.23723697975235));
#32239=CARTESIAN_POINT('Ctrl Pts',(42.8255127530867,-47.3868318541555,-7.27781871875171));
#32240=CARTESIAN_POINT('Ctrl Pts',(42.6178445264477,-46.6914344157477,-7.31840045775107));
#32241=CARTESIAN_POINT('Ctrl Pts',(42.6141425307955,-45.9980711599138,-7.35898219675043));
#32242=CARTESIAN_POINT('Ctrl Pts',(42.6084212224847,-45.9973272800439,-7.01601780324956));
#32243=CARTESIAN_POINT('Ctrl Pts',(42.6162900981709,-46.9093309168622,-6.96240837656147));
#32244=CARTESIAN_POINT('Ctrl Pts',(42.9974284256452,-47.8271407233737,-6.90879894987337));
#32245=CARTESIAN_POINT('Ctrl Pts',(43.6551847755762,-48.4552992360462,-6.85518952318527));
#32246=CARTESIAN_POINT('Ctrl Pts',(44.4562244998004,-49.2202936322432,-6.78990200391684));
#32247=CARTESIAN_POINT('Ctrl Pts',(45.6675235674587,-49.5556987031322,-6.72461448464841));
#32248=CARTESIAN_POINT('Ctrl Pts',(46.7479567014102,-49.3116783556131,-6.65932696537998));
#32249=CARTESIAN_POINT('Ctrl Pts',(47.8283898353616,-49.067658008094,-6.59403944611154));
#32250=CARTESIAN_POINT('Ctrl Pts',(48.7779570356062,-48.2442122421669,-6.52875192684312));
#32251=CARTESIAN_POINT('Ctrl Pts',(49.1724577001302,-47.2091998064185,-6.46346440757469));
#32252=CARTESIAN_POINT('Ctrl Pts',(49.5669583646541,-46.1741873706701,-6.39817688830625));
#32253=CARTESIAN_POINT('Ctrl Pts',(49.4063924934574,-44.9276082651004,-6.33288936903782));
#32254=CARTESIAN_POINT('Ctrl Pts',(48.7624896500348,-44.0263477099034,-6.26760184976939));
#32255=CARTESIAN_POINT('Ctrl Pts',(48.1185868066121,-43.1250871547063,-6.20231433050096));
#32256=CARTESIAN_POINT('Ctrl Pts',(46.9913469909636,-42.5691451498819,-6.13702681123253));
#32257=CARTESIAN_POINT('Ctrl Pts',(45.8843430380562,-42.6068781550557,-6.0717392919641));
#32258=CARTESIAN_POINT('Ctrl Pts',(44.7773390851488,-42.6446111602295,-6.00645177269567));
#32259=CARTESIAN_POINT('Ctrl Pts',(43.6905709949825,-43.2760191754015,-5.94116425342724));
#32260=CARTESIAN_POINT('Ctrl Pts',(43.1095315203292,-44.2190327676712,-5.8758767341588));
#32261=CARTESIAN_POINT('Ctrl Pts',(42.7836275996577,-44.7479672727674,-5.83925709052239));
#32262=CARTESIAN_POINT('Ctrl Pts',(42.6168292626847,-45.3749349634637,-5.80263744688598));
#32263=CARTESIAN_POINT('Ctrl Pts',(42.6150733527443,-46.0010327955954,-5.76601780324956));
#32264=CARTESIAN_POINT('Origin',(46.,-46.,-5.));
#32265=CARTESIAN_POINT('',(42.6053665892596,-46.0010845675542,-4.51601780324957));
#32266=CARTESIAN_POINT('',(42.6073208444166,-45.9976551525847,-4.85898219675043));
#32267=CARTESIAN_POINT('',(42.61025,-46.,-5.));
#32268=CARTESIAN_POINT('Ctrl Pts',(42.6073208444166,-45.9976551525847,-4.85898219675043));
#32269=CARTESIAN_POINT('Ctrl Pts',(42.6060650108524,-45.8395539076774,-4.86828355986323));
#32270=CARTESIAN_POINT('Ctrl Pts',(42.6161878381193,-45.6816141480506,-4.87758492297603));
#32271=CARTESIAN_POINT('Ctrl Pts',(42.6382491084881,-45.5253599574508,-4.88688628608883));
#32272=CARTESIAN_POINT('Ctrl Pts',(42.7931001337434,-44.4285907682639,-4.95217380535726));
#32273=CARTESIAN_POINT('Ctrl Pts',(43.5361373577979,-43.4148666152112,-5.01746132462569));
#32274=CARTESIAN_POINT('Ctrl Pts',(44.5354231635466,-42.9370493109476,-5.08274884389412));
#32275=CARTESIAN_POINT('Ctrl Pts',(45.5347089692953,-42.459232006684,-5.14803636316255));
#32276=CARTESIAN_POINT('Ctrl Pts',(46.7902433567382,-42.5173215512096,-5.21332388243098));
#32277=CARTESIAN_POINT('Ctrl Pts',(47.7411404203322,-43.0853675567301,-5.27861140169942));
#32278=CARTESIAN_POINT('Ctrl Pts',(48.6920374839263,-43.6534135622506,-5.34389892096785));
#32279=CARTESIAN_POINT('Ctrl Pts',(49.3382972236715,-44.7314160287659,-5.40918644023628));
#32280=CARTESIAN_POINT('Ctrl Pts',(49.3912155219598,-45.8377980365326,-5.47447395950471));
#32281=CARTESIAN_POINT('Ctrl Pts',(49.444133820248,-46.9441800442992,-5.53976147877314));
#32282=CARTESIAN_POINT('Ctrl Pts',(48.9037106770792,-48.0789415933172,-5.60504899804157));
#32283=CARTESIAN_POINT('Ctrl Pts',(48.0113697202318,-48.735149742658,-5.67033651731));
#32284=CARTESIAN_POINT('Ctrl Pts',(47.1190287633844,-49.3913578919989,-5.73562403657843));
#32285=CARTESIAN_POINT('Ctrl Pts',(45.8747699928583,-49.5690126416627,-5.80091155584687));
#32286=CARTESIAN_POINT('Ctrl Pts',(44.8344422234934,-49.1887501277354,-5.8661990751153));
#32287=CARTESIAN_POINT('Ctrl Pts',(43.7941144541285,-48.8084876138081,-5.93148659438373));
#32288=CARTESIAN_POINT('Ctrl Pts',(42.9577176859246,-47.8703078362897,-5.99677411365216));
#32289=CARTESIAN_POINT('Ctrl Pts',(42.6988959526055,-46.7933246359025,-6.06206163292059));
#32290=CARTESIAN_POINT('Ctrl Pts',(42.6368929756464,-46.5353240279064,-6.07770182086387));
#32291=CARTESIAN_POINT('Ctrl Pts',(42.608036066463,-46.2693577230156,-6.09334200880715));
#32292=CARTESIAN_POINT('Ctrl Pts',(42.610367575631,-46.0028925918188,-6.10898219675042));
#32293=CARTESIAN_POINT('Ctrl Pts',(42.6150733527443,-46.0010327955954,-5.76601780324956));
#32294=CARTESIAN_POINT('Ctrl Pts',(42.6136987296515,-46.4911766911296,-5.73734992761755));
#32295=CARTESIAN_POINT('Ctrl Pts',(42.7134723622383,-46.980787483279,-5.70868205198553));
#32296=CARTESIAN_POINT('Ctrl Pts',(42.9172426426718,-47.4224132450777,-5.68001417635351));
#32297=CARTESIAN_POINT('Ctrl Pts',(43.3813040988082,-48.4281609608471,-5.61472665708508));
#32298=CARTESIAN_POINT('Ctrl Pts',(44.3847378702214,-49.1850372230187,-5.54943913781665));
#32299=CARTESIAN_POINT('Ctrl Pts',(45.4792791649687,-49.3549220805656,-5.48415161854822));
#32300=CARTESIAN_POINT('Ctrl Pts',(46.573820459716,-49.5248069381124,-5.41886409927979));
#32301=CARTESIAN_POINT('Ctrl Pts',(47.7594692777973,-49.1077003910346,-5.35357658001136));
#32302=CARTESIAN_POINT('Ctrl Pts',(48.5065597651538,-48.2899367876744,-5.28828906074293));
#32303=CARTESIAN_POINT('Ctrl Pts',(49.2536502525103,-47.4721731843143,-5.22300154147449));
#32304=CARTESIAN_POINT('Ctrl Pts',(49.562182409142,-46.2537525246719,-5.15771402220606));
#32305=CARTESIAN_POINT('Ctrl Pts',(49.2943254121986,-45.178980857527,-5.09242650293763));
#32306=CARTESIAN_POINT('Ctrl Pts',(49.0264684152553,-44.104209190382,-5.0271389836692));
#32307=CARTESIAN_POINT('Ctrl Pts',(48.1822222647368,-43.1730865157345,-4.96185146440077));
#32308=CARTESIAN_POINT('Ctrl Pts',(47.1387377295478,-42.8015740221576,-4.89656394513234));
#32309=CARTESIAN_POINT('Ctrl Pts',(46.0952531943588,-42.4300615285808,-4.83127642586391));
#32310=CARTESIAN_POINT('Ctrl Pts',(44.8525302744992,-42.6181592160746,-4.76598890659548));
#32311=CARTESIAN_POINT('Ctrl Pts',(43.965731587706,-43.2818380515628,-4.70070138732704));
#32312=CARTESIAN_POINT('Ctrl Pts',(43.1295474713166,-43.9076370168566,-4.63914019263455));
#32313=CARTESIAN_POINT('Ctrl Pts',(42.6098178745654,-44.9562782327072,-4.57757899794206));
#32314=CARTESIAN_POINT('Ctrl Pts',(42.6053665892596,-46.0010845675542,-4.51601780324957));
#32315=CARTESIAN_POINT('Origin',(46.,-46.,-5.));
#32316=CARTESIAN_POINT('',(42.6129095260066,-45.9974837232043,-3.26601780324956));
#32317=CARTESIAN_POINT('',(42.6153408714561,-46.0004230001184,-3.60898219675043));
#32318=CARTESIAN_POINT('',(42.61025,-46.,-5.));
#32319=CARTESIAN_POINT('Ctrl Pts',(42.6153408714561,-46.0004230001184,-3.60898219675043));
#32320=CARTESIAN_POINT('Ctrl Pts',(42.6160101781871,-45.4148448381747,-3.64322511091931));
#32321=CARTESIAN_POINT('Ctrl Pts',(42.7607380833382,-44.828956794812,-3.67746802508819));
#32322=CARTESIAN_POINT('Ctrl Pts',(43.047571146859,-44.3237493941201,-3.71171093925707));
#32323=CARTESIAN_POINT('Ctrl Pts',(43.5944468908181,-43.3605212721047,-3.7769984585255));
#32324=CARTESIAN_POINT('Ctrl Pts',(44.6578921134554,-42.6905770674502,-3.84228597779393));
#32325=CARTESIAN_POINT('Ctrl Pts',(45.7628330693288,-42.6132015000149,-3.90757349706236));
#32326=CARTESIAN_POINT('Ctrl Pts',(46.8677740252022,-42.5358259325796,-3.97286101633079));
#32327=CARTESIAN_POINT('Ctrl Pts',(48.0142107143115,-43.0510190023635,-4.03814853559923));
#32328=CARTESIAN_POINT('Ctrl Pts',(48.6899945433991,-43.9286280904542,-4.10343605486766));
#32329=CARTESIAN_POINT('Ctrl Pts',(49.3657783724867,-44.8062371785449,-4.16872357413609));
#32330=CARTESIAN_POINT('Ctrl Pts',(49.5709093415525,-46.0462622849423,-4.23401109340452));
#32331=CARTESIAN_POINT('Ctrl Pts',(49.2137491270214,-47.0947459881169,-4.29929861267295));
#32332=CARTESIAN_POINT('Ctrl Pts',(48.8565889124903,-48.1432296912914,-4.36458613194138));
#32333=CARTESIAN_POINT('Ctrl Pts',(47.9371375143622,-49.000171991243,-4.42987365120981));
#32334=CARTESIAN_POINT('Ctrl Pts',(46.8661422009793,-49.2827503588996,-4.49516117047824));
#32335=CARTESIAN_POINT('Ctrl Pts',(45.7951468875964,-49.5653287265562,-4.56044868974667));
#32336=CARTESIAN_POINT('Ctrl Pts',(44.5726076589586,-49.273543161918,-4.62573620901511));
#32337=CARTESIAN_POINT('Ctrl Pts',(43.7446704578678,-48.5377432669383,-4.69102372828354));
#32338=CARTESIAN_POINT('Ctrl Pts',(43.034687570683,-47.9067710952089,-4.74700988443917));
#32339=CARTESIAN_POINT('Ctrl Pts',(42.6148798756228,-46.9492878195862,-4.8029960405948));
#32340=CARTESIAN_POINT('Ctrl Pts',(42.6073208444166,-45.9976551525847,-4.85898219675043));
#32341=CARTESIAN_POINT('Ctrl Pts',(42.6053665892596,-46.0010845675542,-4.51601780324957));
#32342=CARTESIAN_POINT('Ctrl Pts',(42.605097151119,-46.0643271271258,-4.51229147867363));
#32343=CARTESIAN_POINT('Ctrl Pts',(42.6067156571417,-46.1275556359581,-4.50856515409769));
#32344=CARTESIAN_POINT('Ctrl Pts',(42.6102662023204,-46.1906754659139,-4.50483882952175));
#32345=CARTESIAN_POINT('Ctrl Pts',(42.672473957455,-47.2965740612939,-4.43955131025332));
#32346=CARTESIAN_POINT('Ctrl Pts',(43.327763921451,-48.3691112685711,-4.37426379098489));
#32347=CARTESIAN_POINT('Ctrl Pts',(44.2833978766996,-48.9291516696896,-4.30897627171646));
#32348=CARTESIAN_POINT('Ctrl Pts',(45.2390318319482,-49.4891920708081,-4.24368875244802));
#32349=CARTESIAN_POINT('Ctrl Pts',(46.4950097784494,-49.5367356657678,-4.1784012331796));
#32350=CARTESIAN_POINT('Ctrl Pts',(47.4902476695321,-49.0505432682207,-4.11311371391116));
#32351=CARTESIAN_POINT('Ctrl Pts',(48.4854855606147,-48.5643508706737,-4.04782619464273));
#32352=CARTESIAN_POINT('Ctrl Pts',(49.2199833962787,-47.5444224806199,-3.9825386753743));
#32353=CARTESIAN_POINT('Ctrl Pts',(49.3656183616491,-46.446391530422,-3.91725115610587));
#32354=CARTESIAN_POINT('Ctrl Pts',(49.5112533270196,-45.3483605802242,-3.85196363683744));
#32355=CARTESIAN_POINT('Ctrl Pts',(49.0680254220965,-44.1722270698824,-3.78667611756901));
#32356=CARTESIAN_POINT('Ctrl Pts',(48.2339382100517,-43.443406086684,-3.72138859830058));
#32357=CARTESIAN_POINT('Ctrl Pts',(47.399850998007,-42.7145851034855,-3.65610107903215));
#32358=CARTESIAN_POINT('Ctrl Pts',(46.1749044788406,-42.4330766474304,-3.59081355976371));
#32359=CARTESIAN_POINT('Ctrl Pts',(45.1063200017372,-42.7246391992172,-3.52552604049528));
#32360=CARTESIAN_POINT('Ctrl Pts',(44.0377355246337,-43.016201751004,-3.46023852122685));
#32361=CARTESIAN_POINT('Ctrl Pts',(43.1255130895933,-43.8808353106326,-3.39495100195842));
#32362=CARTESIAN_POINT('Ctrl Pts',(42.7771705717271,-44.932281467922,-3.32966348268999));
#32363=CARTESIAN_POINT('Ctrl Pts',(42.6639764192765,-45.2739496551732,-3.30844825620985));
#32364=CARTESIAN_POINT('Ctrl Pts',(42.6103240227328,-45.6353439396863,-3.28723302972971));
#32365=CARTESIAN_POINT('Ctrl Pts',(42.6129095260066,-45.9974837232043,-3.26601780324956));
#32366=CARTESIAN_POINT('Origin',(46.,-46.,-5.));
#32367=CARTESIAN_POINT('',(42.6120197259946,-46.0027475428216,-2.01601780324957));
#32368=CARTESIAN_POINT('',(42.6060559323604,-46.0016943206056,-2.35898219675043));
#32369=CARTESIAN_POINT('',(42.61025,-46.,-5.));
#32370=CARTESIAN_POINT('Ctrl Pts',(42.6060559323604,-46.0016943206056,-2.35898219675043));
#32371=CARTESIAN_POINT('Ctrl Pts',(42.6122935187612,-44.9966832429612,-2.41816666197539));
#32372=CARTESIAN_POINT('Ctrl Pts',(43.0878127283745,-43.9865345414923,-2.47735112720035));
#32373=CARTESIAN_POINT('Ctrl Pts',(43.869639312536,-43.3564767353091,-2.53653559242531));
#32374=CARTESIAN_POINT('Ctrl Pts',(44.7320872198372,-42.6614478792562,-2.60182311169374));
#32375=CARTESIAN_POINT('Ctrl Pts',(45.9672719776796,-42.4289409701107,-2.66711063096218));
#32376=CARTESIAN_POINT('Ctrl Pts',(47.0233986173667,-42.7628241355343,-2.73239815023061));
#32377=CARTESIAN_POINT('Ctrl Pts',(48.0795252570539,-43.0967073009578,-2.79768566949904));
#32378=CARTESIAN_POINT('Ctrl Pts',(48.9565937785859,-43.9969805409503,-2.86297318876747));
#32379=CARTESIAN_POINT('Ctrl Pts',(49.2627905908148,-45.0614639981771,-2.9282607080359));
#32380=CARTESIAN_POINT('Ctrl Pts',(49.5689874030437,-46.1259474554039,-2.99354822730433));
#32381=CARTESIAN_POINT('Ctrl Pts',(49.3043125059696,-47.3546411298651,-3.05883574657276));
#32382=CARTESIAN_POINT('Ctrl Pts',(48.5870043599298,-48.1986497299566,-3.12412326584119));
#32383=CARTESIAN_POINT('Ctrl Pts',(47.86969621389,-49.0426583300481,-3.18941078510962));
#32384=CARTESIAN_POINT('Ctrl Pts',(46.6997548188846,-49.5019818557699,-3.25469830437805));
#32385=CARTESIAN_POINT('Ctrl Pts',(45.5998290294583,-49.3714263208636,-3.31998582364648));
#32386=CARTESIAN_POINT('Ctrl Pts',(44.4999032400321,-49.2408707859573,-3.38527334291491));
#32387=CARTESIAN_POINT('Ctrl Pts',(43.469993056185,-48.5204361904228,-3.45056086218334));
#32388=CARTESIAN_POINT('Ctrl Pts',(42.970191096902,-47.5319628729674,-3.51584838145177));
#32389=CARTESIAN_POINT('Ctrl Pts',(42.7325322820506,-47.0619379105289,-3.54689298655132));
#32390=CARTESIAN_POINT('Ctrl Pts',(42.6147340783819,-46.5313078045718,-3.57793759165088));
#32391=CARTESIAN_POINT('Ctrl Pts',(42.6153408714561,-46.0004230001184,-3.60898219675043));
#32392=CARTESIAN_POINT('Ctrl Pts',(42.6129095260066,-45.9974837232043,-3.26601780324956));
#32393=CARTESIAN_POINT('Ctrl Pts',(42.6182806238543,-46.7497891762914,-3.22194551046127));
#32394=CARTESIAN_POINT('Ctrl Pts',(42.8663490738179,-47.505311866065,-3.17787321767298));
#32395=CARTESIAN_POINT('Ctrl Pts',(43.3274955589895,-48.093889309761,-3.13380092488469));
#32396=CARTESIAN_POINT('Ctrl Pts',(44.0106256648098,-48.9657922393603,-3.06851340561626));
#32397=CARTESIAN_POINT('Ctrl Pts',(45.1613484771422,-49.4713393436086,-3.00322588634783));
#32398=CARTESIAN_POINT('Ctrl Pts',(46.2656006877289,-49.3846873276029,-2.9379383670794));
#32399=CARTESIAN_POINT('Ctrl Pts',(47.3698528983157,-49.2980353115972,-2.87265084781097));
#32400=CARTESIAN_POINT('Ctrl Pts',(48.4276345071569,-48.6191841753375,-2.80736332854254));
#32401=CARTESIAN_POINT('Ctrl Pts',(48.9664018219562,-47.651397283792,-2.74207580927411));
#32402=CARTESIAN_POINT('Ctrl Pts',(49.5051691367556,-46.6836103922464,-2.67678829000568));
#32403=CARTESIAN_POINT('Ctrl Pts',(49.5249221575132,-45.426887745415,-2.61150077073725));
#32404=CARTESIAN_POINT('Ctrl Pts',(49.0168367155399,-44.442646794401,-2.54621325146882));
#32405=CARTESIAN_POINT('Ctrl Pts',(48.5087512735665,-43.4584058433871,-2.48092573220038));
#32406=CARTESIAN_POINT('Ctrl Pts',(47.4728273688623,-42.7466465881905,-2.41563821293195));
#32407=CARTESIAN_POINT('Ctrl Pts',(46.3718438942752,-42.6253323397915,-2.35035069366352));
#32408=CARTESIAN_POINT('Ctrl Pts',(45.2708604196881,-42.5040180913925,-2.28506317439509));
#32409=CARTESIAN_POINT('Ctrl Pts',(44.1048173752182,-42.973148849791,-2.21977565512666));
#32410=CARTESIAN_POINT('Ctrl Pts',(43.3946225937203,-43.8231524727757,-2.15448813585823));
#32411=CARTESIAN_POINT('Ctrl Pts',(42.8925311847605,-44.4240855235442,-2.10833135832201));
#32412=CARTESIAN_POINT('Ctrl Pts',(42.6182802792207,-45.2153851332211,-2.06217458078579));
#32413=CARTESIAN_POINT('Ctrl Pts',(42.6120197259946,-46.0027475428216,-2.01601780324957));
#32414=CARTESIAN_POINT('Origin',(46.,-46.,-5.));
#32415=CARTESIAN_POINT('',(42.6059703323355,-45.9984546826137,-0.766017803249566));
#32416=CARTESIAN_POINT('',(42.6118898788522,-45.9972329038001,-1.10898219675043));
#32417=CARTESIAN_POINT('',(42.61025,-46.,-5.));
#32418=CARTESIAN_POINT('',(48.5732344270147,-43.7934484719077,0.));
#32419=CARTESIAN_POINT('Ctrl Pts',(42.6059703323355,-45.9984546826137,-0.766017803249566));
#32420=CARTESIAN_POINT('Ctrl Pts',(42.6120010430613,-47.0081804904946,-0.706541093305004));
#32421=CARTESIAN_POINT('Ctrl Pts',(43.092762513117,-48.0226959853748,-0.647064383360442));
#32422=CARTESIAN_POINT('Ctrl Pts',(43.881269223622,-48.652638909118,-0.58758767341588));
#32423=CARTESIAN_POINT('Ctrl Pts',(44.7468121748606,-49.3441265655507,-0.522300154147449));
#32424=CARTESIAN_POINT('Ctrl Pts',(45.9831705630329,-49.572226239798,-0.457012634879018));
#32425=CARTESIAN_POINT('Ctrl Pts',(47.0377267586678,-49.2331399892057,-0.391725115610587));
#32426=CARTESIAN_POINT('Ctrl Pts',(48.0922829543027,-48.8940537386135,-0.326437596342156));
#32427=CARTESIAN_POINT('Ctrl Pts',(48.9650369574003,-47.9877815631816,-0.261150077073725));
#32428=CARTESIAN_POINT('Ctrl Pts',(49.2663063067355,-46.9237453887335,-0.195862557805293));
#32429=CARTESIAN_POINT('Ctrl Pts',(49.5675756560707,-45.8597092142853,-0.130575038536862));
#32430=CARTESIAN_POINT('Ctrl Pts',(49.2973603516436,-44.6379090408209,-0.065287519268431));
#32431=CARTESIAN_POINT('Ctrl Pts',(48.5732344270147,-43.7934484719077,1.57716942569499E-16));
#32432=CARTESIAN_POINT('',(43.4219943175761,-43.7905055070549,-2.82134898316155E-15));
#32433=CARTESIAN_POINT('Origin',(46.,-46.,0.));
#32434=CARTESIAN_POINT('Ctrl Pts',(43.4219651657257,-43.7904875258606,-1.80411241501588E-15));
#32435=CARTESIAN_POINT('Ctrl Pts',(44.1103019067085,-42.9932828189542,-0.0620616329205985));
#32436=CARTESIAN_POINT('Ctrl Pts',(45.2006369367306,-42.5364250742059,-0.124123265841195));
#32437=CARTESIAN_POINT('Ctrl Pts',(46.2508550217425,-42.6143560679205,-0.186184898761792));
#32438=CARTESIAN_POINT('Ctrl Pts',(47.3556621341977,-42.6963378175832,-0.251472418030223));
#32439=CARTESIAN_POINT('Ctrl Pts',(48.4160734564188,-43.3701484975484,-0.316759937298653));
#32440=CARTESIAN_POINT('Ctrl Pts',(48.9590107118729,-44.3354564297113,-0.382047456567084));
#32441=CARTESIAN_POINT('Ctrl Pts',(49.501947967327,-45.3007643618741,-0.447334975835515));
#32442=CARTESIAN_POINT('Ctrl Pts',(49.5274111560141,-46.5575695462346,-0.512622495103946));
#32443=CARTESIAN_POINT('Ctrl Pts',(49.0237120278267,-47.5440867715274,-0.577910014372376));
#32444=CARTESIAN_POINT('Ctrl Pts',(48.5200128996393,-48.5306039968202,-0.643197533640807));
#32445=CARTESIAN_POINT('Ctrl Pts',(47.4871514545773,-49.2468332630454,-0.708485052909238));
#32446=CARTESIAN_POINT('Ctrl Pts',(46.3866918750129,-49.372975105968,-0.773772572177669));
#32447=CARTESIAN_POINT('Ctrl Pts',(45.2862322954484,-49.4991169488906,-0.8390600914461));
#32448=CARTESIAN_POINT('Ctrl Pts',(44.1181745813813,-49.0351713685107,-0.904347610714531));
#32449=CARTESIAN_POINT('Ctrl Pts',(43.404251173025,-48.1883177881507,-0.969635129982962));
#32450=CARTESIAN_POINT('Ctrl Pts',(42.8963279948238,-47.5858209979168,-1.01608415223878));
#32451=CARTESIAN_POINT('Ctrl Pts',(42.618272082018,-46.7895092640711,-1.06253317449461));
#32452=CARTESIAN_POINT('Ctrl Pts',(42.6118898788522,-45.9972329038001,-1.10898219675043));
#32453=CARTESIAN_POINT('Origin',(46.,-46.,2.76038497140452));
#32454=CARTESIAN_POINT('',(41.9196909029574,-45.9976755478274,-7.76038497140452));
#32455=CARTESIAN_POINT('',(41.9137289353857,-46.0033881484067,-7.86461502859548));
#32456=CARTESIAN_POINT('',(41.915,-45.9999999999999,2.76038497140452));
#32457=CARTESIAN_POINT('',(42.5743852316216,-48.2253962475631,-9.));
#32458=CARTESIAN_POINT('Ctrl Pts',(41.9137289353857,-46.0033881484067,-7.86461502859549));
#32459=CARTESIAN_POINT('Ctrl Pts',(41.9230935686005,-44.9361783803566,-7.91663908938817));
#32460=CARTESIAN_POINT('Ctrl Pts',(42.891985057322,-42.5144885624548,-8.03395066944928));
#32461=CARTESIAN_POINT('Ctrl Pts',(46.947226477628,-41.2871007943775,-8.21654976877883));
#32462=CARTESIAN_POINT('Ctrl Pts',(50.4487171774031,-44.1804056791643,-8.41241232658412));
#32463=CARTESIAN_POINT('Ctrl Pts',(49.979557221961,-48.7013821925377,-8.60827488438941));
#32464=CARTESIAN_POINT('Ctrl Pts',(45.946358746692,-50.8047710666759,-8.80413744219471));
#32465=CARTESIAN_POINT('Ctrl Pts',(43.3046954441484,-49.3495832107922,-8.93471248073157));
#32466=CARTESIAN_POINT('Ctrl Pts',(42.5743852316216,-48.2253962475631,-9.));
#32467=CARTESIAN_POINT('',(41.9138451336777,-46.212441516533,-8.99999999999999));
#32468=CARTESIAN_POINT('Origin',(46.,-46.,-9.));
#32469=CARTESIAN_POINT('Ctrl Pts',(41.9196909029574,-45.9976755478274,-7.76038497140452));
#32470=CARTESIAN_POINT('Ctrl Pts',(41.9169749126423,-45.4889856236339,-7.78509075167359));
#32471=CARTESIAN_POINT('Ctrl Pts',(42.2389226908427,-43.6393407000909,-7.8750840512111));
#32472=CARTESIAN_POINT('Ctrl Pts',(44.9804152684286,-41.3020771440901,-8.03036487001703));
#32473=CARTESIAN_POINT('Ctrl Pts',(49.3490847557137,-42.5514377898613,-8.22622742782233));
#32474=CARTESIAN_POINT('Ctrl Pts',(50.7259989091243,-46.8818733140433,-8.42208998562761));
#32475=CARTESIAN_POINT('Ctrl Pts',(47.8793446557761,-50.4245587866615,-8.61795254343292));
#32476=CARTESIAN_POINT('Ctrl Pts',(43.4302591581606,-50.0204898973754,-8.81058921489037));
#32477=CARTESIAN_POINT('Ctrl Pts',(41.9843544528723,-47.4797545535775,-8.9379383670794));
#32478=CARTESIAN_POINT('Ctrl Pts',(41.9138040800513,-46.2124372338608,-9.));
#32479=CARTESIAN_POINT('Origin',(46.,-46.,2.76038497140452));
#32480=CARTESIAN_POINT('',(41.9151416908186,-46.0034858728755,-6.51038497140452));
#32481=CARTESIAN_POINT('',(41.912796133594,-45.9967790955024,-6.61461502859548));
#32482=CARTESIAN_POINT('',(41.915,-45.9999999999999,2.76038497140452));
#32483=CARTESIAN_POINT('Ctrl Pts',(41.912796133594,-45.9967790955024,-6.61461502859548));
#32484=CARTESIAN_POINT('Ctrl Pts',(41.9107304308479,-45.7573638992105,-6.62629312117581));
#32485=CARTESIAN_POINT('Ctrl Pts',(42.0377964723628,-44.1816628889412,-6.70325873302458));
#32486=CARTESIAN_POINT('Ctrl Pts',(44.0829608206919,-41.591478562833,-6.84551186414177));
#32487=CARTESIAN_POINT('Ctrl Pts',(48.6116788957116,-41.9640100582522,-7.04137442194706));
#32488=CARTESIAN_POINT('Ctrl Pts',(50.8069346691015,-45.9425306737833,-7.23723697975236));
#32489=CARTESIAN_POINT('Ctrl Pts',(48.7074348723187,-49.9724245030734,-7.43309953755765));
#32490=CARTESIAN_POINT('Ctrl Pts',(44.1888312987275,-50.4530551698565,-7.62896209536294));
#32491=CARTESIAN_POINT('Ctrl Pts',(42.0589980216041,-47.8842560929907,-7.77280059237556));
#32492=CARTESIAN_POINT('Ctrl Pts',(41.9113414357962,-46.2754717233481,-7.85135157011974));
#32493=CARTESIAN_POINT('Ctrl Pts',(41.9137289353857,-46.0033881484067,-7.86461502859549));
#32494=CARTESIAN_POINT('Ctrl Pts',(41.9151416908186,-46.0034858728755,-6.51038497140452));
#32495=CARTESIAN_POINT('Ctrl Pts',(41.9240606763713,-44.9841466877243,-6.56003230272967));
#32496=CARTESIAN_POINT('Ctrl Pts',(42.8214698193968,-42.6103273354142,-6.67496715332326));
#32497=CARTESIAN_POINT('Ctrl Pts',(46.777185224748,-41.255945113868,-6.85518952318527));
#32498=CARTESIAN_POINT('Ctrl Pts',(50.3817996987672,-44.0226574502926,-7.05105208099057));
#32499=CARTESIAN_POINT('Ctrl Pts',(50.071451482069,-48.5560483299491,-7.24691463879586));
#32500=CARTESIAN_POINT('Ctrl Pts',(46.1234029447301,-50.8057104508671,-7.44277719660115));
#32501=CARTESIAN_POINT('Ctrl Pts',(42.5770326391767,-49.01948437455,-7.61393397413737));
#32502=CARTESIAN_POINT('Ctrl Pts',(41.9241521913235,-46.8332501182475,-7.71980323240516));
#32503=CARTESIAN_POINT('Ctrl Pts',(41.9196909029574,-45.9976755478274,-7.76038497140452));
#32504=CARTESIAN_POINT('Origin',(46.,-46.,2.76038497140452));
#32505=CARTESIAN_POINT('',(41.9114700639993,-45.9971742158887,-5.26038497140452));
#32506=CARTESIAN_POINT('',(41.9208126398586,-46.001244625712,-5.36461502859548));
#32507=CARTESIAN_POINT('',(41.915,-45.9999999999999,2.76038497140452));
#32508=CARTESIAN_POINT('Ctrl Pts',(41.9208126398586,-46.001244625712,-5.36461502859548));
#32509=CARTESIAN_POINT('Ctrl Pts',(41.9229286932863,-45.2467318609778,-5.40123467223189));
#32510=CARTESIAN_POINT('Ctrl Pts',(42.4823083976697,-43.1441149653643,-5.50314183513673));
#32511=CARTESIAN_POINT('Ctrl Pts',(45.8362350648755,-41.1954966730761,-5.67033651731001));
#32512=CARTESIAN_POINT('Ctrl Pts',(49.9115574163095,-43.2053998426678,-5.86619907511531));
#32513=CARTESIAN_POINT('Ctrl Pts',(50.4920529547756,-47.7121708254118,-6.0620616329206));
#32514=CARTESIAN_POINT('Ctrl Pts',(47.0590723399817,-50.6891832485807,-6.25792419072589));
#32515=CARTESIAN_POINT('Ctrl Pts',(42.9409560641467,-49.5488892301137,-6.44210865595086));
#32516=CARTESIAN_POINT('Ctrl Pts',(41.9222789441782,-47.0958379807898,-6.56100560190738));
#32517=CARTESIAN_POINT('Ctrl Pts',(41.912796133594,-45.9967790955024,-6.61461502859548));
#32518=CARTESIAN_POINT('Ctrl Pts',(41.9114700639993,-45.9971742158887,-5.26038497140452));
#32519=CARTESIAN_POINT('Ctrl Pts',(41.9099566544234,-45.8066458331328,-5.26968633451732));
#32520=CARTESIAN_POINT('Ctrl Pts',(42.0077825243435,-44.2803336702357,-5.34427521689855));
#32521=CARTESIAN_POINT('Ctrl Pts',(43.9262270571184,-41.6630037489246,-5.48415161854821));
#32522=CARTESIAN_POINT('Ctrl Pts',(48.4653741677054,-41.8730155103115,-5.68001417635351));
#32523=CARTESIAN_POINT('Ctrl Pts',(50.8018040255352,-45.7703295385275,-5.8758767341588));
#32524=CARTESIAN_POINT('Ctrl Pts',(48.8480063650781,-49.8728452943253,-6.0717392919641));
#32525=CARTESIAN_POINT('Ctrl Pts',(44.349624114825,-50.5151224407608,-6.26760184976939));
#32526=CARTESIAN_POINT('Ctrl Pts',(42.0922727086059,-47.9830688501961,-6.41381707624953));
#32527=CARTESIAN_POINT('Ctrl Pts',(41.9123319806774,-46.3246039674072,-6.49474478346124));
#32528=CARTESIAN_POINT('Ctrl Pts',(41.9151416908186,-46.0034858728755,-6.51038497140452));
#32529=CARTESIAN_POINT('Origin',(46.,-46.,2.76038497140452));
#32530=CARTESIAN_POINT('',(41.9211350276268,-46.0005097589745,-4.01038497140452));
#32531=CARTESIAN_POINT('',(41.9091149840328,-46.0013070162871,-4.11461502859548));
#32532=CARTESIAN_POINT('',(41.915,-45.9999999999999,2.76038497140452));
#32533=CARTESIAN_POINT('Ctrl Pts',(41.9091149840328,-46.0013070162871,-4.11461502859548));
#32534=CARTESIAN_POINT('Ctrl Pts',(41.9144792440739,-44.7422071186988,-4.17617622328797));
#32535=CARTESIAN_POINT('Ctrl Pts',(43.2050471763048,-42.1382708909912,-4.30302493724889));
#32536=CARTESIAN_POINT('Ctrl Pts',(47.6123998603384,-41.4711770162521,-4.49516117047826));
#32537=CARTESIAN_POINT('Ctrl Pts',(50.6646121398881,-44.8374749372802,-4.69102372828354));
#32538=CARTESIAN_POINT('Ctrl Pts',(49.5491724822373,-49.2424443845602,-4.88688628608884));
#32539=CARTESIAN_POINT('Ctrl Pts',(45.2626834297744,-50.7504142155033,-5.08274884389412));
#32540=CARTESIAN_POINT('Ctrl Pts',(42.3132197363476,-48.5256744077654,-5.24199175806301));
#32541=CARTESIAN_POINT('Ctrl Pts',(41.9191560765917,-46.5919188091348,-5.33594715296346));
#32542=CARTESIAN_POINT('Ctrl Pts',(41.9208126398586,-46.001244625712,-5.36461502859548));
#32543=CARTESIAN_POINT('Ctrl Pts',(41.9211350276268,-46.0005097589745,-4.01038497140452));
#32544=CARTESIAN_POINT('Ctrl Pts',(41.9219416115921,-45.294827395514,-4.0446278855734));
#32545=CARTESIAN_POINT('Ctrl Pts',(42.428887780726,-43.242606030091,-4.14415831901071));
#32546=CARTESIAN_POINT('Ctrl Pts',(45.6641826146291,-41.204450252827,-4.30897627171645));
#32547=CARTESIAN_POINT('Ctrl Pts',(49.8089076312337,-43.0670333548852,-4.50483882952175));
#32548=CARTESIAN_POINT('Ctrl Pts',(50.5505198521649,-47.5501095932216,-4.70070138732704));
#32549=CARTESIAN_POINT('Ctrl Pts',(47.2264172239299,-50.6482223997432,-4.89656394513234));
#32550=CARTESIAN_POINT('Ctrl Pts',(43.0164536107202,-49.6434230598024,-5.08312513982483));
#32551=CARTESIAN_POINT('Ctrl Pts',(41.9205794798788,-47.1439901889548,-5.20439881524889));
#32552=CARTESIAN_POINT('Ctrl Pts',(41.9114700639993,-45.9971742158887,-5.26038497140452));
#32553=CARTESIAN_POINT('Origin',(46.,-46.,2.76038497140452));
#32554=CARTESIAN_POINT('',(41.9099457138999,-46.0020418318974,-2.76038497140452));
#32555=CARTESIAN_POINT('',(41.9182050044213,-45.9969676257214,-2.86461502859548));
#32556=CARTESIAN_POINT('',(41.915,-45.9999999999999,2.76038497140452));
#32557=CARTESIAN_POINT('Ctrl Pts',(41.9182050044213,-45.9969676257214,-2.86461502859548));
#32558=CARTESIAN_POINT('Ctrl Pts',(41.9150892050634,-45.5605516612194,-2.88583025507562));
#32559=CARTESIAN_POINT('Ctrl Pts',(42.178719756358,-43.7847768478177,-2.97233300082419));
#32560=CARTESIAN_POINT('Ctrl Pts',(44.7345905347796,-41.3622408914429,-3.12412326584119));
#32561=CARTESIAN_POINT('Ctrl Pts',(49.1631529928913,-42.3799814708233,-3.31998582364649));
#32562=CARTESIAN_POINT('Ctrl Pts',(50.765559652625,-46.6320697278449,-3.51584838145178));
#32563=CARTESIAN_POINT('Ctrl Pts',(48.1101216480341,-50.3194279165342,-3.71171093925708));
#32564=CARTESIAN_POINT('Ctrl Pts',(43.5693709335647,-50.1475430411802,-3.90757349706237));
#32565=CARTESIAN_POINT('Ctrl Pts',(41.9449141512117,-47.488734824337,-4.04187486017517));
#32566=CARTESIAN_POINT('Ctrl Pts',(41.9087902831539,-46.0775208538414,-4.11088870401954));
#32567=CARTESIAN_POINT('Ctrl Pts',(41.9091149840328,-46.0013070162871,-4.11461502859548));
#32568=CARTESIAN_POINT('Ctrl Pts',(41.9099457138999,-46.0020418318974,-2.76038497140452));
#32569=CARTESIAN_POINT('Ctrl Pts',(41.9174626518591,-44.7908993428709,-2.81956943662948));
#32570=CARTESIAN_POINT('Ctrl Pts',(43.1226549378218,-42.230701146723,-2.94404142112287));
#32571=CARTESIAN_POINT('Ctrl Pts',(47.4490849663269,-41.4163089133544,-3.13380092488469));
#32572=CARTESIAN_POINT('Ctrl Pts',(50.6199603203723,-44.6710765381374,-3.32966348268999));
#32573=CARTESIAN_POINT('Ctrl Pts',(49.6630782896489,-49.1131861274939,-3.52552604049528));
#32574=CARTESIAN_POINT('Ctrl Pts',(45.433376454472,-50.7737834599584,-3.72138859830057));
#32575=CARTESIAN_POINT('Ctrl Pts',(42.3609059541842,-48.6245532873833,-3.88300824193699));
#32576=CARTESIAN_POINT('Ctrl Pts',(41.9204037790959,-46.6402809592672,-3.97934036630497));
#32577=CARTESIAN_POINT('Ctrl Pts',(41.9211350276268,-46.0005097589745,-4.01038497140452));
#32578=CARTESIAN_POINT('Origin',(46.,-46.,2.76038497140452));
#32579=CARTESIAN_POINT('',(41.9169762239431,-45.9966653623493,-1.51038497140452));
#32580=CARTESIAN_POINT('',(41.9171327032046,-46.0033110738038,-1.61461502859548));
#32581=CARTESIAN_POINT('',(41.915,-45.9999999999999,2.76038497140452));
#32582=CARTESIAN_POINT('Ctrl Pts',(41.9171327032046,-46.0033110738038,-1.61461502859548));
#32583=CARTESIAN_POINT('Ctrl Pts',(41.9246773185682,-45.0544577827888,-1.6607718061317));
#32584=CARTESIAN_POINT('Ctrl Pts',(42.7226625049108,-42.7520210224136,-1.77221610293635));
#32585=CARTESIAN_POINT('Ctrl Pts',(46.5265139467765,-41.2216283664815,-1.94894791900943));
#32586=CARTESIAN_POINT('Ctrl Pts',(50.2717008933508,-43.7948593340848,-2.14481047681473));
#32587=CARTESIAN_POINT('Ctrl Pts',(50.2002875828164,-48.338302371748,-2.34067303462002));
#32588=CARTESIAN_POINT('Ctrl Pts',(46.3760782410217,-50.7925602594573,-2.53653559242531));
#32589=CARTESIAN_POINT('Ctrl Pts',(42.6664797940018,-49.1628222089761,-2.71118292375047));
#32590=CARTESIAN_POINT('Ctrl Pts',(41.9246777338874,-46.9035736514935,-2.82054273580719));
#32591=CARTESIAN_POINT('Ctrl Pts',(41.9182050044213,-45.9969676257214,-2.86461502859548));
#32592=CARTESIAN_POINT('Ctrl Pts',(41.9169762239431,-45.9966653623493,-1.51038497140452));
#32593=CARTESIAN_POINT('Ctrl Pts',(41.9138568697487,-45.6094337867792,-1.52922346841713));
#32594=CARTESIAN_POINT('Ctrl Pts',(42.1404160610226,-43.8837676902663,-1.61334948469817));
#32595=CARTESIAN_POINT('Ctrl Pts',(44.5692320816632,-41.4105744865513,-1.76276302024764));
#32596=CARTESIAN_POINT('Ctrl Pts',(49.0314013549138,-42.268956305567,-1.95862557805293));
#32597=CARTESIAN_POINT('Ctrl Pts',(50.7851507003408,-46.4609045572623,-2.15448813585823));
#32598=CARTESIAN_POINT('Ctrl Pts',(48.263541336862,-50.2410414729541,-2.35035069366352));
#32599=CARTESIAN_POINT('Ctrl Pts',(43.7195496474102,-50.2319758772438,-2.54621325146881));
#32600=CARTESIAN_POINT('Ctrl Pts',(41.9704479226572,-47.5870902922536,-2.68289134404915));
#32601=CARTESIAN_POINT('Ctrl Pts',(41.9091705733553,-46.1269338628851,-2.75428191736105));
#32602=CARTESIAN_POINT('Ctrl Pts',(41.9099457138999,-46.0020418318974,-2.76038497140452));
#32603=CARTESIAN_POINT('Origin',(46.,-46.,2.76038497140452));
#32604=CARTESIAN_POINT('',(41.9194196464784,-46.0038358614086,-0.260384971404518));
#32605=CARTESIAN_POINT('',(41.9098425569998,-45.9981377324218,-0.364615028595479));
#32606=CARTESIAN_POINT('',(41.915,-45.9999999999999,2.76038497140452));
#32607=CARTESIAN_POINT('',(44.942095577027,-49.9456385074984,0.));
#32608=CARTESIAN_POINT('Ctrl Pts',(44.942095577027,-49.9456385074984,5.55111512312578E-16));
#32609=CARTESIAN_POINT('Ctrl Pts',(43.6472519732776,-49.5984650974504,-0.0652875192684306));
#32610=CARTESIAN_POINT('Ctrl Pts',(42.1846929797356,-48.2273651784823,-0.152082509736603));
#32611=CARTESIAN_POINT('Ctrl Pts',(41.9164508003806,-46.4463095999464,-0.238877500204776));
#32612=CARTESIAN_POINT('Ctrl Pts',(41.9194196464784,-46.0038358614086,-0.260384971404518));
#32613=CARTESIAN_POINT('',(47.0606474189675,-49.9518122604704,1.27273922847335E-15));
#32614=CARTESIAN_POINT('Origin',(46.,-46.,0.));
#32615=CARTESIAN_POINT('Ctrl Pts',(47.0606641786102,-49.9518499819597,3.86518074491082E-16));
#32616=CARTESIAN_POINT('Ctrl Pts',(45.8335725344782,-50.2763751643415,-0.0620616329205975));
#32617=CARTESIAN_POINT('Ctrl Pts',(43.101024906791,-49.7132899277509,-0.183599975785757));
#32618=CARTESIAN_POINT('Ctrl Pts',(41.917110188334,-47.2149619599294,-0.305138318650917));
#32619=CARTESIAN_POINT('Ctrl Pts',(41.9098425569998,-45.9981377324218,-0.364615028595479));
#32620=CARTESIAN_POINT('Origin',(-46.,46.,-5.));
#32621=CARTESIAN_POINT('',(-49.390804277264,45.9971884954151,-8.26601780324957));
#32622=CARTESIAN_POINT('',(-49.3955878307095,45.9998426774376,-8.60898219675043));
#32623=CARTESIAN_POINT('',(-49.38975,46.,-5.));
#32624=CARTESIAN_POINT('',(-44.696617959125,49.1291532909119,-9.));
#32625=CARTESIAN_POINT('Ctrl Pts',(-49.3955878307095,45.9998426774376,-8.60898219675043));
#32626=CARTESIAN_POINT('Ctrl Pts',(-49.3946787862589,47.103578210484,-8.67403394523185));
#32627=CARTESIAN_POINT('Ctrl Pts',(-48.8034231054609,48.2078784353154,-8.73908569371328));
#32628=CARTESIAN_POINT('Ctrl Pts',(-47.8878799940434,48.8209858903891,-8.8041374421947));
#32629=CARTESIAN_POINT('Ctrl Pts',(-46.9690186271608,49.4363154660142,-8.86942496146314));
#32630=CARTESIAN_POINT('Ctrl Pts',(-45.723514902722,49.5568853032748,-8.93471248073157));
#32631=CARTESIAN_POINT('Ctrl Pts',(-44.696617959125,49.1291532909119,-9.));
#32632=CARTESIAN_POINT('',(-49.38975,46.,-9.));
#32633=CARTESIAN_POINT('Origin',(-46.,46.,-9.));
#32634=CARTESIAN_POINT('',(-49.38975,46.,-10.));
#32635=CARTESIAN_POINT('',(-49.38975,46.,-5.));
#32636=CARTESIAN_POINT('Origin',(-46.,46.,-10.));
#32637=CARTESIAN_POINT('',(-43.101998404785,44.230942529973,-9.00000000000001));
#32638=CARTESIAN_POINT('Origin',(-46.,46.,-9.));
#32639=CARTESIAN_POINT('Ctrl Pts',(-43.1019723047815,44.2309203707046,-9.00000000000001));
#32640=CARTESIAN_POINT('Ctrl Pts',(-42.5564929566499,45.1319175212271,-8.93793836707941));
#32641=CARTESIAN_POINT('Ctrl Pts',(-42.4589283016514,46.3100640648579,-8.87587673415881));
#32642=CARTESIAN_POINT('Ctrl Pts',(-42.8575804387187,47.2847985850388,-8.81381510123821));
#32643=CARTESIAN_POINT('Ctrl Pts',(-43.2769540171336,48.3101985910188,-8.74852758196978));
#32644=CARTESIAN_POINT('Ctrl Pts',(-44.2454705226989,49.1104907897642,-8.68324006270135));
#32645=CARTESIAN_POINT('Ctrl Pts',(-45.3313095094966,49.3285582706994,-8.61795254343292));
#32646=CARTESIAN_POINT('Ctrl Pts',(-46.4171484962944,49.5466257516345,-8.55266502416448));
#32647=CARTESIAN_POINT('Ctrl Pts',(-47.6203099643246,49.1824685147595,-8.48737750489605));
#32648=CARTESIAN_POINT('Ctrl Pts',(-48.4028919771909,48.3985716685866,-8.42208998562762));
#32649=CARTESIAN_POINT('Ctrl Pts',(-49.0264888708823,47.773927055995,-8.37006592483494));
#32650=CARTESIAN_POINT('Ctrl Pts',(-49.383033529559,46.8827634791248,-8.31804186404225));
#32651=CARTESIAN_POINT('Ctrl Pts',(-49.390804277264,45.9971884954151,-8.26601780324957));
#32652=CARTESIAN_POINT('Origin',(-46.,46.,-5.));
#32653=CARTESIAN_POINT('',(-49.3915783323198,46.002672719373,-7.01601780324957));
#32654=CARTESIAN_POINT('',(-49.3858580102862,46.0019288502567,-7.35898219675043));
#32655=CARTESIAN_POINT('',(-49.38975,46.,-5.));
#32656=CARTESIAN_POINT('Ctrl Pts',(-49.3858580102862,46.0019288502567,-7.35898219675043));
#32657=CARTESIAN_POINT('Ctrl Pts',(-49.3881117467423,46.4240419378505,-7.3836879770195));
#32658=CARTESIAN_POINT('Ctrl Pts',(-49.314770291966,46.8454011027671,-7.40839375728858));
#32659=CARTESIAN_POINT('Ctrl Pts',(-49.1621985550924,47.2357983892983,-7.43309953755765));
#32660=CARTESIAN_POINT('Ctrl Pts',(-48.7590123329831,48.2674626431351,-7.49838705682608));
#32661=CARTESIAN_POINT('Ctrl Pts',(-47.8025341154912,49.0829095742609,-7.56367457609451));
#32662=CARTESIAN_POINT('Ctrl Pts',(-46.7201048386092,49.3178456032442,-7.62896209536294));
#32663=CARTESIAN_POINT('Ctrl Pts',(-45.6376755617271,49.5527816322275,-7.69424961463137));
#32664=CARTESIAN_POINT('Ctrl Pts',(-44.4292952254548,49.2072067590683,-7.75953713389981));
#32665=CARTESIAN_POINT('Ctrl Pts',(-43.6346769280645,48.4355169169347,-7.82482465316824));
#32666=CARTESIAN_POINT('Ctrl Pts',(-42.8400586306741,47.663827074801,-7.89011217243667));
#32667=CARTESIAN_POINT('Ctrl Pts',(-42.4592023721657,46.4660222636928,-7.9553996917051));
#32668=CARTESIAN_POINT('Ctrl Pts',(-42.6624684232406,45.3771640589127,-8.02068721097353));
#32669=CARTESIAN_POINT('Ctrl Pts',(-42.8657344743155,44.2883058541325,-8.08597473024196));
#32670=CARTESIAN_POINT('Ctrl Pts',(-43.6531228349737,43.3083942556804,-8.15126224951039));
#32671=CARTESIAN_POINT('Ctrl Pts',(-44.6724329422056,42.8752570111787,-8.21654976877882));
#32672=CARTESIAN_POINT('Ctrl Pts',(-45.6917430494375,42.4421197666769,-8.28183728804725));
#32673=CARTESIAN_POINT('Ctrl Pts',(-46.942974903243,42.5557568761255,-8.34712480731569));
#32674=CARTESIAN_POINT('Ctrl Pts',(-47.8680862672342,43.1652560477182,-8.41241232658412));
#32675=CARTESIAN_POINT('Ctrl Pts',(-48.7931976312253,43.7747552193109,-8.47769984585255));
#32676=CARTESIAN_POINT('Ctrl Pts',(-49.3921885054021,44.8801164530478,-8.54298736512098));
#32677=CARTESIAN_POINT('Ctrl Pts',(-49.3955744378273,45.9878417269111,-8.60827488438941));
#32678=CARTESIAN_POINT('Ctrl Pts',(-49.3955866653397,45.9918420207273,-8.60851065517642));
#32679=CARTESIAN_POINT('Ctrl Pts',(-49.3955911254115,45.9958423453736,-8.60874642596342));
#32680=CARTESIAN_POINT('Ctrl Pts',(-49.3955878307095,45.9998426774376,-8.60898219675043));
#32681=CARTESIAN_POINT('Ctrl Pts',(-49.390804277264,45.9971884954151,-8.26601780324957));
#32682=CARTESIAN_POINT('Ctrl Pts',(-49.3927854180658,45.7714124440146,-8.25275434477382));
#32683=CARTESIAN_POINT('Ctrl Pts',(-49.3720966873643,45.5459996442359,-8.23949088629808));
#32684=CARTESIAN_POINT('Ctrl Pts',(-49.327383847567,45.3254592826471,-8.22622742782233));
#32685=CARTESIAN_POINT('Ctrl Pts',(-49.1072911473747,44.2398801983513,-8.1609399085539));
#32686=CARTESIAN_POINT('Ctrl Pts',(-48.305103189288,43.2723584852303,-8.09565238928547));
#32687=CARTESIAN_POINT('Ctrl Pts',(-47.2790832574686,42.8550691740869,-8.03036487001704));
#32688=CARTESIAN_POINT('Ctrl Pts',(-46.2530633256491,42.4377798629434,-7.96507735074861));
#32689=CARTESIAN_POINT('Ctrl Pts',(-45.003211420097,42.5707229537774,-7.89978983148017));
#32690=CARTESIAN_POINT('Ctrl Pts',(-44.0879232413465,43.1945315388044,-7.83450231221174));
#32691=CARTESIAN_POINT('Ctrl Pts',(-43.1726350625961,43.8183401238314,-7.76921479294331));
#32692=CARTESIAN_POINT('Ctrl Pts',(-42.5919106106473,44.9330142030514,-7.70392727367488));
#32693=CARTESIAN_POINT('Ctrl Pts',(-42.6051537334803,46.0405833305628,-7.63863975440645));
#32694=CARTESIAN_POINT('Ctrl Pts',(-42.6183968563134,47.1481524580742,-7.57335223513801));
#32695=CARTESIAN_POINT('Ctrl Pts',(-43.2256075539281,48.2486166338769,-7.50806471586958));
#32696=CARTESIAN_POINT('Ctrl Pts',(-44.1555376756467,48.8503700797306,-7.44277719660115));
#32697=CARTESIAN_POINT('Ctrl Pts',(-45.0854677973652,49.4521235255844,-7.37748967733272));
#32698=CARTESIAN_POINT('Ctrl Pts',(-46.3381173431877,49.5551662414892,-7.31220215806429));
#32699=CARTESIAN_POINT('Ctrl Pts',(-47.3538834999244,49.1134631917099,-7.24691463879586));
#32700=CARTESIAN_POINT('Ctrl Pts',(-48.3696496566611,48.6717601419306,-7.18162711952743));
#32701=CARTESIAN_POINT('Ctrl Pts',(-49.1485324243119,47.6853113264672,-7.116339600259));
#32702=CARTESIAN_POINT('Ctrl Pts',(-49.3425836444144,46.5947951363276,-7.05105208099057));
#32703=CARTESIAN_POINT('Ctrl Pts',(-49.3772939250174,46.3997326010758,-7.03937398841023));
#32704=CARTESIAN_POINT('Ctrl Pts',(-49.3932924608325,46.201340419597,-7.0276958958299));
#32705=CARTESIAN_POINT('Ctrl Pts',(-49.3915783323198,46.002672719373,-7.01601780324957));
#32706=CARTESIAN_POINT('Origin',(-46.,46.,-5.));
#32707=CARTESIAN_POINT('',(-49.3849262043165,45.9989672045366,-5.76601780324957));
#32708=CARTESIAN_POINT('',(-49.3896329814502,45.9971074077133,-6.10898219675043));
#32709=CARTESIAN_POINT('',(-49.38975,46.,-5.));
#32710=CARTESIAN_POINT('Ctrl Pts',(-49.3896329814502,45.9971074077133,-6.10898219675043));
#32711=CARTESIAN_POINT('Ctrl Pts',(-49.3822319686501,46.8429594447226,-6.15862952807558));
#32712=CARTESIAN_POINT('Ctrl Pts',(-49.0605621281795,47.6938378847277,-6.20827685940074));
#32713=CARTESIAN_POINT('Ctrl Pts',(-48.4872411182123,48.3109063253483,-6.25792419072589));
#32714=CARTESIAN_POINT('Ctrl Pts',(-47.7333092252755,49.122367216229,-6.32321170999432));
#32715=CARTESIAN_POINT('Ctrl Pts',(-46.5441987940589,49.5295021746259,-6.38849922926275));
#32716=CARTESIAN_POINT('Ctrl Pts',(-45.4511228133513,49.3504313564188,-6.45378674853118));
#32717=CARTESIAN_POINT('Ctrl Pts',(-44.3580468326437,49.1713605382117,-6.51907426779961));
#32718=CARTESIAN_POINT('Ctrl Pts',(-43.3610053024451,48.4060839434005,-6.58436178706805));
#32719=CARTESIAN_POINT('Ctrl Pts',(-42.9054059204164,47.3964744387992,-6.64964930633648));
#32720=CARTESIAN_POINT('Ctrl Pts',(-42.4498065383877,46.3868649341978,-6.71493682560491));
#32721=CARTESIAN_POINT('Ctrl Pts',(-42.5356493045288,45.1329225198063,-6.78022434487333));
#32722=CARTESIAN_POINT('Ctrl Pts',(-43.1245886239275,44.19482143211,-6.84551186414177));
#32723=CARTESIAN_POINT('Ctrl Pts',(-43.7135279433262,43.2567203444137,-6.9107993834102));
#32724=CARTESIAN_POINT('Ctrl Pts',(-44.8055638159825,42.6344605834126,-6.97608690267863));
#32725=CARTESIAN_POINT('Ctrl Pts',(-45.9128440093134,42.6060257295712,-7.04137442194706));
#32726=CARTESIAN_POINT('Ctrl Pts',(-47.0201242026443,42.5775908757298,-7.1066619412155));
#32727=CARTESIAN_POINT('Ctrl Pts',(-48.1426487166498,43.142980929048,-7.17194946048392));
#32728=CARTESIAN_POINT('Ctrl Pts',(-48.7789638602892,44.049616743981,-7.23723697975235));
#32729=CARTESIAN_POINT('Ctrl Pts',(-49.1744877731268,44.6131679161094,-7.27781871875171));
#32730=CARTESIAN_POINT('Ctrl Pts',(-49.3821560205639,45.3085654768932,-7.31840045775107));
#32731=CARTESIAN_POINT('Ctrl Pts',(-49.3858580102862,46.0019288502567,-7.35898219675043));
#32732=CARTESIAN_POINT('Ctrl Pts',(-49.3915783323198,46.002672719373,-7.01601780324957));
#32733=CARTESIAN_POINT('Ctrl Pts',(-49.3837094576552,45.0906692019163,-6.96240837656147));
#32734=CARTESIAN_POINT('Ctrl Pts',(-49.0025711816212,44.1728595157671,-6.90879894987337));
#32735=CARTESIAN_POINT('Ctrl Pts',(-48.3448149181929,43.5447010853554,-6.85518952318527));
#32736=CARTESIAN_POINT('Ctrl Pts',(-47.5437752993149,42.7797067893384,-6.78990200391684));
#32737=CARTESIAN_POINT('Ctrl Pts',(-46.3324763890047,42.4443017621203,-6.72461448464841));
#32738=CARTESIAN_POINT('Ctrl Pts',(-45.2520433961537,42.6883220776615,-6.65932696537998));
#32739=CARTESIAN_POINT('Ctrl Pts',(-44.1716104033028,42.9323423932026,-6.59403944611155));
#32740=CARTESIAN_POINT('Ctrl Pts',(-43.2220433279111,43.7557880515031,-6.52875192684312));
#32741=CARTESIAN_POINT('Ctrl Pts',(-42.827542715153,44.7908003518449,-6.46346440757469));
#32742=CARTESIAN_POINT('Ctrl Pts',(-42.4330421023949,45.8258126521868,-6.39817688830625));
#32743=CARTESIAN_POINT('Ctrl Pts',(-42.5936079522705,47.07239159457,-6.33288936903782));
#32744=CARTESIAN_POINT('Ctrl Pts',(-43.2375107113618,47.9736520318194,-6.26760184976939));
#32745=CARTESIAN_POINT('Ctrl Pts',(-43.881413470453,48.8749124690688,-6.20231433050096));
#32746=CARTESIAN_POINT('Ctrl Pts',(-45.00865313876,49.4308544011843,-6.13702681123253));
#32747=CARTESIAN_POINT('Ctrl Pts',(-46.1156569468521,49.3931214009566,-6.0717392919641));
#32748=CARTESIAN_POINT('Ctrl Pts',(-47.2226607549441,49.3553884007288,-6.00645177269567));
#32749=CARTESIAN_POINT('Ctrl Pts',(-48.3094287028214,48.7239804681578,-5.94116425342724));
#32750=CARTESIAN_POINT('Ctrl Pts',(-48.8904681014242,47.780966999279,-5.8758767341588));
#32751=CARTESIAN_POINT('Ctrl Pts',(-49.2163719794391,47.2520325633926,-5.83925709052239));
#32752=CARTESIAN_POINT('Ctrl Pts',(-49.3831702945945,46.6250649547388,-5.80263744688598));
#32753=CARTESIAN_POINT('Ctrl Pts',(-49.3849262043165,45.9989672045366,-5.76601780324957));
#32754=CARTESIAN_POINT('Origin',(-46.,46.,-5.));
#32755=CARTESIAN_POINT('',(-49.3946329665444,45.9989154325886,-4.51601780324957));
#32756=CARTESIAN_POINT('',(-49.3926797131717,46.0023448477992,-4.85898219675043));
#32757=CARTESIAN_POINT('',(-49.38975,46.,-5.));
#32758=CARTESIAN_POINT('Ctrl Pts',(-49.3926797131717,46.0023448477992,-4.85898219675043));
#32759=CARTESIAN_POINT('Ctrl Pts',(-49.3939355469422,46.1604461186904,-4.86828355986323));
#32760=CARTESIAN_POINT('Ctrl Pts',(-49.3838127180113,46.3183859042746,-4.87758492297603));
#32761=CARTESIAN_POINT('Ctrl Pts',(-49.3617514440163,46.4746401205548,-4.88688628608883));
#32762=CARTESIAN_POINT('Ctrl Pts',(-49.2069003933082,47.571409489996,-4.95217380535726));
#32763=CARTESIAN_POINT('Ctrl Pts',(-48.4638630471224,48.585133809658,-5.0174613246257));
#32764=CARTESIAN_POINT('Ctrl Pts',(-47.4645770771483,49.0629511924481,-5.08274884389413));
#32765=CARTESIAN_POINT('Ctrl Pts',(-46.4652911071743,49.5407685752381,-5.14803636316256));
#32766=CARTESIAN_POINT('Ctrl Pts',(-45.209756513412,49.4826790211562,-5.21332388243099));
#32767=CARTESIAN_POINT('Ctrl Pts',(-44.2588592935263,48.9146329222825,-5.27861140169942));
#32768=CARTESIAN_POINT('Ctrl Pts',(-43.3079620736407,48.3465868234088,-5.34389892096785));
#32769=CARTESIAN_POINT('Ctrl Pts',(-42.6617022276319,47.2685841797434,-5.40918644023628));
#32770=CARTESIAN_POINT('Ctrl Pts',(-42.6087839206706,46.1622019901345,-5.47447395950472));
#32771=CARTESIAN_POINT('Ctrl Pts',(-42.5558656137093,45.0558198005256,-5.53976147877315));
#32772=CARTESIAN_POINT('Ctrl Pts',(-43.0962888457956,43.9210580649734,-5.60504899804157));
#32773=CARTESIAN_POINT('Ctrl Pts',(-43.9886299492523,43.2648498078038,-5.67033651731001));
#32774=CARTESIAN_POINT('Ctrl Pts',(-44.8809710527091,42.6086415506342,-5.73562403657844));
#32775=CARTESIAN_POINT('Ctrl Pts',(-46.1252300275364,42.4309867718473,-5.80091155584687));
#32776=CARTESIAN_POINT('Ctrl Pts',(-47.1655579679665,42.8112493482335,-5.8661990751153));
#32777=CARTESIAN_POINT('Ctrl Pts',(-48.2058859083967,43.1915119246197,-5.93148659438373));
#32778=CARTESIAN_POINT('Ctrl Pts',(-49.0422828144297,44.1296918561791,-5.99677411365216));
#32779=CARTESIAN_POINT('Ctrl Pts',(-49.3011045901178,45.206675233641,-6.06206163292059));
#32780=CARTESIAN_POINT('Ctrl Pts',(-49.3631075772268,45.4646758840569,-6.07770182086387));
#32781=CARTESIAN_POINT('Ctrl Pts',(-49.3919644910817,45.7306422326894,-6.09334200880715));
#32782=CARTESIAN_POINT('Ctrl Pts',(-49.3896329814502,45.9971074077133,-6.10898219675043));
#32783=CARTESIAN_POINT('Ctrl Pts',(-49.3849262043165,45.9989672045366,-5.76601780324957));
#32784=CARTESIAN_POINT('Ctrl Pts',(-49.3863008272383,45.5088233731412,-5.73734992761755));
#32785=CARTESIAN_POINT('Ctrl Pts',(-49.2865272077179,45.0192126450613,-5.70868205198553));
#32786=CARTESIAN_POINT('Ctrl Pts',(-49.0827569539528,44.5775869410516,-5.68001417635351));
#32787=CARTESIAN_POINT('Ctrl Pts',(-48.6186955585504,43.5718393568893,-5.61472665708508));
#32788=CARTESIAN_POINT('Ctrl Pts',(-47.6152619184171,42.814963193751,-5.54943913781665));
#32789=CARTESIAN_POINT('Ctrl Pts',(-46.520720766888,42.6450783584327,-5.48415161854822));
#32790=CARTESIAN_POINT('Ctrl Pts',(-45.4261796153588,42.4751935231143,-5.41886409927979));
#32791=CARTESIAN_POINT('Ctrl Pts',(-44.2405309524337,42.8923000156159,-5.35357658001136));
#32792=CARTESIAN_POINT('Ctrl Pts',(-43.4934405628386,43.7100635119704,-5.28828906074292));
#32793=CARTESIAN_POINT('Ctrl Pts',(-42.7463501732435,44.5278270083248,-5.22300154147449));
#32794=CARTESIAN_POINT('Ctrl Pts',(-42.4378180569783,45.746247508532,-5.15771402220606));
#32795=CARTESIAN_POINT('Ctrl Pts',(-42.7056750188706,46.8210190350401,-5.09242650293763));
#32796=CARTESIAN_POINT('Ctrl Pts',(-42.9735319807628,47.8957905615482,-5.0271389836692));
#32797=CARTESIAN_POINT('Ctrl Pts',(-43.8177780208124,48.8269131143573,-4.96185146440077));
#32798=CARTESIAN_POINT('Ctrl Pts',(-44.8612624194596,49.1984255593208,-4.89656394513234));
#32799=CARTESIAN_POINT('Ctrl Pts',(-45.9047468181068,49.5699380042843,-4.83127642586391));
#32800=CARTESIAN_POINT('Ctrl Pts',(-47.1474695753515,49.3818403414024,-4.76598890659548));
#32801=CARTESIAN_POINT('Ctrl Pts',(-48.0342681461046,48.7181615927584,-4.70070138732704));
#32802=CARTESIAN_POINT('Ctrl Pts',(-48.8704521530768,48.0923627093522,-4.63914019263455));
#32803=CARTESIAN_POINT('Ctrl Pts',(-49.3901816818208,47.0437216307205,-4.57757899794206));
#32804=CARTESIAN_POINT('Ctrl Pts',(-49.3946329665444,45.9989154325886,-4.51601780324957));
#32805=CARTESIAN_POINT('Origin',(-46.,46.,-5.));
#32806=CARTESIAN_POINT('',(-49.3870900307866,46.0025162764443,-3.26601780324957));
#32807=CARTESIAN_POINT('',(-49.3846596848065,45.9995769998069,-3.60898219675043));
#32808=CARTESIAN_POINT('',(-49.38975,46.,-5.));
#32809=CARTESIAN_POINT('Ctrl Pts',(-49.3846596848065,45.9995769998069,-3.60898219675043));
#32810=CARTESIAN_POINT('Ctrl Pts',(-49.3839903779672,46.5851552579925,-3.64322511091931));
#32811=CARTESIAN_POINT('Ctrl Pts',(-49.2392624490329,47.1710433976494,-3.67746802508819));
#32812=CARTESIAN_POINT('Ctrl Pts',(-48.9524293383723,47.6762508813733,-3.71171093925707));
#32813=CARTESIAN_POINT('Ctrl Pts',(-48.4055535045364,48.6394791616974,-3.7769984585255));
#32814=CARTESIAN_POINT('Ctrl Pts',(-47.3421081071184,49.3094234764506,-3.84228597779394));
#32815=CARTESIAN_POINT('Ctrl Pts',(-46.2371669696481,49.386799056601,-3.90757349706237));
#32816=CARTESIAN_POINT('Ctrl Pts',(-45.1322258321778,49.4641746367513,-3.9728610163308));
#32817=CARTESIAN_POINT('Ctrl Pts',(-43.9857889546551,48.9489814822988,-4.03814853559923));
#32818=CARTESIAN_POINT('Ctrl Pts',(-43.3100050145034,48.0713722499747,-4.10343605486766));
#32819=CARTESIAN_POINT('Ctrl Pts',(-42.6342210743516,47.1937630176505,-4.16872357413609));
#32820=CARTESIAN_POINT('Ctrl Pts',(-42.4290900715707,45.9537377074547,-4.23401109340452));
#32821=CARTESIAN_POINT('Ctrl Pts',(-42.786250344801,44.9052538319623,-4.29929861267295));
#32822=CARTESIAN_POINT('Ctrl Pts',(-43.1434106180313,43.8567699564698,-4.36458613194138));
#32823=CARTESIAN_POINT('Ctrl Pts',(-44.0628621672728,42.9998275156808,-4.42987365120982));
#32824=CARTESIAN_POINT('Ctrl Pts',(-45.1338576566721,42.7172491015831,-4.49516117047825));
#32825=CARTESIAN_POINT('Ctrl Pts',(-46.2048531460714,42.4346706874855,-4.56044868974668));
#32826=CARTESIAN_POINT('Ctrl Pts',(-47.4273925756286,42.7264563000792,-4.62573620901511));
#32827=CARTESIAN_POINT('Ctrl Pts',(-48.2553299127918,43.4622563159863,-4.69102372828354));
#32828=CARTESIAN_POINT('Ctrl Pts',(-48.965312916663,44.0932285914148,-4.74700988443917));
#32829=CARTESIAN_POINT('Ctrl Pts',(-49.3851206807237,45.0507120243974,-4.8029960405948));
#32830=CARTESIAN_POINT('Ctrl Pts',(-49.3926797131717,46.0023448477992,-4.85898219675043));
#32831=CARTESIAN_POINT('Ctrl Pts',(-49.3946329665444,45.9989154325886,-4.51601780324957));
#32832=CARTESIAN_POINT('Ctrl Pts',(-49.3949024046497,45.9356728812925,-4.51229147867363));
#32833=CARTESIAN_POINT('Ctrl Pts',(-49.3932838988388,45.8724443807338,-4.50856515409769));
#32834=CARTESIAN_POINT('Ctrl Pts',(-49.3897333541247,45.8093245590373,-4.50483882952175));
#32835=CARTESIAN_POINT('Ctrl Pts',(-49.3275256071303,44.7034261083662,-4.43955131025332));
#32836=CARTESIAN_POINT('Ctrl Pts',(-48.6722357288803,43.63088904143,-4.37426379098489));
#32837=CARTESIAN_POINT('Ctrl Pts',(-47.7166018986786,43.0708487135956,-4.30897627171646));
#32838=CARTESIAN_POINT('Ctrl Pts',(-46.7609680684769,42.5108083857612,-4.24368875244803));
#32839=CARTESIAN_POINT('Ctrl Pts',(-45.5049902863237,42.4632647970286,-4.1784012331796));
#32840=CARTESIAN_POINT('Ctrl Pts',(-44.5097525254705,42.9494571309534,-4.11311371391116));
#32841=CARTESIAN_POINT('Ctrl Pts',(-43.5145147646174,43.4356494648782,-4.04782619464273));
#32842=CARTESIAN_POINT('Ctrl Pts',(-42.7800170250644,44.4555777214603,-3.9825386753743));
#32843=CARTESIAN_POINT('Ctrl Pts',(-42.6343820787504,45.5536085279835,-3.91725115610587));
#32844=CARTESIAN_POINT('Ctrl Pts',(-42.4887471324365,46.6516393345068,-3.85196363683744));
#32845=CARTESIAN_POINT('Ctrl Pts',(-42.9319749793616,47.8277726909711,-3.78667611756901));
#32846=CARTESIAN_POINT('Ctrl Pts',(-43.7660620822644,48.5565935787908,-3.72138859830058));
#32847=CARTESIAN_POINT('Ctrl Pts',(-44.6001491851673,49.2854144666106,-3.65610107903214));
#32848=CARTESIAN_POINT('Ctrl Pts',(-45.8250955440479,49.5669228857858,-3.59081355976371));
#32849=CARTESIAN_POINT('Ctrl Pts',(-46.8936798813232,49.2753603721713,-3.52552604049528));
#32850=CARTESIAN_POINT('Ctrl Pts',(-47.9622642185986,48.9837978585568,-3.46023852122685));
#32851=CARTESIAN_POINT('Ctrl Pts',(-48.8744865342686,48.1191644121527,-3.39495100195842));
#32852=CARTESIAN_POINT('Ctrl Pts',(-49.222829006556,47.0677183924078,-3.32966348268999));
#32853=CARTESIAN_POINT('Ctrl Pts',(-49.3360231441957,46.7260502498519,-3.30844825620985));
#32854=CARTESIAN_POINT('Ctrl Pts',(-49.3896755337205,46.364656012602,-3.28723302972971));
#32855=CARTESIAN_POINT('Ctrl Pts',(-49.3870900307866,46.0025162764443,-3.26601780324957));
#32856=CARTESIAN_POINT('Origin',(-46.,46.,-5.));
#32857=CARTESIAN_POINT('',(-49.387979831519,45.997252452837,-2.01601780324957));
#32858=CARTESIAN_POINT('',(-49.3939446252011,45.9983056787136,-2.35898219675043));
#32859=CARTESIAN_POINT('',(-49.38975,46.,-5.));
#32860=CARTESIAN_POINT('Ctrl Pts',(-49.3939446252011,45.9983056787136,-2.35898219675043));
#32861=CARTESIAN_POINT('Ctrl Pts',(-49.3877070377124,47.0033169214029,-2.41816666197539));
#32862=CARTESIAN_POINT('Ctrl Pts',(-48.9121877502659,48.0134657894478,-2.47735112720035));
#32863=CARTESIAN_POINT('Ctrl Pts',(-48.130361037692,48.6435236993263,-2.53653559242531));
#32864=CARTESIAN_POINT('Ctrl Pts',(-47.2679129887364,49.3385526697674,-2.60182311169374));
#32865=CARTESIAN_POINT('Ctrl Pts',(-46.0327280276914,49.5710596167832,-2.66711063096217));
#32866=CARTESIAN_POINT('Ctrl Pts',(-44.9766012143833,49.2371763964032,-2.7323981502306));
#32867=CARTESIAN_POINT('Ctrl Pts',(-43.9204744010753,48.9032931760232,-2.79768566949903));
#32868=CARTESIAN_POINT('Ctrl Pts',(-43.0434057355042,48.0030197882473,-2.86297318876747));
#32869=CARTESIAN_POINT('Ctrl Pts',(-42.7372088729773,46.9385361561164,-2.9282607080359));
#32870=CARTESIAN_POINT('Ctrl Pts',(-42.4310120104504,45.8740525239854,-2.99354822730433));
#32871=CARTESIAN_POINT('Ctrl Pts',(-42.6956869509677,44.6453586474994,-3.05883574657276));
#32872=CARTESIAN_POINT('Ctrl Pts',(-43.4129952148832,43.8013499086738,-3.12412326584119));
#32873=CARTESIAN_POINT('Ctrl Pts',(-44.1303034787986,42.9573411698482,-3.18941078510962));
#32874=CARTESIAN_POINT('Ctrl Pts',(-45.3002450661123,42.498017568683,-3.25469830437805));
#32875=CARTESIAN_POINT('Ctrl Pts',(-46.4001710363173,42.6285731250573,-3.31998582364648));
#32876=CARTESIAN_POINT('Ctrl Pts',(-47.5000970065224,42.7591286814316,-3.38527334291492));
#32877=CARTESIAN_POINT('Ctrl Pts',(-48.5300073596189,43.4795633953454,-3.45056086218335));
#32878=CARTESIAN_POINT('Ctrl Pts',(-49.0298094010404,44.4680368752498,-3.51584838145178));
#32879=CARTESIAN_POINT('Ctrl Pts',(-49.2674682549491,44.9380619149337,-3.54689298655133));
#32880=CARTESIAN_POINT('Ctrl Pts',(-49.3852664779787,45.4686921081007,-3.57793759165088));
#32881=CARTESIAN_POINT('Ctrl Pts',(-49.3846596848065,45.9995769998069,-3.60898219675043));
#32882=CARTESIAN_POINT('Ctrl Pts',(-49.3870900307866,46.0025162764443,-3.26601780324957));
#32883=CARTESIAN_POINT('Ctrl Pts',(-49.3817189336448,45.2502109217426,-3.22194551046128));
#32884=CARTESIAN_POINT('Ctrl Pts',(-49.1336505161444,44.4946883307728,-3.17787321767299));
#32885=CARTESIAN_POINT('Ctrl Pts',(-48.6725040913107,43.9061109641452,-3.1338009248847));
#32886=CARTESIAN_POINT('Ctrl Pts',(-47.9893740748734,43.0342081487129,-3.06851340561626));
#32887=CARTESIAN_POINT('Ctrl Pts',(-46.838651413094,42.5286611109342,-3.00322588634783));
#32888=CARTESIAN_POINT('Ctrl Pts',(-45.7343993470158,42.6153131154549,-2.9379383670794));
#32889=CARTESIAN_POINT('Ctrl Pts',(-44.6301472809376,42.7019651199757,-2.87265084781097));
#32890=CARTESIAN_POINT('Ctrl Pts',(-43.5723658105607,43.3808161667959,-2.80736332854254));
#32891=CARTESIAN_POINT('Ctrl Pts',(-43.0335985662276,44.3486029319831,-2.74207580927411));
#32892=CARTESIAN_POINT('Ctrl Pts',(-42.4948313218946,45.3163896971703,-2.67678829000568));
#32893=CARTESIAN_POINT('Ctrl Pts',(-42.4750783036054,46.5731121807244,-2.61150077073725));
#32894=CARTESIAN_POINT('Ctrl Pts',(-42.9831636791679,47.5573530024191,-2.54621325146882));
#32895=CARTESIAN_POINT('Ctrl Pts',(-43.4912490547304,48.5415938241138,-2.48092573220038));
#32896=CARTESIAN_POINT('Ctrl Pts',(-44.5271728241445,49.2533529839491,-2.41563821293195));
#32897=CARTESIAN_POINT('Ctrl Pts',(-45.6281561545019,49.3746672174706,-2.35035069366352));
#32898=CARTESIAN_POINT('Ctrl Pts',(-46.7291394848593,49.4959814509922,-2.28506317439509));
#32899=CARTESIAN_POINT('Ctrl Pts',(-47.89518237616,49.0268507581999,-2.21977565512666));
#32900=CARTESIAN_POINT('Ctrl Pts',(-48.6053770650879,48.1768472445751,-2.15448813585823));
#32901=CARTESIAN_POINT('Ctrl Pts',(-49.1074684086029,47.5759142711215,-2.10833135832201));
#32902=CARTESIAN_POINT('Ctrl Pts',(-49.3817192789863,46.7846147606282,-2.06217458078579));
#32903=CARTESIAN_POINT('Ctrl Pts',(-49.387979831519,45.997252452837,-2.01601780324957));
#32904=CARTESIAN_POINT('Origin',(-46.,46.,-5.));
#32905=CARTESIAN_POINT('',(-49.3940292623548,46.0015451960205,-0.766017803249567));
#32906=CARTESIAN_POINT('',(-49.3881106776293,46.0027671006797,-1.10898219675043));
#32907=CARTESIAN_POINT('',(-49.38975,46.,-5.));
#32908=CARTESIAN_POINT('',(-43.4267655729853,48.2065515280923,0.));
#32909=CARTESIAN_POINT('Ctrl Pts',(-49.3940292623548,46.0015451960205,-0.766017803249567));
#32910=CARTESIAN_POINT('Ctrl Pts',(-49.3879984452729,44.9918196666451,-0.706541093305005));
#32911=CARTESIAN_POINT('Ctrl Pts',(-48.9072367960306,43.9773046953768,-0.647064383360443));
#32912=CARTESIAN_POINT('Ctrl Pts',(-48.1187303416659,43.3473617203725,-0.58758767341588));
#32913=CARTESIAN_POINT('Ctrl Pts',(-47.2531876715922,42.6558740076704,-0.522300154147449));
#32914=CARTESIAN_POINT('Ctrl Pts',(-46.0168300891286,42.4277735844645,-0.457012634879018));
#32915=CARTESIAN_POINT('Ctrl Pts',(-44.962273444483,42.7668602707044,-0.391725115610587));
#32916=CARTESIAN_POINT('Ctrl Pts',(-43.9077167998373,43.1059469569444,-0.326437596342156));
#32917=CARTESIAN_POINT('Ctrl Pts',(-43.0349610930096,44.0122207526302,-0.261150077073725));
#32918=CARTESIAN_POINT('Ctrl Pts',(-42.7336918051393,45.0762567531889,-0.195862557805293));
#32919=CARTESIAN_POINT('Ctrl Pts',(-42.4324225172691,46.1402927537476,-0.130575038536862));
#32920=CARTESIAN_POINT('Ctrl Pts',(-42.7026396483563,47.3620909591791,-0.0652875192684313));
#32921=CARTESIAN_POINT('Ctrl Pts',(-43.4267655729853,48.2065515280923,0.));
#32922=CARTESIAN_POINT('',(-48.5780060810925,48.2094945163745,-2.82133879660966E-15));
#32923=CARTESIAN_POINT('Origin',(-46.,46.,0.));
#32924=CARTESIAN_POINT('Ctrl Pts',(-48.5780352480409,48.2095125055216,-1.80411241501588E-15));
#32925=CARTESIAN_POINT('Ctrl Pts',(-47.8896986135138,49.0067166723596,-0.0620616329205985));
#32926=CARTESIAN_POINT('Ctrl Pts',(-46.7993632977221,49.4635756417559,-0.124123265841195));
#32927=CARTESIAN_POINT('Ctrl Pts',(-45.7491449739559,49.3856448917061,-0.186184898761792));
#32928=CARTESIAN_POINT('Ctrl Pts',(-44.644337610336,49.3036633983736,-0.251472418030223));
#32929=CARTESIAN_POINT('Ctrl Pts',(-43.58392608898,48.6298518891241,-0.316759937298654));
#32930=CARTESIAN_POINT('Ctrl Pts',(-43.0409887593006,47.6645436361188,-0.382047456567084));
#32931=CARTESIAN_POINT('Ctrl Pts',(-42.4980514296212,46.6992353831134,-0.447334975835515));
#32932=CARTESIAN_POINT('Ctrl Pts',(-42.4725882916183,45.4424303863521,-0.512622495103946));
#32933=CARTESIAN_POINT('Ctrl Pts',(-42.9762875061872,44.4559130885416,-0.577910014372377));
#32934=CARTESIAN_POINT('Ctrl Pts',(-43.4799867207561,43.4693957907312,-0.643197533640808));
#32935=CARTESIAN_POINT('Ctrl Pts',(-44.5128482878968,42.7531661918715,-0.708485052909239));
#32936=CARTESIAN_POINT('Ctrl Pts',(-45.6133080412482,42.6270242787203,-0.773772572177669));
#32937=CARTESIAN_POINT('Ctrl Pts',(-46.7137677945997,42.5008823655691,-0.8390600914461));
#32938=CARTESIAN_POINT('Ctrl Pts',(-47.881825734162,42.9648281381265,-0.904347610714531));
#32939=CARTESIAN_POINT('Ctrl Pts',(-48.5957492659174,43.8116818846328,-0.969635129982962));
#32940=CARTESIAN_POINT('Ctrl Pts',(-49.1036725319113,44.414178793072,-1.01608415223878));
#32941=CARTESIAN_POINT('Ctrl Pts',(-49.3817284808321,45.210490631947,-1.06253317449461));
#32942=CARTESIAN_POINT('Ctrl Pts',(-49.3881106776293,46.0027671006797,-1.10898219675043));
#32943=CARTESIAN_POINT('Origin',(-46.,46.,2.76038497140452));
#32944=CARTESIAN_POINT('',(-50.0803097491022,46.0023244644292,-7.76038497140452));
#32945=CARTESIAN_POINT('',(-50.0862705133486,45.9966118456437,-7.86461502859548));
#32946=CARTESIAN_POINT('',(-50.085,46.,2.76038497140452));
#32947=CARTESIAN_POINT('',(-49.4256147683784,43.7746037524369,-9.));
#32948=CARTESIAN_POINT('Ctrl Pts',(-50.0862705133486,45.9966118456437,-7.86461502859549));
#32949=CARTESIAN_POINT('Ctrl Pts',(-50.0769059571497,47.0638214653661,-7.91663908938817));
#32950=CARTESIAN_POINT('Ctrl Pts',(-49.1080148673377,49.4855109457225,-8.03395066944928));
#32951=CARTESIAN_POINT('Ctrl Pts',(-45.0527729214423,50.7128987412233,-8.21654976877883));
#32952=CARTESIAN_POINT('Ctrl Pts',(-41.5512846772643,47.8195936610183,-8.41241232658412));
#32953=CARTESIAN_POINT('Ctrl Pts',(-42.0204412135141,43.2986191788456,-8.60827488438942));
#32954=CARTESIAN_POINT('Ctrl Pts',(-46.0536470456105,41.195226046819,-8.80413744219471));
#32955=CARTESIAN_POINT('Ctrl Pts',(-48.6953045558515,42.6504167892078,-8.93471248073157));
#32956=CARTESIAN_POINT('Ctrl Pts',(-49.4256147683784,43.7746037524369,-9.));
#32957=CARTESIAN_POINT('',(-50.0861552640897,45.7875587543876,-9.));
#32958=CARTESIAN_POINT('Origin',(-46.,46.,-9.));
#32959=CARTESIAN_POINT('Ctrl Pts',(-50.0803097491022,46.0023244644292,-7.76038497140452));
#32960=CARTESIAN_POINT('Ctrl Pts',(-50.0830257350667,46.5110144748489,-7.78509075167359));
#32961=CARTESIAN_POINT('Ctrl Pts',(-49.7610778975337,48.3606597045947,-7.8750840512111));
#32962=CARTESIAN_POINT('Ctrl Pts',(-47.0195850264259,50.6979235414129,-8.03036487001704));
#32963=CARTESIAN_POINT('Ctrl Pts',(-42.6509144693004,49.448562948282,-8.22622742782232));
#32964=CARTESIAN_POINT('Ctrl Pts',(-41.274000700432,45.1181262021708,-8.42208998562762));
#32965=CARTESIAN_POINT('Ctrl Pts',(-44.1206543946181,41.5754411548869,-8.61795254343291));
#32966=CARTESIAN_POINT('Ctrl Pts',(-48.5697422531351,41.9795081408631,-8.81058921489038));
#32967=CARTESIAN_POINT('Ctrl Pts',(-50.0156456694632,44.5202463146725,-8.9379383670794));
#32968=CARTESIAN_POINT('Ctrl Pts',(-50.0861963379778,45.7875630405758,-9.));
#32969=CARTESIAN_POINT('Origin',(-46.,46.,2.76038497140452));
#32970=CARTESIAN_POINT('',(-50.0848589805219,45.9965141265607,-6.51038497140452));
#32971=CARTESIAN_POINT('',(-50.0872033298994,46.003220903795,-6.61461502859548));
#32972=CARTESIAN_POINT('',(-50.085,46.,2.76038497140452));
#32973=CARTESIAN_POINT('Ctrl Pts',(-50.0872033298994,46.003220903795,-6.61461502859548));
#32974=CARTESIAN_POINT('Ctrl Pts',(-50.0892690323773,46.2426360687525,-6.62629312117581));
#32975=CARTESIAN_POINT('Ctrl Pts',(-49.9622030080971,47.8183368728873,-6.70325873302458));
#32976=CARTESIAN_POINT('Ctrl Pts',(-47.9170389384488,50.4085208617021,-6.84551186414178));
#32977=CARTESIAN_POINT('Ctrl Pts',(-43.3883214271118,50.0359894114731,-7.04137442194707));
#32978=CARTESIAN_POINT('Ctrl Pts',(-41.1930659955112,46.0574693216547,-7.23723697975236));
#32979=CARTESIAN_POINT('Ctrl Pts',(-43.2925654154187,42.0275760136403,-7.43309953755766));
#32980=CARTESIAN_POINT('Ctrl Pts',(-47.8111685874939,41.5469454131034,-7.62896209536294));
#32981=CARTESIAN_POINT('Ctrl Pts',(-49.9410013296604,44.1157441623102,-7.77280059237556));
#32982=CARTESIAN_POINT('Ctrl Pts',(-50.0886579933029,45.7245283085182,-7.85135157011974));
#32983=CARTESIAN_POINT('Ctrl Pts',(-50.0862705133486,45.9966118456437,-7.86461502859549));
#32984=CARTESIAN_POINT('Ctrl Pts',(-50.0848589805219,45.9965141265607,-6.51038497140452));
#32985=CARTESIAN_POINT('Ctrl Pts',(-50.0759399931959,47.0158534793692,-6.56003230272967));
#32986=CARTESIAN_POINT('Ctrl Pts',(-49.1785307017076,49.3896732222161,-6.67496715332326));
#32987=CARTESIAN_POINT('Ctrl Pts',(-45.2228146507001,50.7440556643996,-6.85518952318527));
#32988=CARTESIAN_POINT('Ctrl Pts',(-41.6181995750799,47.9773428774946,-7.05105208099057));
#32989=CARTESIAN_POINT('Ctrl Pts',(-41.9285478600743,43.4439512443748,-7.24691463879586));
#32990=CARTESIAN_POINT('Ctrl Pts',(-45.8765970139655,41.1942887704259,-7.44277719660115));
#32991=CARTESIAN_POINT('Ctrl Pts',(-49.4229679546423,42.9805151113374,-7.61393397413737));
#32992=CARTESIAN_POINT('Ctrl Pts',(-50.0758484678822,45.1667497523738,-7.71980323240516));
#32993=CARTESIAN_POINT('Ctrl Pts',(-50.0803097491022,46.0023244644292,-7.76038497140452));
#32994=CARTESIAN_POINT('Origin',(-46.,46.,2.76038497140452));
#32995=CARTESIAN_POINT('',(-50.0885306079523,46.002825784574,-5.26038497140452));
#32996=CARTESIAN_POINT('',(-50.0791868263538,45.9987553744471,-5.36461502859548));
#32997=CARTESIAN_POINT('',(-50.085,46.,2.76038497140452));
#32998=CARTESIAN_POINT('Ctrl Pts',(-50.0791868263538,45.9987553744471,-5.36461502859548));
#32999=CARTESIAN_POINT('Ctrl Pts',(-50.0770707731893,46.7532680404479,-5.40123467223189));
#33000=CARTESIAN_POINT('Ctrl Pts',(-49.5176911419739,48.8558846609211,-5.50314183513674));
#33001=CARTESIAN_POINT('Ctrl Pts',(-46.1637649138928,50.8045026982905,-5.67033651731001));
#33002=CARTESIAN_POINT('Ctrl Pts',(-42.0884430951448,48.7945997915639,-5.86619907511531));
#33003=CARTESIAN_POINT('Ctrl Pts',(-41.507947633761,44.2878293987898,-6.0620616329206));
#33004=CARTESIAN_POINT('Ctrl Pts',(-44.940927797173,41.3108173647246,-6.25792419072589));
#33005=CARTESIAN_POINT('Ctrl Pts',(-49.0590435380633,42.4511112347217,-6.44210865595086));
#33006=CARTESIAN_POINT('Ctrl Pts',(-50.0777205205462,44.9041621623507,-6.56100560190738));
#33007=CARTESIAN_POINT('Ctrl Pts',(-50.0872033298994,46.003220903795,-6.61461502859548));
#33008=CARTESIAN_POINT('Ctrl Pts',(-50.0885306079524,46.002825784574,-5.26038497140452));
#33009=CARTESIAN_POINT('Ctrl Pts',(-50.0900440177768,46.1933541986431,-5.26968633451732));
#33010=CARTESIAN_POINT('Ctrl Pts',(-49.9922181317767,47.7196666123893,-5.34427521689856));
#33011=CARTESIAN_POINT('Ctrl Pts',(-48.0737732836718,50.3369969638681,-5.48415161854822));
#33012=CARTESIAN_POINT('Ctrl Pts',(-43.5346254271756,50.1269851679324,-5.68001417635351));
#33013=CARTESIAN_POINT('Ctrl Pts',(-41.19819518517,46.2296704992633,-5.87587673415881));
#33014=CARTESIAN_POINT('Ctrl Pts',(-43.1519931670912,42.1271540690863,-6.07173929196409));
#33015=CARTESIAN_POINT('Ctrl Pts',(-47.650376155957,41.4848768173615,-6.2676018497694));
#33016=CARTESIAN_POINT('Ctrl Pts',(-49.9077279341632,44.0169308236675,-6.41381707624953));
#33017=CARTESIAN_POINT('Ctrl Pts',(-50.0876686912218,45.6753959792127,-6.49474478346124));
#33018=CARTESIAN_POINT('Ctrl Pts',(-50.0848589805219,45.9965141265607,-6.51038497140452));
#33019=CARTESIAN_POINT('Origin',(-46.,46.,2.76038497140452));
#33020=CARTESIAN_POINT('',(-50.0788656427272,45.9994902409355,-4.01038497140452));
#33021=CARTESIAN_POINT('',(-50.0908844806649,45.9986929838851,-4.11461502859548));
#33022=CARTESIAN_POINT('',(-50.085,46.,2.76038497140452));
#33023=CARTESIAN_POINT('Ctrl Pts',(-50.0908844806649,45.9986929838851,-4.11461502859548));
#33024=CARTESIAN_POINT('Ctrl Pts',(-50.0855202213255,47.2577927167175,-4.17617622328797));
#33025=CARTESIAN_POINT('Ctrl Pts',(-48.7949524579669,49.8617286036896,-4.3030249372489));
#33026=CARTESIAN_POINT('Ctrl Pts',(-44.3876003506517,50.5288223911423,-4.49516117047825));
#33027=CARTESIAN_POINT('Ctrl Pts',(-41.3353884704811,47.1625249105979,-4.69102372828355));
#33028=CARTESIAN_POINT('Ctrl Pts',(-42.4508279821942,42.7575560397258,-4.88688628608884));
#33029=CARTESIAN_POINT('Ctrl Pts',(-46.7373164737192,41.2495864060927,-5.08274884389414));
#33030=CARTESIAN_POINT('Ctrl Pts',(-49.6867797812653,43.4743259227351,-5.24199175806301));
#33031=CARTESIAN_POINT('Ctrl Pts',(-50.0808433894147,45.4080812683183,-5.33594715296346));
#33032=CARTESIAN_POINT('Ctrl Pts',(-50.0791868263538,45.9987553744471,-5.36461502859548));
#33033=CARTESIAN_POINT('Ctrl Pts',(-50.0788656427272,45.9994902409355,-4.01038497140452));
#33034=CARTESIAN_POINT('Ctrl Pts',(-50.0780590586315,46.7051727203774,-4.0446278855734));
#33035=CARTESIAN_POINT('Ctrl Pts',(-49.5711128061907,48.7573944230954,-4.14415831901071));
#33036=CARTESIAN_POINT('Ctrl Pts',(-46.3358174405565,50.7955505353102,-4.30897627171646));
#33037=CARTESIAN_POINT('Ctrl Pts',(-42.1910917427793,48.9329671271487,-4.50483882952175));
#33038=CARTESIAN_POINT('Ctrl Pts',(-41.4494793999576,44.4498901520179,-4.70070138732704));
#33039=CARTESIAN_POINT('Ctrl Pts',(-44.7735825745146,41.351776836325,-4.89656394513234));
#33040=CARTESIAN_POINT('Ctrl Pts',(-48.9835468796149,42.3565763414064,-5.08312513982483));
#33041=CARTESIAN_POINT('Ctrl Pts',(-50.0794211905764,44.8560096230292,-5.20439881524889));
#33042=CARTESIAN_POINT('Ctrl Pts',(-50.0885306079524,46.002825784574,-5.26038497140452));
#33043=CARTESIAN_POINT('Origin',(-46.,46.,2.76038497140452));
#33044=CARTESIAN_POINT('',(-50.0900549580195,45.9979581672823,-2.76038497140452));
#33045=CARTESIAN_POINT('',(-50.0817944614686,46.0030323738549,-2.86461502859548));
#33046=CARTESIAN_POINT('',(-50.085,46.,2.76038497140452));
#33047=CARTESIAN_POINT('Ctrl Pts',(-50.0817944614686,46.0030323738549,-2.86461502859548));
#33048=CARTESIAN_POINT('Ctrl Pts',(-50.0849102604169,46.439448281283,-2.88583025507562));
#33049=CARTESIAN_POINT('Ctrl Pts',(-49.8212797436113,48.2152228624484,-2.97233300082419));
#33050=CARTESIAN_POINT('Ctrl Pts',(-47.2654092996424,50.6377585015902,-3.1241232658412));
#33051=CARTESIAN_POINT('Ctrl Pts',(-42.8368474210137,49.6200180555421,-3.31998582364649));
#33052=CARTESIAN_POINT('Ctrl Pts',(-41.2344409709606,45.3679303548353,-3.51584838145178));
#33053=CARTESIAN_POINT('Ctrl Pts',(-43.8898786280806,41.6805726486878,-3.71171093925708));
#33054=CARTESIAN_POINT('Ctrl Pts',(-48.430628748381,41.8524575015287,-3.90757349706237));
#33055=CARTESIAN_POINT('Ctrl Pts',(-50.0550853181707,44.5112653704681,-4.04187486017517));
#33056=CARTESIAN_POINT('Ctrl Pts',(-50.0912091815013,45.9224791563035,-4.11088870401954));
#33057=CARTESIAN_POINT('Ctrl Pts',(-50.0908844806649,45.9986929838851,-4.11461502859548));
#33058=CARTESIAN_POINT('Ctrl Pts',(-50.0900549580195,45.9979581672823,-2.76038497140452));
#33059=CARTESIAN_POINT('Ctrl Pts',(-50.0825380187493,47.2091008552049,-2.81956943662948));
#33060=CARTESIAN_POINT('Ctrl Pts',(-48.87734553552,49.7692994735359,-2.94404142112287));
#33061=CARTESIAN_POINT('Ctrl Pts',(-44.5509147952652,50.5836918395513,-3.13380092488469));
#33062=CARTESIAN_POINT('Ctrl Pts',(-41.380038920474,47.3289236804855,-3.32966348268999));
#33063=CARTESIAN_POINT('Ctrl Pts',(-42.3369211082577,42.8868133607463,-3.52552604049528));
#33064=CARTESIAN_POINT('Ctrl Pts',(-46.5666236386886,41.2262157555308,-3.72138859830058));
#33065=CARTESIAN_POINT('Ctrl Pts',(-49.6390946438884,43.3754462812598,-3.88300824193699));
#33066=CARTESIAN_POINT('Ctrl Pts',(-50.0795968913763,45.3597189354941,-3.97934036630497));
#33067=CARTESIAN_POINT('Ctrl Pts',(-50.0788656427272,45.9994902409355,-4.01038497140452));
#33068=CARTESIAN_POINT('Origin',(-46.,46.,2.76038497140452));
#33069=CARTESIAN_POINT('',(-50.0830244466748,46.0033346430494,-1.51038497140452));
#33070=CARTESIAN_POINT('',(-50.0828667635534,45.9966889209644,-1.61461502859548));
#33071=CARTESIAN_POINT('',(-50.085,46.,2.76038497140452));
#33072=CARTESIAN_POINT('Ctrl Pts',(-50.0828667635534,45.9966889209644,-1.61461502859548));
#33073=CARTESIAN_POINT('Ctrl Pts',(-50.0753221490254,46.9455420892886,-1.6607718061317));
#33074=CARTESIAN_POINT('Ctrl Pts',(-49.2773370649769,49.24797856107,-1.77221610293635));
#33075=CARTESIAN_POINT('Ctrl Pts',(-45.4734861227781,50.7783710029823,-1.94894791900944));
#33076=CARTESIAN_POINT('Ctrl Pts',(-41.7282996653196,48.2051403801394,-2.14481047681473));
#33077=CARTESIAN_POINT('Ctrl Pts',(-41.7997129669298,43.6616979327745,-2.34067303462002));
#33078=CARTESIAN_POINT('Ctrl Pts',(-45.6239218081334,41.2074403684165,-2.53653559242531));
#33079=CARTESIAN_POINT('Ctrl Pts',(-49.3335197698138,42.8371782046192,-2.71118292375047));
#33080=CARTESIAN_POINT('Ctrl Pts',(-50.0753217328532,45.0964264666476,-2.82054273580719));
#33081=CARTESIAN_POINT('Ctrl Pts',(-50.0817944614686,46.0030323738549,-2.86461502859548));
#33082=CARTESIAN_POINT('Ctrl Pts',(-50.0830244466748,46.0033346430494,-1.51038497140452));
#33083=CARTESIAN_POINT('Ctrl Pts',(-50.0861437977564,46.390566271631,-1.52922346841713));
#33084=CARTESIAN_POINT('Ctrl Pts',(-49.859584554975,48.116232607913,-1.61334948469817));
#33085=CARTESIAN_POINT('Ctrl Pts',(-47.4307681707597,50.5894263088653,-1.76276302024764));
#33086=CARTESIAN_POINT('Ctrl Pts',(-42.968598137007,49.7310442859955,-1.95862557805294));
#33087=CARTESIAN_POINT('Ctrl Pts',(-41.2148485187469,45.539095378305,-2.15448813585823));
#33088=CARTESIAN_POINT('Ctrl Pts',(-43.7364582880855,41.758957824139,-2.35035069366352));
#33089=CARTESIAN_POINT('Ctrl Pts',(-48.2804507290339,41.7680234302945,-2.54621325146882));
#33090=CARTESIAN_POINT('Ctrl Pts',(-50.0295527394747,44.4129094467295,-2.68289134404915));
#33091=CARTESIAN_POINT('Ctrl Pts',(-50.0908300986993,45.8730661157845,-2.75428191736105));
#33092=CARTESIAN_POINT('Ctrl Pts',(-50.0900549580195,45.9979581672823,-2.76038497140452));
#33093=CARTESIAN_POINT('Origin',(-46.,46.,2.76038497140452));
#33094=CARTESIAN_POINT('',(-50.0805800719598,45.9961676961768,-0.260384971404518));
#33095=CARTESIAN_POINT('',(-50.0901569545599,46.0018621213198,-0.364615028595478));
#33096=CARTESIAN_POINT('',(-50.085,46.,2.76038497140452));
#33097=CARTESIAN_POINT('',(-47.057904422973,42.0543614925016,0.));
#33098=CARTESIAN_POINT('Ctrl Pts',(-47.0579044229729,42.0543614925016,5.55111512312578E-16));
#33099=CARTESIAN_POINT('Ctrl Pts',(-48.3527480267224,42.4015349025495,-0.0652875192684306));
#33100=CARTESIAN_POINT('Ctrl Pts',(-49.8153062247254,43.7726401555849,-0.152082509736603));
#33101=CARTESIAN_POINT('Ctrl Pts',(-50.0835487927699,45.5536944557427,-0.238877500204777));
#33102=CARTESIAN_POINT('Ctrl Pts',(-50.0805800719598,45.9961676961768,-0.260384971404518));
#33103=CARTESIAN_POINT('',(-44.9393528874294,42.0481879703258,-3.26985762221281E-15));
#33104=CARTESIAN_POINT('Origin',(-46.,46.,0.));
#33105=CARTESIAN_POINT('Ctrl Pts',(-44.9393361356002,42.0481502636203,8.02309607639273E-17));
#33106=CARTESIAN_POINT('Ctrl Pts',(-46.1664281570359,41.7236247110316,-0.0620616329205977));
#33107=CARTESIAN_POINT('Ctrl Pts',(-48.8989740353372,42.2867115510563,-0.183599975785758));
#33108=CARTESIAN_POINT('Ctrl Pts',(-50.0828891950556,44.7850382294403,-0.305138318650917));
#33109=CARTESIAN_POINT('Ctrl Pts',(-50.0901569545599,46.0018621213198,-0.364615028595479));
#33110=CARTESIAN_POINT('Origin',(46.,46.,-5.));
#33111=CARTESIAN_POINT('',(42.6091954699811,45.9971884981445,-8.26601780324957));
#33112=CARTESIAN_POINT('',(42.6044122534151,45.9998426503687,-8.60898219675043));
#33113=CARTESIAN_POINT('',(42.61025,46.,-5.));
#33114=CARTESIAN_POINT('',(47.303382040875,49.1291532909119,-9.));
#33115=CARTESIAN_POINT('Ctrl Pts',(42.6044122534151,45.9998426503687,-8.60898219675043));
#33116=CARTESIAN_POINT('Ctrl Pts',(42.6053213723518,47.1035783352378,-8.67403394523186));
#33117=CARTESIAN_POINT('Ctrl Pts',(43.1965773203909,48.2078791190907,-8.73908569371329));
#33118=CARTESIAN_POINT('Ctrl Pts',(44.1121203927824,48.8209865441,-8.80413744219471));
#33119=CARTESIAN_POINT('Ctrl Pts',(45.0309817204976,49.4363160895516,-8.86942496146314));
#33120=CARTESIAN_POINT('Ctrl Pts',(46.276485097278,49.5568853032748,-8.93471248073157));
#33121=CARTESIAN_POINT('Ctrl Pts',(47.303382040875,49.1291532909119,-9.));
#33122=CARTESIAN_POINT('',(42.61025,46.,-9.));
#33123=CARTESIAN_POINT('Origin',(46.,46.,-9.));
#33124=CARTESIAN_POINT('',(42.61025,46.,-10.));
#33125=CARTESIAN_POINT('',(42.61025,46.,-5.));
#33126=CARTESIAN_POINT('Origin',(46.,46.,-10.));
#33127=CARTESIAN_POINT('',(48.898001656697,44.2309423651523,-9.));
#33128=CARTESIAN_POINT('Origin',(46.,46.,-9.));
#33129=CARTESIAN_POINT('Ctrl Pts',(48.8980277622168,44.2309202005125,-9.));
#33130=CARTESIAN_POINT('Ctrl Pts',(49.4435068986972,45.1319172328957,-8.9379383670794));
#33131=CARTESIAN_POINT('Ctrl Pts',(49.5410720297735,46.3100640638366,-8.8758767341588));
#33132=CARTESIAN_POINT('Ctrl Pts',(49.1424199628038,47.2847987174335,-8.81381510123821));
#33133=CARTESIAN_POINT('Ctrl Pts',(48.7230464581302,48.3101988637643,-8.74852758196978));
#33134=CARTESIAN_POINT('Ctrl Pts',(47.7545295770243,49.1104910325523,-8.68324006270134));
#33135=CARTESIAN_POINT('Ctrl Pts',(46.6686904456162,49.3285585007771,-8.61795254343291));
#33136=CARTESIAN_POINT('Ctrl Pts',(45.5828513142082,49.5466259690018,-8.55266502416448));
#33137=CARTESIAN_POINT('Ctrl Pts',(44.3796899324978,49.1824687366633,-8.48737750489605));
#33138=CARTESIAN_POINT('Ctrl Pts',(43.5971079012266,48.3985718445634,-8.42208998562762));
#33139=CARTESIAN_POINT('Ctrl Pts',(42.9735109928692,47.7739271953753,-8.37006592483494));
#33140=CARTESIAN_POINT('Ctrl Pts',(42.6169662530301,46.882763549866,-8.31804186404225));
#33141=CARTESIAN_POINT('Ctrl Pts',(42.6091954699811,45.9971884981445,-8.26601780324957));
#33142=CARTESIAN_POINT('Origin',(46.,46.,-5.));
#33143=CARTESIAN_POINT('',(42.6084214217016,46.0026727196953,-7.01601780324957));
#33144=CARTESIAN_POINT('',(42.6141421045691,46.0019288481038,-7.35898219675043));
#33145=CARTESIAN_POINT('',(42.61025,46.,-5.));
#33146=CARTESIAN_POINT('Ctrl Pts',(42.6141421045691,46.0019288481038,-7.35898219675043));
#33147=CARTESIAN_POINT('Ctrl Pts',(42.6118883673488,46.4240419205118,-7.38368797701951));
#33148=CARTESIAN_POINT('Ctrl Pts',(42.6852298192571,46.8454010706231,-7.40839375728858));
#33149=CARTESIAN_POINT('Ctrl Pts',(42.8378015517891,47.2357983442509,-7.43309953755765));
#33150=CARTESIAN_POINT('Ctrl Pts',(43.2409877624255,48.267462563989,-7.49838705682608));
#33151=CARTESIAN_POINT('Ctrl Pts',(44.1974659581544,49.0829094742983,-7.56367457609451));
#33152=CARTESIAN_POINT('Ctrl Pts',(45.2798951927721,49.3178454913476,-7.62896209536294));
#33153=CARTESIAN_POINT('Ctrl Pts',(46.3623244273898,49.5527815083968,-7.69424961463137));
#33154=CARTESIAN_POINT('Ctrl Pts',(47.5707047008963,49.207206632186,-7.75953713389981));
#33155=CARTESIAN_POINT('Ctrl Pts',(48.3653229781552,48.4355168243605,-7.82482465316824));
#33156=CARTESIAN_POINT('Ctrl Pts',(49.1599412554142,47.663827016535,-7.89011217243667));
#33157=CARTESIAN_POINT('Ctrl Pts',(49.5407975364256,46.4660222770948,-7.9553996917051));
#33158=CARTESIAN_POINT('Ctrl Pts',(49.3375314802461,45.3771640957291,-8.02068721097353));
#33159=CARTESIAN_POINT('Ctrl Pts',(49.1342654240667,44.2883059143633,-8.08597473024196));
#33160=CARTESIAN_POINT('Ctrl Pts',(48.3468770306965,43.308394291072,-8.15126224951039));
#33161=CARTESIAN_POINT('Ctrl Pts',(47.3275669774877,42.8752570908402,-8.21654976877882));
#33162=CARTESIAN_POINT('Ctrl Pts',(46.308256924279,42.4421198906085,-8.28183728804726));
#33163=CARTESIAN_POINT('Ctrl Pts',(45.0570252112318,42.5557571134363,-8.34712480731569));
#33164=CARTESIAN_POINT('Ctrl Pts',(44.1319138563052,43.1652562095208,-8.41241232658412));
#33165=CARTESIAN_POINT('Ctrl Pts',(43.2068025013787,43.7747553056054,-8.47769984585255));
#33166=CARTESIAN_POINT('Ctrl Pts',(42.6078115045729,44.8801162749467,-8.54298736512098));
#33167=CARTESIAN_POINT('Ctrl Pts',(42.604425645495,45.9878416982074,-8.60827488438941));
#33168=CARTESIAN_POINT('Ctrl Pts',(42.6044134182475,45.9918419925632,-8.60851065517642));
#33169=CARTESIAN_POINT('Ctrl Pts',(42.6044089584431,45.9958423177544,-8.60874642596342));
#33170=CARTESIAN_POINT('Ctrl Pts',(42.6044122534151,45.9998426503687,-8.60898219675043));
#33171=CARTESIAN_POINT('Ctrl Pts',(42.6091954699811,45.9971884981445,-8.26601780324957));
#33172=CARTESIAN_POINT('Ctrl Pts',(42.6072143201684,45.7714124294044,-8.25275434477382));
#33173=CARTESIAN_POINT('Ctrl Pts',(42.6279030448371,45.545999612327,-8.23949088629807));
#33174=CARTESIAN_POINT('Ctrl Pts',(42.672615883441,45.3254592340216,-8.22622742782233));
#33175=CARTESIAN_POINT('Ctrl Pts',(42.8927085777588,44.2398800674407,-8.1609399085539));
#33176=CARTESIAN_POINT('Ctrl Pts',(43.6948966472266,43.2723582861398,-8.09565238928547));
#33177=CARTESIAN_POINT('Ctrl Pts',(44.7209166654019,42.8550689459674,-8.03036487001703));
#33178=CARTESIAN_POINT('Ctrl Pts',(45.7469366835771,42.437779605795,-7.9650773507486));
#33179=CARTESIAN_POINT('Ctrl Pts',(46.9967886504598,42.570722706751,-7.89978983148017));
#33180=CARTESIAN_POINT('Ctrl Pts',(47.9120768886828,43.1945313366717,-7.83450231221174));
#33181=CARTESIAN_POINT('Ctrl Pts',(48.8273651269058,43.8183399665924,-7.76921479294331));
#33182=CARTESIAN_POINT('Ctrl Pts',(49.4080896364691,44.9330141254778,-7.70392727367488));
#33183=CARTESIAN_POINT('Ctrl Pts',(49.3948465163211,46.0405833329933,-7.63863975440645));
#33184=CARTESIAN_POINT('Ctrl Pts',(49.3816033961731,47.1481525405088,-7.57335223513802));
#33185=CARTESIAN_POINT('Ctrl Pts',(48.7743926463139,48.2486167966545,-7.50806471586959));
#33186=CARTESIAN_POINT('Ctrl Pts',(47.8444624554029,48.8503702861328,-7.44277719660115));
#33187=CARTESIAN_POINT('Ctrl Pts',(46.9145322644919,49.4521237756111,-7.37748967733272));
#33188=CARTESIAN_POINT('Ctrl Pts',(45.6618826325292,49.555166498422,-7.31220215806428));
#33189=CARTESIAN_POINT('Ctrl Pts',(44.6461164034007,49.1134634166091,-7.24691463879585));
#33190=CARTESIAN_POINT('Ctrl Pts',(43.6303501742723,48.6717603347961,-7.18162711952743));
#33191=CARTESIAN_POINT('Ctrl Pts',(42.8514673479782,47.6853114483593,-7.116339600259));
#33192=CARTESIAN_POINT('Ctrl Pts',(42.6574161132917,46.5947951794462,-7.05105208099057));
#33193=CARTESIAN_POINT('Ctrl Pts',(42.62270583008,46.399732630104,-7.03937398841023));
#33194=CARTESIAN_POINT('Ctrl Pts',(42.6067072930659,46.2013404342854,-7.0276958958299));
#33195=CARTESIAN_POINT('Ctrl Pts',(42.6084214217016,46.0026727196953,-7.01601780324957));
#33196=CARTESIAN_POINT('Origin',(46.,46.,-5.));
#33197=CARTESIAN_POINT('',(42.6150735509525,45.9989672044636,-5.76601780324957));
#33198=CARTESIAN_POINT('',(42.6103671367935,45.9971074078126,-6.10898219675043));
#33199=CARTESIAN_POINT('',(42.61025,46.,-5.));
#33200=CARTESIAN_POINT('Ctrl Pts',(42.6103671367935,45.9971074078126,-6.10898219675043));
#33201=CARTESIAN_POINT('Ctrl Pts',(42.6177681492814,46.8429594152923,-6.15862952807558));
#33202=CARTESIAN_POINT('Ctrl Pts',(42.939437978457,47.6938378255849,-6.20827685940074));
#33203=CARTESIAN_POINT('Ctrl Pts',(43.5127589684757,48.3109062447032,-6.25792419072589));
#33204=CARTESIAN_POINT('Ctrl Pts',(44.2666908351797,49.1223671073078,-6.32321170999432));
#33205=CARTESIAN_POINT('Ctrl Pts',(45.4558012251992,49.5295020516264,-6.38849922926275));
#33206=CARTESIAN_POINT('Ctrl Pts',(46.5488771676489,49.3504312396045,-6.45378674853118));
#33207=CARTESIAN_POINT('Ctrl Pts',(47.6419531100986,49.1713604275825,-6.51907426779961));
#33208=CARTESIAN_POINT('Ctrl Pts',(48.6389946049786,48.4060838592201,-6.58436178706805));
#33209=CARTESIAN_POINT('Ctrl Pts',(49.0945939713514,47.3964743899603,-6.64964930633648));
#33210=CARTESIAN_POINT('Ctrl Pts',(49.5501933377243,46.3868649207005,-6.71493682560491));
#33211=CARTESIAN_POINT('Ctrl Pts',(49.46435057559,45.1329225505433,-6.78022434487334));
#33212=CARTESIAN_POINT('Ctrl Pts',(48.8754112762962,44.1948214953291,-6.84551186414177));
#33213=CARTESIAN_POINT('Ctrl Pts',(48.2864719770025,43.2567204401148,-6.9107993834102));
#33214=CARTESIAN_POINT('Ctrl Pts',(47.1944361405491,42.6344606998434,-6.97608690267863));
#33215=CARTESIAN_POINT('Ctrl Pts',(46.0871559866506,42.6060258474755,-7.04137442194706));
#33216=CARTESIAN_POINT('Ctrl Pts',(44.9798758327521,42.5775909951076,-7.1066619412155));
#33217=CARTESIAN_POINT('Ctrl Pts',(43.8573513614085,43.1429810306431,-7.17194946048392));
#33218=CARTESIAN_POINT('Ctrl Pts',(43.2210362385086,44.0496168129944,-7.23723697975236));
#33219=CARTESIAN_POINT('Ctrl Pts',(42.8255123385624,44.6131679648705,-7.27781871875171));
#33220=CARTESIAN_POINT('Ctrl Pts',(42.6178440955465,45.3085654996843,-7.31840045775107));
#33221=CARTESIAN_POINT('Ctrl Pts',(42.6141421045691,46.0019288481038,-7.35898219675043));
#33222=CARTESIAN_POINT('Ctrl Pts',(42.6084214217016,46.0026727196953,-7.01601780324957));
#33223=CARTESIAN_POINT('Ctrl Pts',(42.6162902969306,45.0906691362893,-6.96240837656147));
#33224=CARTESIAN_POINT('Ctrl Pts',(42.9974286013873,44.1728593836379,-6.90879894987337));
#33225=CARTESIAN_POINT('Ctrl Pts',(43.65518491261,43.5447009077758,-6.85518952318527));
#33226=CARTESIAN_POINT('Ctrl Pts',(44.4562245896939,42.7797065564077,-6.78990200391684));
#33227=CARTESIAN_POINT('Ctrl Pts',(45.6675235869406,42.4443015050609,-6.72461448464841));
#33228=CARTESIAN_POINT('Ctrl Pts',(46.7479566577516,42.6883218382704,-6.65932696537998));
#33229=CARTESIAN_POINT('Ctrl Pts',(47.8283897285627,42.9323421714799,-6.59403944611155));
#33230=CARTESIAN_POINT('Ctrl Pts',(48.7779568729381,43.7557878892457,-6.52875192684311));
#33231=CARTESIAN_POINT('Ctrl Pts',(49.1724575142977,44.7908002644018,-6.46346440757468));
#33232=CARTESIAN_POINT('Ctrl Pts',(49.5669581556574,45.8258126395579,-6.39817688830625));
#33233=CARTESIAN_POINT('Ctrl Pts',(49.4063922940013,47.0723916721042,-6.33288936903782));
#33234=CARTESIAN_POINT('Ctrl Pts',(48.7624894883155,47.9736521745216,-6.26760184976939));
#33235=CARTESIAN_POINT('Ctrl Pts',(48.1185866826298,48.874912676939,-6.20231433050096));
#33236=CARTESIAN_POINT('Ctrl Pts',(46.9913469329144,49.4308546492274,-6.13702681123253));
#33237=CARTESIAN_POINT('Ctrl Pts',(45.8843430448095,49.3931216462669,-6.0717392919641));
#33238=CARTESIAN_POINT('Ctrl Pts',(44.7773391567047,49.3553886433064,-6.00645177269566));
#33239=CARTESIAN_POINT('Ctrl Pts',(43.6905711302104,48.723980665097,-5.94116425342724));
#33240=CARTESIAN_POINT('Ctrl Pts',(43.1095316895885,47.7809671280428,-5.87587673415881));
#33241=CARTESIAN_POINT('Ctrl Pts',(42.7836277880051,47.2520326539168,-5.83925709052239));
#33242=CARTESIAN_POINT('Ctrl Pts',(42.6168294607952,46.6250649999332,-5.80263744688598));
#33243=CARTESIAN_POINT('Ctrl Pts',(42.6150735509525,45.9989672044636,-5.76601780324957));
#33244=CARTESIAN_POINT('Origin',(46.,46.,-5.));
#33245=CARTESIAN_POINT('',(42.6053667880302,45.9989154325097,-4.51601780324956));
#33246=CARTESIAN_POINT('',(42.6073204051797,46.0023448477177,-4.85898219675043));
#33247=CARTESIAN_POINT('',(42.61025,46.,-5.));
#33248=CARTESIAN_POINT('Ctrl Pts',(42.6073204051797,46.0023448477177,-4.85898219675043));
#33249=CARTESIAN_POINT('Ctrl Pts',(42.6060645714529,46.1604461130937,-4.86828355986323));
#33250=CARTESIAN_POINT('Ctrl Pts',(42.6161874000306,46.3183858931683,-4.87758492297603));
#33251=CARTESIAN_POINT('Ctrl Pts',(42.638248673256,46.4746401039977,-4.88688628608884));
#33252=CARTESIAN_POINT('Ctrl Pts',(42.7930997185616,47.5714094351789,-4.95217380535727));
#33253=CARTESIAN_POINT('Ctrl Pts',(43.5361370388243,48.585133719477,-5.0174613246257));
#33254=CARTESIAN_POINT('Ctrl Pts',(44.5354229739406,49.0629510855994,-5.08274884389413));
#33255=CARTESIAN_POINT('Ctrl Pts',(45.5347089090568,49.5407684517217,-5.14803636316256));
#33256=CARTESIAN_POINT('Ctrl Pts',(46.7902434590266,49.4826788996682,-5.21332388243099));
#33257=CARTESIAN_POINT('Ctrl Pts',(47.7411406457384,48.9146328206093,-5.27861140169942));
#33258=CARTESIAN_POINT('Ctrl Pts',(48.6920378324503,48.3465867415504,-5.34389892096786));
#33259=CARTESIAN_POINT('Ctrl Pts',(49.3382976559041,47.268584135486,-5.40918644023628));
#33260=CARTESIAN_POINT('Ctrl Pts',(49.3912159610244,46.1622019844742,-5.47447395950471));
#33261=CARTESIAN_POINT('Ctrl Pts',(49.4441342661448,45.0558198334624,-5.53976147877314));
#33262=CARTESIAN_POINT('Ctrl Pts',(48.9037110529317,43.9210581375031,-5.60504899804158));
#33263=CARTESIAN_POINT('Ctrl Pts',(48.0113699805936,43.2648499032208,-5.67033651731001));
#33264=CARTESIAN_POINT('Ctrl Pts',(47.1190289082556,42.6086416689385,-5.73562403657844));
#33265=CARTESIAN_POINT('Ctrl Pts',(45.8747699767926,42.4309868963332,-5.80091155584687));
#33266=CARTESIAN_POINT('Ctrl Pts',(44.834442072672,42.8112494594622,-5.8661990751153));
#33267=CARTESIAN_POINT('Ctrl Pts',(43.7941141685514,43.1915120225911,-5.93148659438373));
#33268=CARTESIAN_POINT('Ctrl Pts',(42.9577172917731,44.1296919214543,-5.99677411365216));
#33269=CARTESIAN_POINT('Ctrl Pts',(42.6988955250782,45.2066752613311,-6.06206163292059));
#33270=CARTESIAN_POINT('Ctrl Pts',(42.6368925401237,45.4646759027431,-6.07770182086387));
#33271=CARTESIAN_POINT('Ctrl Pts',(42.6080356272603,45.7306422420912,-6.09334200880715));
#33272=CARTESIAN_POINT('Ctrl Pts',(42.6103671367935,45.9971074078126,-6.10898219675043));
#33273=CARTESIAN_POINT('Ctrl Pts',(42.6150735509525,45.9989672044636,-5.76601780324957));
#33274=CARTESIAN_POINT('Ctrl Pts',(42.6136989279362,45.5088233376305,-5.73734992761755));
#33275=CARTESIAN_POINT('Ctrl Pts',(42.713472554676,45.0192125741512,-5.70868205198553));
#33276=CARTESIAN_POINT('Ctrl Pts',(42.9172428231758,44.5775868382122,-5.68001417635351));
#33277=CARTESIAN_POINT('Ctrl Pts',(43.3813042521348,43.5718391813348,-5.61472665708508));
#33278=CARTESIAN_POINT('Ctrl Pts',(44.3847379648023,42.814962963479,-5.54943913781665));
#33279=CARTESIAN_POINT('Ctrl Pts',(45.4792791954617,42.6450781158791,-5.48415161854822));
#33280=CARTESIAN_POINT('Ctrl Pts',(46.5738204261212,42.4751932682792,-5.41886409927979));
#33281=CARTESIAN_POINT('Ctrl Pts',(47.7594691747726,42.8922997909351,-5.35357658001136));
#33282=CARTESIAN_POINT('Ctrl Pts',(48.5065596183824,43.7100633464118,-5.28828906074292));
#33283=CARTESIAN_POINT('Ctrl Pts',(49.2536500619923,44.5278269018886,-5.22300154147449));
#33284=CARTESIAN_POINT('Ctrl Pts',(49.5621822005606,45.7462474901862,-5.15771402220606));
#33285=CARTESIAN_POINT('Ctrl Pts',(49.294325219302,46.8210190943985,-5.09242650293763));
#33286=CARTESIAN_POINT('Ctrl Pts',(49.0264682380435,47.8957906986107,-5.0271389836692));
#33287=CARTESIAN_POINT('Ctrl Pts',(48.1822221369581,48.8269133187375,-4.96185146440077));
#33288=CARTESIAN_POINT('Ctrl Pts',(47.1387376628694,49.1984257905606,-4.89656394513234));
#33289=CARTESIAN_POINT('Ctrl Pts',(46.0952531887807,49.5699382623838,-4.83127642586391));
#33290=CARTESIAN_POINT('Ctrl Pts',(44.8525303416886,49.3818405859034,-4.76598890659547));
#33291=CARTESIAN_POINT('Ctrl Pts',(43.9657317068215,48.7181617892766,-4.70070138732704));
#33292=CARTESIAN_POINT('Ctrl Pts',(43.1295476393945,48.0923628606262,-4.63914019263455));
#33293=CARTESIAN_POINT('Ctrl Pts',(42.6098180730754,47.0437217061788,-4.57757899794206));
#33294=CARTESIAN_POINT('Ctrl Pts',(42.6053667880302,45.9989154325097,-4.51601780324956));
#33295=CARTESIAN_POINT('Origin',(46.,46.,-5.));
#33296=CARTESIAN_POINT('',(42.6129097243346,46.0025162766385,-3.26601780324956));
#33297=CARTESIAN_POINT('',(42.6153404332635,45.9995769998228,-3.60898219675043));
#33298=CARTESIAN_POINT('',(42.61025,46.,-5.));
#33299=CARTESIAN_POINT('Ctrl Pts',(42.6153404332635,45.9995769998228,-3.60898219675043));
#33300=CARTESIAN_POINT('Ctrl Pts',(42.6160097400798,46.5851552375805,-3.64322511091931));
#33301=CARTESIAN_POINT('Ctrl Pts',(42.760737663966,47.1710433567983,-3.67746802508819));
#33302=CARTESIAN_POINT('Ctrl Pts',(43.0475707646209,47.6762508228982,-3.71171093925708));
#33303=CARTESIAN_POINT('Ctrl Pts',(43.5944465793799,48.6394790696203,-3.77699845852551));
#33304=CARTESIAN_POINT('Ctrl Pts',(44.6578919396997,49.3094233610044,-3.84228597779394));
#33305=CARTESIAN_POINT('Ctrl Pts',(45.762833038625,49.3867989384559,-3.90757349706237));
#33306=CARTESIAN_POINT('Ctrl Pts',(46.8677741375502,49.4641745159074,-3.9728610163308));
#33307=CARTESIAN_POINT('Ctrl Pts',(48.0142109750811,48.9489813794264,-4.03814853559923));
#33308=CARTESIAN_POINT('Ctrl Pts',(48.6899948916588,48.0713721777166,-4.10343605486766));
#33309=CARTESIAN_POINT('Ctrl Pts',(49.3657788082366,47.1937629760069,-4.16872357413609));
#33310=CARTESIAN_POINT('Ctrl Pts',(49.5709098038613,45.9537377090685,-4.23401109340452));
#33311=CARTESIAN_POINT('Ctrl Pts',(49.2137495430902,44.9052538701515,-4.29929861267296));
#33312=CARTESIAN_POINT('Ctrl Pts',(48.8565892823191,43.8567700312346,-4.36458613194139));
#33313=CARTESIAN_POINT('Ctrl Pts',(47.9371377651523,42.9998276203391,-4.42987365120982));
#33314=CARTESIAN_POINT('Ctrl Pts',(46.8661423131135,42.7172492160988,-4.49516117047825));
#33315=CARTESIAN_POINT('Ctrl Pts',(45.7951468610747,42.4346708118586,-4.56044868974668));
#33316=CARTESIAN_POINT('Ctrl Pts',(44.5726074741639,42.7264564142735,-4.62573620901511));
#33317=CARTESIAN_POINT('Ctrl Pts',(43.7446701658828,43.462256404513,-4.69102372828354));
#33318=CARTESIAN_POINT('Ctrl Pts',(43.034687186779,44.0932286579308,-4.74700988443917));
#33319=CARTESIAN_POINT('Ctrl Pts',(42.6148794373641,45.0507120575128,-4.8029960405948));
#33320=CARTESIAN_POINT('Ctrl Pts',(42.6073204051797,46.0023448477177,-4.85898219675043));
#33321=CARTESIAN_POINT('Ctrl Pts',(42.6053667880302,45.9989154325097,-4.51601780324956));
#33322=CARTESIAN_POINT('Ctrl Pts',(42.6050973499054,45.9356728766413,-4.51229147867363));
#33323=CARTESIAN_POINT('Ctrl Pts',(42.6067158558333,45.8724443715113,-4.50856515409769));
#33324=CARTESIAN_POINT('Ctrl Pts',(42.6102664008042,45.8093245452514,-4.50483882952175));
#33325=CARTESIAN_POINT('Ctrl Pts',(42.6724741522961,44.7034260146263,-4.43955131025332));
#33326=CARTESIAN_POINT('Ctrl Pts',(43.3277640779222,43.6308888701494,-4.37426379098489));
#33327=CARTESIAN_POINT('Ctrl Pts',(44.2833979772143,43.0708485018244,-4.30897627171646));
#33328=CARTESIAN_POINT('Ctrl Pts',(45.2390318765064,42.5108081334994,-4.24368875244803));
#33329=CARTESIAN_POINT('Ctrl Pts',(46.4950097494645,42.4632645413262,-4.17840123317959));
#33330=CARTESIAN_POINT('Ctrl Pts',(47.4902475822715,42.9494569104033,-4.11311371391116));
#33331=CARTESIAN_POINT('Ctrl Pts',(48.4854854150785,43.4356492794804,-4.04782619464273));
#33332=CARTESIAN_POINT('Ctrl Pts',(49.2199832077344,44.4555776098078,-3.9825386753743));
#33333=CARTESIAN_POINT('Ctrl Pts',(49.3656181645774,45.5536084957135,-3.91725115610587));
#33334=CARTESIAN_POINT('Ctrl Pts',(49.5112531214204,46.6516393816192,-3.85196363683744));
#33335=CARTESIAN_POINT('Ctrl Pts',(49.0680252424504,47.8277728231033,-3.78667611756901));
#33336=CARTESIAN_POINT('Ctrl Pts',(48.2339380792449,48.5565937636213,-3.72138859830058));
#33337=CARTESIAN_POINT('Ctrl Pts',(47.3998509160394,49.2854147041394,-3.65610107903214));
#33338=CARTESIAN_POINT('Ctrl Pts',(46.1749044685984,49.5669231436913,-3.59081355976371));
#33339=CARTESIAN_POINT('Ctrl Pts',(45.1063200540658,49.275360608986,-3.52552604049528));
#33340=CARTESIAN_POINT('Ctrl Pts',(44.0377356395332,48.9837980742807,-3.46023852122685));
#33341=CARTESIAN_POINT('Ctrl Pts',(43.125513257909,48.1191645653182,-3.39495100195842));
#33342=CARTESIAN_POINT('Ctrl Pts',(42.7771707604387,47.0677184695778,-3.32966348268999));
#33343=CARTESIAN_POINT('Ctrl Pts',(42.6639766146157,46.726050302327,-3.30844825620985));
#33344=CARTESIAN_POINT('Ctrl Pts',(42.6103242212129,46.3646560389635,-3.28723302972971));
#33345=CARTESIAN_POINT('Ctrl Pts',(42.6129097243346,46.0025162766385,-3.26601780324956));
#33346=CARTESIAN_POINT('Origin',(46.,46.,-5.));
#33347=CARTESIAN_POINT('',(42.612019924001,45.9972524552388,-2.01601780324957));
#33348=CARTESIAN_POINT('',(42.6060554931448,45.9983056788579,-2.35898219675043));
#33349=CARTESIAN_POINT('',(42.61025,46.,-5.));
#33350=CARTESIAN_POINT('Ctrl Pts',(42.6060554931448,45.9983056788579,-2.35898219675043));
#33351=CARTESIAN_POINT('Ctrl Pts',(42.6122930804025,47.0033168865153,-2.41816666197539));
#33352=CARTESIAN_POINT('Ctrl Pts',(43.0878123513283,48.0134657192039,-2.47735112720035));
#33353=CARTESIAN_POINT('Ctrl Pts',(43.8696390366459,48.6435236070725,-2.53653559242531));
#33354=CARTESIAN_POINT('Ctrl Pts',(44.7320870555345,49.3385525532341,-2.60182311169375));
#33355=CARTESIAN_POINT('Ctrl Pts',(45.9672719734487,49.5710594922115,-2.66711063096218));
#33356=CARTESIAN_POINT('Ctrl Pts',(47.0233987499047,49.2371762834963,-2.73239815023061));
#33357=CARTESIAN_POINT('Ctrl Pts',(48.0795255263607,48.903293074781,-2.79768566949904));
#33358=CARTESIAN_POINT('Ctrl Pts',(48.9565941613586,48.0030197183732,-2.86297318876747));
#33359=CARTESIAN_POINT('Ctrl Pts',(49.2627910132094,46.9385361233667,-2.9282607080359));
#33360=CARTESIAN_POINT('Ctrl Pts',(49.5689878650602,45.8740525283602,-2.99354822730433));
#33361=CARTESIAN_POINT('Ctrl Pts',(49.304312933764,44.6453586947551,-3.05883574657276));
#33362=CARTESIAN_POINT('Ctrl Pts',(48.5870046948683,43.8013499853766,-3.12412326584119));
#33363=CARTESIAN_POINT('Ctrl Pts',(47.8696964559727,42.9573412759981,-3.18941078510963));
#33364=CARTESIAN_POINT('Ctrl Pts',(46.6997549094776,42.4980176908463,-3.25469830437806));
#33365=CARTESIAN_POINT('Ctrl Pts',(45.5998289776439,42.6285732426639,-3.31998582364649));
#33366=CARTESIAN_POINT('Ctrl Pts',(44.4999030458102,42.7591287944815,-3.38527334291492));
#33367=CARTESIAN_POINT('Ctrl Pts',(43.4699927286378,43.4795634832685,-3.45056086218335));
#33368=CARTESIAN_POINT('Ctrl Pts',(42.9701907046508,44.4680369286922,-3.51584838145178));
#33369=CARTESIAN_POINT('Ctrl Pts',(42.7325318590322,44.9380619519803,-3.54689298655133));
#33370=CARTESIAN_POINT('Ctrl Pts',(42.6147336401121,45.4686921266364,-3.57793759165088));
#33371=CARTESIAN_POINT('Ctrl Pts',(42.6153404332635,45.9995769998228,-3.60898219675043));
#33372=CARTESIAN_POINT('Ctrl Pts',(42.6129097243346,46.0025162766385,-3.26601780324956));
#33373=CARTESIAN_POINT('Ctrl Pts',(42.6182808218664,45.2502108675773,-3.22194551046127));
#33374=CARTESIAN_POINT('Ctrl Pts',(42.8663492573033,44.4946882220169,-3.17787321767299));
#33375=CARTESIAN_POINT('Ctrl Pts',(43.3274957154746,43.9061108128077,-3.1338009248847));
#33376=CARTESIAN_POINT('Ctrl Pts',(44.0106257812974,43.0342079342963,-3.06851340561626));
#33377=CARTESIAN_POINT('Ctrl Pts',(45.1613485262596,42.5286608597917,-3.00322588634783));
#33378=CARTESIAN_POINT('Ctrl Pts',(46.2656006721812,42.6153128706582,-2.9379383670794));
#33379=CARTESIAN_POINT('Ctrl Pts',(47.3698528181026,42.7019648815247,-2.87265084781097));
#33380=CARTESIAN_POINT('Ctrl Pts',(48.4276343649834,43.3808159777622,-2.80736332854254));
#33381=CARTESIAN_POINT('Ctrl Pts',(48.9664016482502,44.3486028127642,-2.74207580927411));
#33382=CARTESIAN_POINT('Ctrl Pts',(49.505168931517,45.3163896477662,-2.67678829000568));
#33383=CARTESIAN_POINT('Ctrl Pts',(49.5249219511698,46.5731122215327,-2.61150077073725));
#33384=CARTESIAN_POINT('Ctrl Pts',(49.0168365389143,47.5573531146787,-2.54621325146882));
#33385=CARTESIAN_POINT('Ctrl Pts',(48.5087511266589,48.5415940078247,-2.48092573220038));
#33386=CARTESIAN_POINT('Ctrl Pts',(47.4728272824952,49.2533532203503,-2.41563821293195));
#33387=CARTESIAN_POINT('Ctrl Pts',(46.3718438724484,49.3746674620912,-2.35035069366352));
#33388=CARTESIAN_POINT('Ctrl Pts',(45.2708604624016,49.4959817038321,-2.28506317439509));
#33389=CARTESIAN_POINT('Ctrl Pts',(44.1048174864718,49.0268509747885,-2.21977565512666));
#33390=CARTESIAN_POINT('Ctrl Pts',(43.3946227463979,48.1768474007417,-2.15448813585823));
#33391=CARTESIAN_POINT('Ctrl Pts',(42.8925313667238,47.5759143845713,-2.10833135832201));
#33392=CARTESIAN_POINT('Ctrl Pts',(42.6182804769167,46.7846148192803,-2.06217458078579));
#33393=CARTESIAN_POINT('Ctrl Pts',(42.612019924001,45.9972524552388,-2.01601780324957));
#33394=CARTESIAN_POINT('Origin',(46.,46.,-5.));
#33395=CARTESIAN_POINT('',(42.6059705137377,46.0015452631454,-0.766017803249565));
#33396=CARTESIAN_POINT('',(42.6118894404877,46.0027670997301,-1.10898219675043));
#33397=CARTESIAN_POINT('',(42.61025,46.,-5.));
#33398=CARTESIAN_POINT('',(48.5732344270147,48.2065515280923,2.77555756156289E-16));
#33399=CARTESIAN_POINT('Ctrl Pts',(42.6059705137377,46.0015452631454,-0.766017803249565));
#33400=CARTESIAN_POINT('Ctrl Pts',(42.612001272004,44.9918195798286,-0.706541093305003));
#33401=CARTESIAN_POINT('Ctrl Pts',(43.0927628221167,43.977304319078,-0.647064383360442));
#33402=CARTESIAN_POINT('Ctrl Pts',(43.8812694180946,43.3473613724735,-0.58758767341588));
#33403=CARTESIAN_POINT('Ctrl Pts',(44.746812243617,42.6558736909459,-0.522300154147449));
#33404=CARTESIAN_POINT('Ctrl Pts',(45.9831702716104,42.4277736819444,-0.457012634879018));
#33405=CARTESIAN_POINT('Ctrl Pts',(47.0377266680876,42.7668601274187,-0.391725115610586));
#33406=CARTESIAN_POINT('Ctrl Pts',(48.0922830645648,43.105946572893,-0.326437596342155));
#33407=CARTESIAN_POINT('Ctrl Pts',(48.9650378295259,44.0122194728431,-0.261150077073724));
#33408=CARTESIAN_POINT('Ctrl Pts',(49.2663071512956,45.0762555694146,-0.195862557805293));
#33409=CARTESIAN_POINT('Ctrl Pts',(49.5675764730653,46.1402916659861,-0.130575038536862));
#33410=CARTESIAN_POINT('Ctrl Pts',(49.2973603516437,47.3620909591791,-0.0652875192684305));
#33411=CARTESIAN_POINT('Ctrl Pts',(48.5732344270147,48.2065515280923,6.43618311088306E-16));
#33412=CARTESIAN_POINT('',(43.4219940034589,48.2094945108994,-4.30182186788769E-15));
#33413=CARTESIAN_POINT('Origin',(46.,46.,0.));
#33414=CARTESIAN_POINT('Ctrl Pts',(43.4219648396841,48.2095124983745,-2.91433543964104E-15));
#33415=CARTESIAN_POINT('Ctrl Pts',(44.1103014967847,49.006716779805,-0.0620616329205997));
#33416=CARTESIAN_POINT('Ctrl Pts',(45.2006367519963,49.463575489776,-0.124123265841196));
#33417=CARTESIAN_POINT('Ctrl Pts',(46.2508550251211,49.3856446881349,-0.186184898761793));
#33418=CARTESIAN_POINT('Ctrl Pts',(47.3556623354671,49.3036631405295,-0.251472418030224));
#33419=CARTESIAN_POINT('Ctrl Pts',(48.4160738145477,48.6298518070086,-0.316759937298655));
#33420=CARTESIAN_POINT('Ctrl Pts',(48.9590111284627,47.664543622046,-0.382047456567087));
#33421=CARTESIAN_POINT('Ctrl Pts',(49.5019484423776,46.6992354370834,-0.447334975835518));
#33422=CARTESIAN_POINT('Ctrl Pts',(49.527411591127,45.442430400679,-0.512622495103949));
#33423=CARTESIAN_POINT('Ctrl Pts',(49.0237123948945,44.4559131182979,-0.57791001437238));
#33424=CARTESIAN_POINT('Ctrl Pts',(48.520013198662,43.4693958359168,-0.643197533640811));
#33425=CARTESIAN_POINT('Ctrl Pts',(47.4871516574478,42.7531663075589,-0.708485052909242));
#33426=CARTESIAN_POINT('Ctrl Pts',(46.3866919409849,42.6270244092924,-0.773772572177674));
#33427=CARTESIAN_POINT('Ctrl Pts',(45.2862322245221,42.5008825110258,-0.839060091446105));
#33428=CARTESIAN_POINT('Ctrl Pts',(44.1181743328107,42.9648282428506,-0.904347610714536));
#33429=CARTESIAN_POINT('Ctrl Pts',(43.4042508272458,43.811681954104,-0.969635129982967));
#33430=CARTESIAN_POINT('Ctrl Pts',(42.8963275798851,44.4141788374625,-1.01608415223879));
#33431=CARTESIAN_POINT('Ctrl Pts',(42.6182716386338,45.2104906540304,-1.06253317449461));
#33432=CARTESIAN_POINT('Ctrl Pts',(42.6118894404877,46.0027670997301,-1.10898219675043));
#33433=CARTESIAN_POINT('Origin',(46.,46.,2.76038497140452));
#33434=CARTESIAN_POINT('',(41.9196903893103,46.0023244618346,-7.76038497140452));
#33435=CARTESIAN_POINT('',(41.9137291820556,45.9966118489329,-7.86461502859548));
#33436=CARTESIAN_POINT('',(41.915,46.0000000000001,2.76038497140452));
#33437=CARTESIAN_POINT('',(42.5743852316216,43.7746037524369,-9.));
#33438=CARTESIAN_POINT('Ctrl Pts',(41.9137291820556,45.9966118489329,-7.86461502859548));
#33439=CARTESIAN_POINT('Ctrl Pts',(41.9230937808476,47.0638215506166,-7.91663908938816));
#33440=CARTESIAN_POINT('Ctrl Pts',(42.8919850912141,49.4855112174958,-8.03395066944928));
#33441=CARTESIAN_POINT('Ctrl Pts',(46.9472267461691,50.7128989977065,-8.21654976877883));
#33442=CARTESIAN_POINT('Ctrl Pts',(50.4487163480431,47.8195940258066,-8.41241232658412));
#33443=CARTESIAN_POINT('Ctrl Pts',(49.9795579209025,43.2986184205048,-8.6082748843894));
#33444=CARTESIAN_POINT('Ctrl Pts',(45.9463561559116,41.1952276423334,-8.80413744219472));
#33445=CARTESIAN_POINT('Ctrl Pts',(43.3046954441484,42.6504167892078,-8.93471248073157));
#33446=CARTESIAN_POINT('Ctrl Pts',(42.5743852316216,43.7746037524369,-9.));
#33447=CARTESIAN_POINT('',(41.9138448206429,45.7875586974126,-9.));
#33448=CARTESIAN_POINT('Origin',(46.,46.,-9.));
#33449=CARTESIAN_POINT('Ctrl Pts',(41.9196903893103,46.0023244618346,-7.76038497140452));
#33450=CARTESIAN_POINT('Ctrl Pts',(41.9169744024249,46.5110144539541,-7.78509075167359));
#33451=CARTESIAN_POINT('Ctrl Pts',(42.2389222273681,48.3606596187085,-7.8750840512111));
#33452=CARTESIAN_POINT('Ctrl Pts',(44.9804150360981,50.6979233958617,-8.03036487001703));
#33453=CARTESIAN_POINT('Ctrl Pts',(49.3490853663058,49.448562791698,-8.22622742782233));
#33454=CARTESIAN_POINT('Ctrl Pts',(50.7259992165293,45.1181263046889,-8.42208998562762));
#33455=CARTESIAN_POINT('Ctrl Pts',(47.8793454040792,41.5754411676036,-8.61795254343291));
#33456=CARTESIAN_POINT('Ctrl Pts',(43.4302580460658,41.9795085567297,-8.81058921489037));
#33457=CARTESIAN_POINT('Ctrl Pts',(41.9843543567741,44.5202461309732,-8.9379383670794));
#33458=CARTESIAN_POINT('Ctrl Pts',(41.913803751014,45.7875629828622,-9.));
#33459=CARTESIAN_POINT('Origin',(46.,46.,2.76038497140452));
#33460=CARTESIAN_POINT('',(41.915141161974,45.9965141266804,-6.51038497140452));
#33461=CARTESIAN_POINT('',(41.9127963736709,46.0032209041833,-6.61461502859548));
#33462=CARTESIAN_POINT('',(41.915,46.0000000000001,2.76038497140452));
#33463=CARTESIAN_POINT('Ctrl Pts',(41.9127963736709,46.0032209041833,-6.61461502859548));
#33464=CARTESIAN_POINT('Ctrl Pts',(41.9107306710448,46.2426360864535,-6.62629312117581));
#33465=CARTESIAN_POINT('Ctrl Pts',(42.0377967048478,47.818337004481,-6.70325873302458));
#33466=CARTESIAN_POINT('Ctrl Pts',(44.0829609284797,50.4085211796553,-6.84551186414177));
#33467=CARTESIAN_POINT('Ctrl Pts',(48.6116787512404,50.0359897044587,-7.04137442194707));
#33468=CARTESIAN_POINT('Ctrl Pts',(50.8069343717212,46.0574693241754,-7.23723697975236));
#33469=CARTESIAN_POINT('Ctrl Pts',(48.7074347435192,42.027575728146,-7.43309953755765));
#33470=CARTESIAN_POINT('Ctrl Pts',(44.1888313497151,41.5469450910147,-7.62896209536295));
#33471=CARTESIAN_POINT('Ctrl Pts',(42.0589983118285,44.1157440212414,-7.77280059237555));
#33472=CARTESIAN_POINT('Ctrl Pts',(41.9113416912421,45.7245282909115,-7.85135157011973));
#33473=CARTESIAN_POINT('Ctrl Pts',(41.9137291820556,45.9966118489329,-7.86461502859548));
#33474=CARTESIAN_POINT('Ctrl Pts',(41.915141161974,45.9965141266804,-6.51038497140452));
#33475=CARTESIAN_POINT('Ctrl Pts',(41.9240601489239,47.0158534439028,-6.56003230272967));
#33476=CARTESIAN_POINT('Ctrl Pts',(42.8214694089007,49.3896731038562,-6.67496715332326));
#33477=CARTESIAN_POINT('Ctrl Pts',(46.7771853228611,50.7440554992066,-6.85518952318527));
#33478=CARTESIAN_POINT('Ctrl Pts',(50.3818002707934,47.9773428079219,-7.05105208099057));
#33479=CARTESIAN_POINT('Ctrl Pts',(50.0714520002853,43.4439513347231,-7.24691463879585));
#33480=CARTESIAN_POINT('Ctrl Pts',(46.1234029772789,41.1942889357184,-7.44277719660116));
#33481=CARTESIAN_POINT('Ctrl Pts',(42.577032171383,42.9805152204495,-7.61393397413737));
#33482=CARTESIAN_POINT('Ctrl Pts',(41.924151672043,45.1667497798393,-7.71980323240516));
#33483=CARTESIAN_POINT('Ctrl Pts',(41.9196903893103,46.0023244618346,-7.76038497140452));
#33484=CARTESIAN_POINT('Origin',(46.,46.,2.76038497140452));
#33485=CARTESIAN_POINT('',(41.9114695346733,46.0028257844758,-5.26038497140452));
#33486=CARTESIAN_POINT('',(41.92081287872,45.9987553743592,-5.36461502859548));
#33487=CARTESIAN_POINT('',(41.915,46.0000000000001,2.76038497140452));
#33488=CARTESIAN_POINT('Ctrl Pts',(41.92081287872,45.9987553743592,-5.36461502859548));
#33489=CARTESIAN_POINT('Ctrl Pts',(41.9229289320299,46.7532680949118,-5.40123467223189));
#33490=CARTESIAN_POINT('Ctrl Pts',(42.4823086036718,48.8558848674044,-5.50314183513673));
#33491=CARTESIAN_POINT('Ctrl Pts',(45.8362350743765,50.8045030456205,-5.67033651731001));
#33492=CARTESIAN_POINT('Ctrl Pts',(49.9115571874415,48.7945999936567,-5.86619907511531));
#33493=CARTESIAN_POINT('Ctrl Pts',(50.4920526914155,44.2878292749147,-6.0620616329206));
#33494=CARTESIAN_POINT('Ctrl Pts',(47.059072278606,41.3108170258638,-6.2579241907259));
#33495=CARTESIAN_POINT('Ctrl Pts',(42.9409562421533,42.4511109778925,-6.44210865595085));
#33496=CARTESIAN_POINT('Ctrl Pts',(41.9222791837043,44.9041620832633,-6.56100560190738));
#33497=CARTESIAN_POINT('Ctrl Pts',(41.9127963736709,46.0032209041833,-6.61461502859548));
#33498=CARTESIAN_POINT('Ctrl Pts',(41.9114695346733,46.0028257844758,-5.26038497140452));
#33499=CARTESIAN_POINT('Ctrl Pts',(41.9099561249016,46.1933541918985,-5.26968633451732));
#33500=CARTESIAN_POINT('Ctrl Pts',(42.0077820074887,47.7196665524005,-5.34427521689856));
#33501=CARTESIAN_POINT('Ctrl Pts',(43.926226788663,50.3369968125737,-5.48415161854822));
#33502=CARTESIAN_POINT('Ctrl Pts',(48.4653744868355,50.126985023971,-5.68001417635351));
#33503=CARTESIAN_POINT('Ctrl Pts',(50.8018046472976,46.229670491242,-5.87587673415881));
#33504=CARTESIAN_POINT('Ctrl Pts',(48.8480067336088,42.1271542042059,-6.07173929196409));
#33505=CARTESIAN_POINT('Ctrl Pts',(44.3496239015183,41.4848769748296,-6.26760184976939));
#33506=CARTESIAN_POINT('Ctrl Pts',(42.092272202268,44.0169308928917,-6.41381707624953));
#33507=CARTESIAN_POINT('Ctrl Pts',(41.9123314513927,45.6753959905429,-6.49474478346124));
#33508=CARTESIAN_POINT('Ctrl Pts',(41.915141161974,45.9965141266804,-6.51038497140452));
#33509=CARTESIAN_POINT('Origin',(46.,46.,2.76038497140452));
#33510=CARTESIAN_POINT('',(41.9211344995594,45.9994902409546,-4.01038497140451));
#33511=CARTESIAN_POINT('',(41.909115223572,45.99869298379,-4.11461502859548));
#33512=CARTESIAN_POINT('',(41.915,46.0000000000001,2.76038497140452));
#33513=CARTESIAN_POINT('Ctrl Pts',(41.909115223572,45.99869298379,-4.11461502859548));
#33514=CARTESIAN_POINT('Ctrl Pts',(41.9144794832991,47.2577928076527,-4.17617622328797));
#33515=CARTESIAN_POINT('Ctrl Pts',(43.2050473399624,49.8617288828865,-4.3030249372489));
#33516=CARTESIAN_POINT('Ctrl Pts',(47.6123997659237,50.5288227185664,-4.49516117047825));
#33517=CARTESIAN_POINT('Ctrl Pts',(50.6646118667576,47.1625249946476,-4.69102372828354));
#33518=CARTESIAN_POINT('Ctrl Pts',(49.5491722744117,42.7575558053009,-4.88688628608884));
#33519=CARTESIAN_POINT('Ctrl Pts',(45.2626834729594,41.249586062651,-5.08274884389413));
#33520=CARTESIAN_POINT('Ctrl Pts',(42.3132199522082,43.4743257401283,-5.24199175806301));
#33521=CARTESIAN_POINT('Ctrl Pts',(41.9191563155453,45.4080812255242,-5.33594715296346));
#33522=CARTESIAN_POINT('Ctrl Pts',(41.92081287872,45.9987553743592,-5.36461502859548));
#33523=CARTESIAN_POINT('Ctrl Pts',(41.9211344995594,45.9994902409546,-4.01038497140451));
#33524=CARTESIAN_POINT('Ctrl Pts',(41.9219410836274,46.7051726957788,-4.0446278855734));
#33525=CARTESIAN_POINT('Ctrl Pts',(42.4288873183858,48.757394326904,-4.14415831901071));
#33526=CARTESIAN_POINT('Ctrl Pts',(45.664182571157,50.7955503680233,-4.30897627171645));
#33527=CARTESIAN_POINT('Ctrl Pts',(49.8089081243513,48.9329670248342,-4.50483882952175));
#33528=CARTESIAN_POINT('Ctrl Pts',(50.5505204413009,44.4498902060922,-4.70070138732704));
#33529=CARTESIAN_POINT('Ctrl Pts',(47.226417382704,41.351776998474,-4.89656394513234));
#33530=CARTESIAN_POINT('Ctrl Pts',(43.0164532244616,42.3565764685033,-5.08312513982482));
#33531=CARTESIAN_POINT('Ctrl Pts',(41.9205789517317,44.8560096629367,-5.20439881524889));
#33532=CARTESIAN_POINT('Ctrl Pts',(41.9114695346733,46.0028257844758,-5.26038497140452));
#33533=CARTESIAN_POINT('Origin',(46.,46.,2.76038497140452));
#33534=CARTESIAN_POINT('',(41.9099451845995,45.9979581674561,-2.76038497140452));
#33535=CARTESIAN_POINT('',(41.9182052434271,46.003032374089,-2.86461502859548));
#33536=CARTESIAN_POINT('',(41.915,46.0000000000001,2.76038497140452));
#33537=CARTESIAN_POINT('Ctrl Pts',(41.918205243427,46.003032374089,-2.86461502859548));
#33538=CARTESIAN_POINT('Ctrl Pts',(41.9150894442525,46.4394483130513,-2.88583025507562));
#33539=CARTESIAN_POINT('Ctrl Pts',(42.1787199801138,48.2152230225309,-2.97233300082419));
#33540=CARTESIAN_POINT('Ctrl Pts',(44.7345906088731,50.6377588369492,-3.1241232658412));
#33541=CARTESIAN_POINT('Ctrl Pts',(49.1631528076755,49.6200183172327,-3.31998582364649));
#33542=CARTESIAN_POINT('Ctrl Pts',(50.7655593735804,45.3679303091532,-3.51584838145178));
#33543=CARTESIAN_POINT('Ctrl Pts',(48.1101215244772,41.6805723363936,-3.71171093925708));
#33544=CARTESIAN_POINT('Ctrl Pts',(43.5693710758889,41.8524572016734,-3.90757349706237));
#33545=CARTESIAN_POINT('Ctrl Pts',(41.9449143886546,44.5112652628352,-4.04187486017517));
#33546=CARTESIAN_POINT('Ctrl Pts',(41.9087905227121,45.9224791506983,-4.11088870401954));
#33547=CARTESIAN_POINT('Ctrl Pts',(41.909115223572,45.99869298379,-4.11461502859548));
#33548=CARTESIAN_POINT('Ctrl Pts',(41.9099451845995,45.9979581674561,-2.76038497140452));
#33549=CARTESIAN_POINT('Ctrl Pts',(41.9174621235915,47.2091008131617,-2.81956943662948));
#33550=CARTESIAN_POINT('Ctrl Pts',(43.1226545649493,49.769299341883,-2.94404142112287));
#33551=CARTESIAN_POINT('Ctrl Pts',(47.4490851541316,50.5836916797423,-3.1338009248847));
#33552=CARTESIAN_POINT('Ctrl Pts',(50.619960918391,47.3289236340817,-3.32966348268999));
#33553=CARTESIAN_POINT('Ctrl Pts',(49.6630787639445,42.8868134693702,-3.52552604049528));
#33554=CARTESIAN_POINT('Ctrl Pts',(45.4333763810852,41.2262159220479,-3.72138859830058));
#33555=CARTESIAN_POINT('Ctrl Pts',(42.3609054830561,43.3754463728178,-3.88300824193698));
#33556=CARTESIAN_POINT('Ctrl Pts',(41.9204032509354,45.3597189578316,-3.97934036630497));
#33557=CARTESIAN_POINT('Ctrl Pts',(41.9211344995594,45.9994902409546,-4.01038497140451));
#33558=CARTESIAN_POINT('Origin',(46.,46.,2.76038497140452));
#33559=CARTESIAN_POINT('',(41.9169756956685,46.0033346419049,-1.51038497140452));
#33560=CARTESIAN_POINT('',(41.9171329418229,45.9966889238588,-1.61461502859548));
#33561=CARTESIAN_POINT('',(41.915,46.0000000000001,2.76038497140452));
#33562=CARTESIAN_POINT('Ctrl Pts',(41.9171329418229,45.9966889238588,-1.61461502859548));
#33563=CARTESIAN_POINT('Ctrl Pts',(41.9246775568123,46.9455421599706,-1.6607718061317));
#33564=CARTESIAN_POINT('Ctrl Pts',(42.7226626973778,49.2479787911961,-1.77221610293635));
#33565=CARTESIAN_POINT('Ctrl Pts',(46.5265139156528,50.7783713513675,-1.94894791900943));
#33566=CARTESIAN_POINT('Ctrl Pts',(50.2717006433544,48.205140538033,-2.14481047681473));
#33567=CARTESIAN_POINT('Ctrl Pts',(50.2002873368139,43.661697764522,-2.34067303462002));
#33568=CARTESIAN_POINT('Ctrl Pts',(46.3760782190255,41.2074400215055,-2.53653559242531));
#33569=CARTESIAN_POINT('Ctrl Pts',(42.6664799891873,42.8371779761014,-2.71118292375047));
#33570=CARTESIAN_POINT('Ctrl Pts',(41.9246779725125,45.0964264013728,-2.82054273580719));
#33571=CARTESIAN_POINT('Ctrl Pts',(41.918205243427,46.003032374089,-2.86461502859548));
#33572=CARTESIAN_POINT('Ctrl Pts',(41.9169756956685,46.0033346419049,-1.51038497140452));
#33573=CARTESIAN_POINT('Ctrl Pts',(41.9138563439275,46.390566259229,-1.52922346841713));
#33574=CARTESIAN_POINT('Ctrl Pts',(42.1404155757815,48.1162325445959,-1.61334948469817));
#33575=CARTESIAN_POINT('Ctrl Pts',(44.5692318828111,50.5894261400569,-1.76276302024764));
#33576=CARTESIAN_POINT('Ctrl Pts',(49.0314017551548,49.7310441604199,-1.95862557805294));
#33577=CARTESIAN_POINT('Ctrl Pts',(50.7851513154972,45.5390953919881,-2.15448813585823));
#33578=CARTESIAN_POINT('Ctrl Pts',(48.2635416323089,41.7589579733313,-2.35035069366352));
#33579=CARTESIAN_POINT('Ctrl Pts',(43.7195493508676,41.7680235772757,-2.54621325146881));
#33580=CARTESIAN_POINT('Ctrl Pts',(41.9704474010668,44.4129095021318,-2.68289134404915));
#33581=CARTESIAN_POINT('Ctrl Pts',(41.9091700439484,45.8730661203117,-2.75428191736105));
#33582=CARTESIAN_POINT('Ctrl Pts',(41.9099451845995,45.9979581674561,-2.76038497140452));
#33583=CARTESIAN_POINT('Origin',(46.,46.,2.76038497140452));
#33584=CARTESIAN_POINT('',(41.9194198683446,45.9961669413359,-0.260384971404518));
#33585=CARTESIAN_POINT('',(41.9098427756084,46.0018622022123,-0.364615028595478));
#33586=CARTESIAN_POINT('',(41.915,46.0000000000001,2.76038497140452));
#33587=CARTESIAN_POINT('',(44.942095577027,42.0543614925016,0.));
#33588=CARTESIAN_POINT('Ctrl Pts',(44.942095577027,42.0543614925016,0.));
#33589=CARTESIAN_POINT('Ctrl Pts',(43.6472519732775,42.4015349025496,-0.0652875192684312));
#33590=CARTESIAN_POINT('Ctrl Pts',(42.1846936066115,43.7726390243385,-0.152082509736604));
#33591=CARTESIAN_POINT('Ctrl Pts',(41.9164511209723,45.5536935953327,-0.238877500204776));
#33592=CARTESIAN_POINT('Ctrl Pts',(41.9194198683446,45.9961669413359,-0.260384971404518));
#33593=CARTESIAN_POINT('',(47.0606472822454,42.0481878432335,2.51247271755868E-15));
#33594=CARTESIAN_POINT('Origin',(46.,46.,0.));
#33595=CARTESIAN_POINT('Ctrl Pts',(47.0606640384105,42.0481501283249,1.75098650856409E-16));
#33596=CARTESIAN_POINT('Ctrl Pts',(45.8335722254876,41.7236247803045,-0.0620616329205975));
#33597=CARTESIAN_POINT('Ctrl Pts',(43.1010253798376,42.2867107335592,-0.183599975785757));
#33598=CARTESIAN_POINT('Ctrl Pts',(41.9171104642337,44.7850381248174,-0.305138318650916));
#33599=CARTESIAN_POINT('Ctrl Pts',(41.9098427756084,46.0018622022123,-0.364615028595478));
#33600=CARTESIAN_POINT('Origin',(60.,-60.,-6.));
#33601=CARTESIAN_POINT('',(64.262772575926,-60.0000736173382,-4.57968167058906));
#33602=CARTESIAN_POINT('',(64.2633463740757,-59.9999932305335,-4.17031832941094));
#33603=CARTESIAN_POINT('',(64.263,-60.,-6.));
#33604=CARTESIAN_POINT('',(60.8043894954945,-64.1864216867795,-3.));
#33605=CARTESIAN_POINT('Ctrl Pts',(64.2633463740757,-59.9999932305335,-4.17031832941094));
#33606=CARTESIAN_POINT('Ctrl Pts',(64.2633470323478,-59.99313820065,-4.16993434591159));
#33607=CARTESIAN_POINT('Ctrl Pts',(64.263330832606,-59.9862831738927,-4.16955036241224));
#33608=CARTESIAN_POINT('Ctrl Pts',(64.2632977556816,-59.9794282285766,-4.1691663789129));
#33609=CARTESIAN_POINT('Ctrl Pts',(64.259940629834,-59.2836889926924,-4.13019416628246));
#33610=CARTESIAN_POINT('Ctrl Pts',(64.0827293990401,-58.588788693418,-4.09122195365203));
#33611=CARTESIAN_POINT('Ctrl Pts',(63.7524939347896,-57.9764089025128,-4.0522497410216));
#33612=CARTESIAN_POINT('Ctrl Pts',(63.4222584705391,-57.3640291116076,-4.01327752839118));
#33613=CARTESIAN_POINT('Ctrl Pts',(62.9389987728321,-56.8341698290715,-3.97430531576075));
#33614=CARTESIAN_POINT('Ctrl Pts',(62.3595200338666,-56.4491133284713,-3.93533310313032));
#33615=CARTESIAN_POINT('Ctrl Pts',(61.780041294901,-56.0640568278712,-3.89636089049989));
#33616=CARTESIAN_POINT('Ctrl Pts',(61.104343514677,-55.8238031092071,-3.85738867786946));
#33617=CARTESIAN_POINT('Ctrl Pts',(60.4118497430403,-55.7565921213005,-3.81841646523903));
#33618=CARTESIAN_POINT('Ctrl Pts',(59.7193559714036,-55.689381133394,-3.77944425260859));
#33619=CARTESIAN_POINT('Ctrl Pts',(59.0100662083542,-55.7952128762451,-3.74047203997817));
#33620=CARTESIAN_POINT('Ctrl Pts',(58.367356732413,-56.0616485702291,-3.70149982734774));
#33621=CARTESIAN_POINT('Ctrl Pts',(57.7246472564718,-56.3280842642132,-3.66252761471731));
#33622=CARTESIAN_POINT('Ctrl Pts',(57.1485180676388,-56.7551239093303,-3.62355540208688));
#33623=CARTESIAN_POINT('Ctrl Pts',(56.7066830424806,-57.2925687565161,-3.58458318945645));
#33624=CARTESIAN_POINT('Ctrl Pts',(56.2648480173224,-57.8300136037019,-3.54561097682602));
#33625=CARTESIAN_POINT('Ctrl Pts',(55.9573071558389,-58.4778636529564,-3.50663876419559));
#33626=CARTESIAN_POINT('Ctrl Pts',(55.8202250112632,-59.1599728770642,-3.46766655156516));
#33627=CARTESIAN_POINT('Ctrl Pts',(55.6831428666875,-59.842082101172,-3.42869433893473));
#33628=CARTESIAN_POINT('Ctrl Pts',(55.7165194390194,-60.558450500133,-3.3897221263043));
#33629=CARTESIAN_POINT('Ctrl Pts',(55.9163989736504,-61.2248597751814,-3.35074991367387));
#33630=CARTESIAN_POINT('Ctrl Pts',(56.1162785082814,-61.8912690502299,-3.31177770104344));
#33631=CARTESIAN_POINT('Ctrl Pts',(56.4826610052114,-62.5077192013657,-3.27280548841301));
#33632=CARTESIAN_POINT('Ctrl Pts',(56.9725485708617,-63.0017699164546,-3.23383327578258));
#33633=CARTESIAN_POINT('Ctrl Pts',(57.462436136512,-63.4958206315434,-3.19486106315215));
#33634=CARTESIAN_POINT('Ctrl Pts',(58.0758287708825,-63.8674719105853,-3.15588885052172));
#33635=CARTESIAN_POINT('Ctrl Pts',(58.740462519741,-64.0729506012584,-3.11691663789129));
#33636=CARTESIAN_POINT('Ctrl Pts',(59.4050962685994,-64.2784292919315,-3.07794442526086));
#33637=CARTESIAN_POINT('Ctrl Pts',(60.1209711319459,-64.3177353942359,-3.03897221263043));
#33638=CARTESIAN_POINT('Ctrl Pts',(60.8043894954946,-64.1864216867795,-3.));
#33639=CARTESIAN_POINT('',(64.0279239112946,-58.6032685651144,-3.00000000000001));
#33640=CARTESIAN_POINT('Origin',(60.,-60.,-3.));
#33641=CARTESIAN_POINT('',(64.2630923571199,-60.0000961870058,-3.07968167058906));
#33642=CARTESIAN_POINT('Ctrl Pts',(64.0279239112946,-58.6032685651144,-3.00000000000001));
#33643=CARTESIAN_POINT('Ctrl Pts',(64.1829036812454,-59.0514416549545,-3.02656055686302));
#33644=CARTESIAN_POINT('Ctrl Pts',(64.2626358475693,-59.5258438271314,-3.05312111372604));
#33645=CARTESIAN_POINT('Ctrl Pts',(64.2630923571199,-60.0000961870058,-3.07968167058906));
#33646=CARTESIAN_POINT('',(64.263,-60.,-2.));
#33647=CARTESIAN_POINT('',(64.263,-60.,-6.));
#33648=CARTESIAN_POINT('Origin',(60.,-60.,-2.));
#33649=CARTESIAN_POINT('Ctrl Pts',(64.2630923571199,-60.0000961870058,-3.07968167058906));
#33650=CARTESIAN_POINT('Ctrl Pts',(64.2632197548392,-60.1324453765281,-3.08709390186401));
#33651=CARTESIAN_POINT('Ctrl Pts',(64.2571731981271,-60.264782898732,-3.09450613313896));
#33652=CARTESIAN_POINT('Ctrl Pts',(64.2448651421447,-60.396535440406,-3.10191836441391));
#33653=CARTESIAN_POINT('Ctrl Pts',(64.1801515414727,-61.0892672074344,-3.14089057704434));
#33654=CARTESIAN_POINT('Ctrl Pts',(63.9423405435201,-61.7658273512139,-3.17986278967477));
#33655=CARTESIAN_POINT('Ctrl Pts',(63.5593783222426,-62.3466916938238,-3.2188350023052));
#33656=CARTESIAN_POINT('Ctrl Pts',(63.1764161009651,-62.9275560364337,-3.25780721493563));
#33657=CARTESIAN_POINT('Ctrl Pts',(62.6483026563626,-63.4127245778742,-3.29677942756606));
#33658=CARTESIAN_POINT('Ctrl Pts',(62.037118094178,-63.7451676100945,-3.33575164019649));
#33659=CARTESIAN_POINT('Ctrl Pts',(61.4259335319934,-64.0776106423148,-3.37472385282692));
#33660=CARTESIAN_POINT('Ctrl Pts',(60.7316778522266,-64.257328165315,-3.41369606545735));
#33661=CARTESIAN_POINT('Ctrl Pts',(60.03595543146,-64.2631957584035,-3.45266827808778));
#33662=CARTESIAN_POINT('Ctrl Pts',(59.3402330106934,-64.269063351492,-3.49164049071821));
#33663=CARTESIAN_POINT('Ctrl Pts',(58.6430438489269,-64.1010810146688,-3.53061270334864));
#33664=CARTESIAN_POINT('Ctrl Pts',(58.0263393834232,-63.7789939606085,-3.56958491597907));
#33665=CARTESIAN_POINT('Ctrl Pts',(57.4096349179195,-63.4569069065482,-3.6085571286095));
#33666=CARTESIAN_POINT('Ctrl Pts',(56.8734151486786,-62.9807151352507,-3.64752934123993));
#33667=CARTESIAN_POINT('Ctrl Pts',(56.4807094070791,-62.4063924445202,-3.68650155387036));
#33668=CARTESIAN_POINT('Ctrl Pts',(56.0880036654796,-61.8320697537898,-3.72547376650079));
#33669=CARTESIAN_POINT('Ctrl Pts',(55.8388119515216,-61.1596161436264,-3.76444597913122));
#33670=CARTESIAN_POINT('Ctrl Pts',(55.7624255353169,-60.4680747538138,-3.80341819176165));
#33671=CARTESIAN_POINT('Ctrl Pts',(55.6860391191123,-59.7765333640012,-3.84239040439208));
#33672=CARTESIAN_POINT('Ctrl Pts',(55.7824580006609,-59.0659041945396,-3.88136261702251));
#33673=CARTESIAN_POINT('Ctrl Pts',(56.0403485787269,-58.4197178343383,-3.92033482965294));
#33674=CARTESIAN_POINT('Ctrl Pts',(56.298239156793,-57.7735314741371,-3.95930704228337));
#33675=CARTESIAN_POINT('Ctrl Pts',(56.7176014313765,-57.1917879231964,-3.9982792549138));
#33676=CARTESIAN_POINT('Ctrl Pts',(57.2491417753782,-56.7428678065456,-4.03725146754423));
#33677=CARTESIAN_POINT('Ctrl Pts',(57.7806821193799,-56.2939476898949,-4.07622368017466));
#33678=CARTESIAN_POINT('Ctrl Pts',(58.4244005327997,-55.977851007534,-4.11519589280509));
#33679=CARTESIAN_POINT('Ctrl Pts',(59.1046313480008,-55.8317333957891,-4.15416810543552));
#33680=CARTESIAN_POINT('Ctrl Pts',(59.7848621632019,-55.6856157840441,-4.19314031806595));
#33681=CARTESIAN_POINT('Ctrl Pts',(60.5016053801842,-55.709477242915,-4.23211253069638));
#33682=CARTESIAN_POINT('Ctrl Pts',(61.1706120606455,-55.9005125186762,-4.27108474332681));
#33683=CARTESIAN_POINT('Ctrl Pts',(61.8396187411067,-56.0915477944374,-4.31005695595724));
#33684=CARTESIAN_POINT('Ctrl Pts',(62.4608888850469,-56.4497568870889,-4.34902916858767));
#33685=CARTESIAN_POINT('Ctrl Pts',(62.9613950792328,-56.9330353155764,-4.3880013812181));
#33686=CARTESIAN_POINT('Ctrl Pts',(63.4619012734186,-57.4163137440639,-4.42697359384853));
#33687=CARTESIAN_POINT('Ctrl Pts',(63.8416435178501,-58.0246615083876,-4.46594580647895));
#33688=CARTESIAN_POINT('Ctrl Pts',(64.0559863899328,-58.6865685071185,-4.50491801910938));
#33689=CARTESIAN_POINT('Ctrl Pts',(64.1930503363015,-59.1098323390043,-4.52983923626927));
#33690=CARTESIAN_POINT('Ctrl Pts',(64.262480725507,-59.5549971097538,-4.55476045342917));
#33691=CARTESIAN_POINT('Ctrl Pts',(64.262772575926,-60.0000736173382,-4.57968167058906));
#33692=CARTESIAN_POINT('Origin',(60.,-60.,-6.));
#33693=CARTESIAN_POINT('',(64.2626973681969,-59.9946117577646,-6.07968167058905));
#33694=CARTESIAN_POINT('',(64.2632169240698,-60.0000544407254,-5.67031832941094));
#33695=CARTESIAN_POINT('',(64.263,-60.,-6.));
#33696=CARTESIAN_POINT('Ctrl Pts',(64.2632169240698,-60.0000544407254,-5.67031832941094));
#33697=CARTESIAN_POINT('Ctrl Pts',(64.2626871719434,-59.4158863751755,-5.63760089747675));
#33698=CARTESIAN_POINT('Ctrl Pts',(64.1414983098939,-58.8315462195081,-5.60488346554256));
#33699=CARTESIAN_POINT('Ctrl Pts',(63.9080437096925,-58.2961477521629,-5.57216603360837));
#33700=CARTESIAN_POINT('Ctrl Pts',(63.6299582432996,-57.65839406314,-5.53319382097794));
#33701=CARTESIAN_POINT('Ctrl Pts',(63.1925789493251,-57.0900837233481,-5.49422160834751));
#33702=CARTESIAN_POINT('Ctrl Pts',(62.6472141694011,-56.6580726270348,-5.45524939571708));
#33703=CARTESIAN_POINT('Ctrl Pts',(62.1018493894771,-56.2260615307214,-5.41627718308665));
#33704=CARTESIAN_POINT('Ctrl Pts',(61.4484991236035,-55.9303496778867,-5.37730497045622));
#33705=CARTESIAN_POINT('Ctrl Pts',(60.7640088680538,-55.805671270223,-5.33833275782579));
#33706=CARTESIAN_POINT('Ctrl Pts',(60.0795186125042,-55.6809928625592,-5.29936054519536));
#33707=CARTESIAN_POINT('Ctrl Pts',(59.3638883672783,-55.7273479000665,-5.26038833256493));
#33708=CARTESIAN_POINT('Ctrl Pts',(58.7012143744383,-55.9392992230255,-5.2214161199345));
#33709=CARTESIAN_POINT('Ctrl Pts',(58.0385403815983,-56.1512505459845,-5.18244390730407));
#33710=CARTESIAN_POINT('Ctrl Pts',(57.428822641144,-56.5287981543954,-5.14347169467364));
#33711=CARTESIAN_POINT('Ctrl Pts',(56.9437403484681,-57.0275580359404,-5.10449948204321));
#33712=CARTESIAN_POINT('Ctrl Pts',(56.4586580557921,-57.5263179174854,-5.06552726941278));
#33713=CARTESIAN_POINT('Ctrl Pts',(56.0982112108944,-58.1462900721645,-5.02655505678235));
#33714=CARTESIAN_POINT('Ctrl Pts',(55.9047635971807,-58.8146026972723,-4.98758284415192));
#33715=CARTESIAN_POINT('Ctrl Pts',(55.711315983467,-59.4829153223801,-4.94861063152149));
#33716=CARTESIAN_POINT('Ctrl Pts',(55.6848676009373,-60.1995684179167,-4.90963841889106));
#33717=CARTESIAN_POINT('Ctrl Pts',(55.8285295105432,-60.8803222262535,-4.87066620626063));
#33718=CARTESIAN_POINT('Ctrl Pts',(55.972191420149,-61.5610760345903,-4.8316939936302));
#33719=CARTESIAN_POINT('Ctrl Pts',(56.2859636218904,-62.2059305557273,-4.79272178099977));
#33720=CARTESIAN_POINT('Ctrl Pts',(56.7329629091576,-62.7390872440468,-4.75374956836934));
#33721=CARTESIAN_POINT('Ctrl Pts',(57.1799621964249,-63.2722439323662,-4.71477735573891));
#33722=CARTESIAN_POINT('Ctrl Pts',(57.7601885692179,-63.693702787868,-4.67580514310848));
#33723=CARTESIAN_POINT('Ctrl Pts',(58.4054401079131,-63.9539234102185,-4.63683293047805));
#33724=CARTESIAN_POINT('Ctrl Pts',(59.0506916466083,-64.214144032569,-4.59786071784762));
#33725=CARTESIAN_POINT('Ctrl Pts',(59.7609683512056,-64.3131264217682,-4.55888850521719));
#33726=CARTESIAN_POINT('Ctrl Pts',(60.4527808941947,-64.239235855233,-4.51991629258676));
#33727=CARTESIAN_POINT('Ctrl Pts',(61.1445934371838,-64.1653452886979,-4.48094407995633));
#33728=CARTESIAN_POINT('Ctrl Pts',(61.8179418185646,-63.9185817664285,-4.4419718673259));
#33729=CARTESIAN_POINT('Ctrl Pts',(62.393677796486,-63.527950932842,-4.40299965469547));
#33730=CARTESIAN_POINT('Ctrl Pts',(62.9694137744075,-63.1373200992555,-4.36402744206504));
#33731=CARTESIAN_POINT('Ctrl Pts',(63.4475373488694,-62.6028219543521,-4.32505522943461));
#33732=CARTESIAN_POINT('Ctrl Pts',(63.7718476256499,-61.9872837956534,-4.28608301680418));
#33733=CARTESIAN_POINT('Ctrl Pts',(64.0929625540898,-61.377810381043,-4.2474947876731));
#33734=CARTESIAN_POINT('Ctrl Pts',(64.263280221346,-60.6888860196627,-4.20890655854202));
#33735=CARTESIAN_POINT('Ctrl Pts',(64.2633463740757,-59.9999932305335,-4.17031832941094));
#33736=CARTESIAN_POINT('Ctrl Pts',(64.262772575926,-60.0000736173382,-4.57968167058906));
#33737=CARTESIAN_POINT('Ctrl Pts',(64.2629371260315,-60.2510151324331,-4.5937326660596));
#33738=CARTESIAN_POINT('Ctrl Pts',(64.2411232856546,-60.5019285896265,-4.60778366153014));
#33739=CARTESIAN_POINT('Ctrl Pts',(64.1970613151823,-60.7488728385771,-4.62183465700067));
#33740=CARTESIAN_POINT('Ctrl Pts',(64.0748498686155,-61.4338039381665,-4.6608068696311));
#33741=CARTESIAN_POINT('Ctrl Pts',(63.7814834757479,-62.0881999042072,-4.69977908226153));
#33742=CARTESIAN_POINT('Ctrl Pts',(63.3514512075064,-62.6351299077276,-4.73875129489196));
#33743=CARTESIAN_POINT('Ctrl Pts',(62.9214189392649,-63.1820599112481,-4.77772350752239));
#33744=CARTESIAN_POINT('Ctrl Pts',(62.3547207956494,-63.6215239522483,-4.81669572015282));
#33745=CARTESIAN_POINT('Ctrl Pts',(61.7179571845381,-63.9018875004117,-4.85566793278325));
#33746=CARTESIAN_POINT('Ctrl Pts',(61.0811935734268,-64.1822510485752,-4.89464014541368));
#33747=CARTESIAN_POINT('Ctrl Pts',(60.3743644948197,-64.3035141039018,-4.93361235804411));
#33748=CARTESIAN_POINT('Ctrl Pts',(59.6805793190517,-64.2513752851793,-4.97258457067454));
#33749=CARTESIAN_POINT('Ctrl Pts',(58.9867941432837,-64.1992364664568,-5.01155678330497));
#33750=CARTESIAN_POINT('Ctrl Pts',(58.3060528703548,-63.9736957736851,-5.0505289959354));
#33751=CARTESIAN_POINT('Ctrl Pts',(57.7183177603327,-63.6013669799594,-5.08950120856583));
#33752=CARTESIAN_POINT('Ctrl Pts',(57.1305826503106,-63.2290381862337,-5.12847342119626));
#33753=CARTESIAN_POINT('Ctrl Pts',(56.6358537031954,-62.7099212915541,-5.16744563382669));
#33754=CARTESIAN_POINT('Ctrl Pts',(56.2924025713763,-62.1048137589543,-5.20641784645712));
#33755=CARTESIAN_POINT('Ctrl Pts',(55.9489514395571,-61.4997062263544,-5.24539005908755));
#33756=CARTESIAN_POINT('Ctrl Pts',(55.756778123034,-60.8086080558343,-5.28436227171798));
#33757=CARTESIAN_POINT('Ctrl Pts',(55.7382146651663,-60.1132326609549,-5.32333448434841));
#33758=CARTESIAN_POINT('Ctrl Pts',(55.7196512072987,-59.4178572660755,-5.36230669697884));
#33759=CARTESIAN_POINT('Ctrl Pts',(55.8746976080865,-58.7182046468368,-5.40127890960927));
#33760=CARTESIAN_POINT('Ctrl Pts',(56.1856839927028,-58.095480130689,-5.4402511222397));
#33761=CARTESIAN_POINT('Ctrl Pts',(56.4966703773191,-57.4727556145412,-5.47922333487013));
#33762=CARTESIAN_POINT('Ctrl Pts',(56.9635967457639,-56.9269592014842,-5.51819554750056));
#33763=CARTESIAN_POINT('Ctrl Pts',(57.5303812800693,-56.5244725420488,-5.55716776013099));
#33764=CARTESIAN_POINT('Ctrl Pts',(58.0971658143748,-56.1219858826134,-5.59613997276142));
#33765=CARTESIAN_POINT('Ctrl Pts',(58.7638085145408,-55.8628089767996,-5.63511218539185));
#33766=CARTESIAN_POINT('Ctrl Pts',(59.4545507191691,-55.772604446058,-5.67408439802228));
#33767=CARTESIAN_POINT('Ctrl Pts',(60.1452929237973,-55.6823999153164,-5.71305661065271));
#33768=CARTESIAN_POINT('Ctrl Pts',(60.8601346328878,-55.761167759647,-5.75202882328314));
#33769=CARTESIAN_POINT('Ctrl Pts',(61.5092342355577,-56.009115703567,-5.79100103591357));
#33770=CARTESIAN_POINT('Ctrl Pts',(62.8074334408974,-56.5050115914071,-5.86894546117443));
#33771=CARTESIAN_POINT('Ctrl Pts',(63.8426642205549,-57.6776278776046,-5.94688988643529));
#33772=CARTESIAN_POINT('Ctrl Pts',(64.1576092650939,-59.0258076707621,-6.02483431169615));
#33773=CARTESIAN_POINT('Ctrl Pts',(64.2314820012626,-59.3420334120301,-6.04311676466045));
#33774=CARTESIAN_POINT('Ctrl Pts',(64.2657266032027,-59.6679181731568,-6.06139921762475));
#33775=CARTESIAN_POINT('Ctrl Pts',(64.2626973681969,-59.9946117577646,-6.07968167058905));
#33776=CARTESIAN_POINT('Origin',(60.,-60.,-6.));
#33777=CARTESIAN_POINT('',(64.2628730310814,-59.999902186829,-7.57968167058906));
#33778=CARTESIAN_POINT('',(64.2625444778277,-60.0004819773136,-7.17031832941094));
#33779=CARTESIAN_POINT('',(64.263,-60.,-6.));
#33780=CARTESIAN_POINT('Ctrl Pts',(64.2625444778277,-60.0004819773136,-7.17031832941094));
#33781=CARTESIAN_POINT('Ctrl Pts',(64.2617098238277,-59.5354191820522,-7.14423966167234));
#33782=CARTESIAN_POINT('Ctrl Pts',(64.1851000643309,-59.0702106162843,-7.11816099393373));
#33783=CARTESIAN_POINT('Ctrl Pts',(64.0358045844181,-58.6286233477238,-7.09208232619513));
#33784=CARTESIAN_POINT('Ctrl Pts',(63.8126959790919,-57.9687110739172,-7.0531101135647));
#33785=CARTESIAN_POINT('Ctrl Pts',(63.4272612479163,-57.3615513028208,-7.01413790093427));
#33786=CARTESIAN_POINT('Ctrl Pts',(62.9188673674461,-56.8879014639496,-6.97516568830384));
#33787=CARTESIAN_POINT('Ctrl Pts',(61.9020796065058,-55.9406017862071,-6.89722126304298));
#33788=CARTESIAN_POINT('Ctrl Pts',(60.3934552483873,-55.5273418373652,-6.81927683778212));
#33789=CARTESIAN_POINT('Ctrl Pts',(59.0443044051678,-55.8381001101711,-6.74133241252126));
#33790=CARTESIAN_POINT('Ctrl Pts',(57.6951535619483,-56.1488583829769,-6.6633879872604));
#33791=CARTESIAN_POINT('Ctrl Pts',(56.5054762336278,-57.1836348774304,-6.58544356199954));
#33792=CARTESIAN_POINT('Ctrl Pts',(56.01072650476,-58.476693811765,-6.50749913673868));
#33793=CARTESIAN_POINT('Ctrl Pts',(55.5159767758922,-59.7697527460996,-6.42955471147783));
#33794=CARTESIAN_POINT('Ctrl Pts',(55.7161546464771,-61.3210941203152,-6.35161028621697));
#33795=CARTESIAN_POINT('Ctrl Pts',(56.5133859887326,-62.4593630767463,-6.27366586095611));
#33796=CARTESIAN_POINT('Ctrl Pts',(56.9120016598604,-63.0284975549619,-6.23469364832568));
#33797=CARTESIAN_POINT('Ctrl Pts',(57.4598806989058,-63.4943639287313,-6.19572143569525));
#33798=CARTESIAN_POINT('Ctrl Pts',(58.0825013140338,-63.8067822836796,-6.15674922306482));
#33799=CARTESIAN_POINT('Ctrl Pts',(58.7051219291619,-64.1192006386278,-6.11777701043439));
#33800=CARTESIAN_POINT('Ctrl Pts',(59.4024841203727,-64.2781709747548,-6.07880479780396));
#33801=CARTESIAN_POINT('Ctrl Pts',(60.0974621223944,-64.2624885664828,-6.03983258517353));
#33802=CARTESIAN_POINT('Ctrl Pts',(60.7924401244162,-64.2468061582107,-6.0008603725431));
#33803=CARTESIAN_POINT('Ctrl Pts',(61.4850339372488,-64.0564710055396,-5.96188815991267));
#33804=CARTESIAN_POINT('Ctrl Pts',(62.0915941530894,-63.7150284794136,-5.92291594728224));
#33805=CARTESIAN_POINT('Ctrl Pts',(62.6981543689299,-63.3735859532875,-5.88394373465181));
#33806=CARTESIAN_POINT('Ctrl Pts',(63.2186809877783,-62.8810360537067,-5.84497152202138));
#33807=CARTESIAN_POINT('Ctrl Pts',(63.5930284383828,-62.2947293311775,-5.80599930939095));
#33808=CARTESIAN_POINT('Ctrl Pts',(63.9673758889872,-61.7084226086483,-5.76702709676052));
#33809=CARTESIAN_POINT('Ctrl Pts',(64.1955441713478,-61.0283590631708,-5.72805488413009));
#33810=CARTESIAN_POINT('Ctrl Pts',(64.2502324931223,-60.3347287713052,-5.68908267149966));
#33811=CARTESIAN_POINT('Ctrl Pts',(64.2590096047169,-60.2234057268317,-5.68282789080342));
#33812=CARTESIAN_POINT('Ctrl Pts',(64.2633181998478,-60.1117332285689,-5.67657311010718));
#33813=CARTESIAN_POINT('Ctrl Pts',(64.2632169240698,-60.0000544407254,-5.67031832941094));
#33814=CARTESIAN_POINT('Ctrl Pts',(64.2626973681969,-59.9946117577646,-6.07968167058905));
#33815=CARTESIAN_POINT('Ctrl Pts',(64.2528119258362,-61.0607260058028,-6.13934364288561));
#33816=CARTESIAN_POINT('Ctrl Pts',(63.8459814397295,-62.1354537612865,-6.19900561518217));
#33817=CARTESIAN_POINT('Ctrl Pts',(63.1240242614618,-62.9112261865645,-6.25866758747873));
#33818=CARTESIAN_POINT('Ctrl Pts',(62.1808349038704,-63.924721609092,-6.33661201273959));
#33819=CARTESIAN_POINT('Ctrl Pts',(60.6997968792671,-64.4279691540293,-6.41455643800045));
#33820=CARTESIAN_POINT('Ctrl Pts',(59.3267918264532,-64.2132809306245,-6.49250086326131));
#33821=CARTESIAN_POINT('Ctrl Pts',(58.6402893000462,-64.1059368189221,-6.53147307589174));
#33822=CARTESIAN_POINT('Ctrl Pts',(57.9807950165867,-63.8191087651342,-6.57044528852217));
#33823=CARTESIAN_POINT('Ctrl Pts',(57.4261724663064,-63.3976167992062,-6.6094175011526));
#33824=CARTESIAN_POINT('Ctrl Pts',(56.8715499160262,-62.9761248332783,-6.64838971378303));
#33825=CARTESIAN_POINT('Ctrl Pts',(56.4217990989253,-62.4199689552105,-6.68736192641346));
#33826=CARTESIAN_POINT('Ctrl Pts',(56.1299141641273,-61.7890621441924,-6.72633413904389));
#33827=CARTESIAN_POINT('Ctrl Pts',(55.8380292293292,-61.1581553331743,-6.76530635167432));
#33828=CARTESIAN_POINT('Ctrl Pts',(55.7040101768341,-60.4524975892059,-6.80427856430475));
#33829=CARTESIAN_POINT('Ctrl Pts',(55.7435429828512,-59.7575619722766,-6.84325077693518));
#33830=CARTESIAN_POINT('Ctrl Pts',(55.7830757888683,-59.0626263553473,-6.88222298956561));
#33831=CARTESIAN_POINT('Ctrl Pts',(55.9961604533976,-58.3784128654571,-6.92119520219604));
#33832=CARTESIAN_POINT('Ctrl Pts',(56.3577826811561,-57.7841730938475,-6.96016741482647));
#33833=CARTESIAN_POINT('Ctrl Pts',(56.7194049089147,-57.1899333222379,-6.9991396274569));
#33834=CARTESIAN_POINT('Ctrl Pts',(57.2295646999025,-56.685667268909,-7.03811184008733));
#33835=CARTESIAN_POINT('Ctrl Pts',(57.828280682058,-56.3311916298766,-7.07708405271776));
#33836=CARTESIAN_POINT('Ctrl Pts',(58.4269966642135,-55.9767159908442,-7.11605626534819));
#33837=CARTESIAN_POINT('Ctrl Pts',(59.1142688375368,-55.7720307661083,-7.15502847797862));
#33838=CARTESIAN_POINT('Ctrl Pts',(59.8093191217818,-55.7409439109291,-7.19400069060904));
#33839=CARTESIAN_POINT('Ctrl Pts',(60.5043694060268,-55.70985705575,-7.23297290323947));
#33840=CARTESIAN_POINT('Ctrl Pts',(61.2071978011936,-55.8523685701277,-7.2719451158699));
#33841=CARTESIAN_POINT('Ctrl Pts',(61.8351875089724,-56.1518435330984,-7.31091732850033));
#33842=CARTESIAN_POINT('Ctrl Pts',(62.4631772167512,-56.4513184960691,-7.34988954113076));
#33843=CARTESIAN_POINT('Ctrl Pts',(63.016328237142,-56.9077569076329,-7.38886175376119));
#33844=CARTESIAN_POINT('Ctrl Pts',(63.4296222200028,-57.4674529852744,-7.42783396639163));
#33845=CARTESIAN_POINT('Ctrl Pts',(63.8429162028636,-58.0271490629158,-7.46680617902206));
#33846=CARTESIAN_POINT('Ctrl Pts',(64.1163531481944,-58.6901028066351,-7.50577839165248));
#33847=CARTESIAN_POINT('Ctrl Pts',(64.2177913673386,-59.3784126701003,-7.54475060428291));
#33848=CARTESIAN_POINT('Ctrl Pts',(64.2480979620442,-59.5840583156947,-7.55639429305163));
#33849=CARTESIAN_POINT('Ctrl Pts',(64.2630514496097,-59.7919673223717,-7.56803798182034));
#33850=CARTESIAN_POINT('Ctrl Pts',(64.2628730310814,-59.999902186829,-7.57968167058906));
#33851=CARTESIAN_POINT('Origin',(60.,-60.,-6.));
#33852=CARTESIAN_POINT('',(64.2632129993401,-59.9999237120662,-9.07968167058906));
#33853=CARTESIAN_POINT('',(64.2626697207193,-59.9999992453659,-8.67031832941094));
#33854=CARTESIAN_POINT('',(64.263,-60.,-6.));
#33855=CARTESIAN_POINT('',(56.7766472160421,-57.2101674189746,-10.));
#33856=CARTESIAN_POINT('Ctrl Pts',(64.2632129993401,-59.9999237120662,-9.07968167058906));
#33857=CARTESIAN_POINT('Ctrl Pts',(64.2627031276559,-60.6063764566768,-9.11364895864636));
#33858=CARTESIAN_POINT('Ctrl Pts',(64.1318733554661,-61.2130420411853,-9.14761624670366));
#33859=CARTESIAN_POINT('Ctrl Pts',(63.8808238845651,-61.7650315954715,-9.18158353476097));
#33860=CARTESIAN_POINT('Ctrl Pts',(63.5927834221001,-62.3983542865008,-9.2205557473914));
#33861=CARTESIAN_POINT('Ctrl Pts',(63.1464855643694,-62.9597013677154,-9.25952796002183));
#33862=CARTESIAN_POINT('Ctrl Pts',(62.5943907479285,-63.3830862528202,-9.29850017265226));
#33863=CARTESIAN_POINT('Ctrl Pts',(62.0422959314875,-63.8064711379249,-9.33747238528269));
#33864=CARTESIAN_POINT('Ctrl Pts',(61.3844041563363,-64.0918938269197,-9.37644459791312));
#33865=CARTESIAN_POINT('Ctrl Pts',(60.6980457544028,-64.2058117593792,-9.41541681054355));
#33866=CARTESIAN_POINT('Ctrl Pts',(60.0116873524693,-64.3197296918386,-9.45438902317398));
#33867=CARTESIAN_POINT('Ctrl Pts',(59.2968623237536,-64.2621428677627,-9.49336123580441));
#33868=CARTESIAN_POINT('Ctrl Pts',(58.6375973345399,-64.0398048735937,-9.53233344843484));
#33869=CARTESIAN_POINT('Ctrl Pts',(57.9783323453263,-63.8174668794247,-9.57130566106527));
#33870=CARTESIAN_POINT('Ctrl Pts',(57.3746273956147,-63.4303777151625,-9.6102778736957));
#33871=CARTESIAN_POINT('Ctrl Pts',(56.8974398008335,-62.9240723226063,-9.64925008632613));
#33872=CARTESIAN_POINT('Ctrl Pts',(56.4202522060524,-62.4177669300501,-9.68822229895656));
#33873=CARTESIAN_POINT('Ctrl Pts',(56.0695819662017,-61.7922453091999,-9.72719451158699));
#33874=CARTESIAN_POINT('Ctrl Pts',(55.8866652661684,-61.1209648644822,-9.76616672421742));
#33875=CARTESIAN_POINT('Ctrl Pts',(55.703748566135,-60.4496844197645,-9.80513893684785));
#33876=CARTESIAN_POINT('Ctrl Pts',(55.6885854059191,-59.7326451511795,-9.84411114947828));
#33877=CARTESIAN_POINT('Ctrl Pts',(55.8429525213217,-59.0543161036114,-9.88308336210871));
#33878=CARTESIAN_POINT('Ctrl Pts',(55.9973196367243,-58.3759870560434,-9.92205557473914));
#33879=CARTESIAN_POINT('Ctrl Pts',(56.3212170277455,-57.7363682294923,-9.96102778736957));
#33880=CARTESIAN_POINT('Ctrl Pts',(56.7766472160421,-57.2101674189746,-10.));
#33881=CARTESIAN_POINT('',(63.2235668665311,-57.2100812780843,-10.));
#33882=CARTESIAN_POINT('Origin',(60.,-60.,-10.));
#33883=CARTESIAN_POINT('Ctrl Pts',(63.2235668665311,-57.2100812780843,-10.));
#33884=CARTESIAN_POINT('Ctrl Pts',(62.8262376065631,-56.7517870228408,-9.96602721186203));
#33885=CARTESIAN_POINT('Ctrl Pts',(62.3301929068535,-56.3786504290086,-9.93205442372406));
#33886=CARTESIAN_POINT('Ctrl Pts',(61.7790228098056,-56.125571221051,-9.89808163558608));
#33887=CARTESIAN_POINT('Ctrl Pts',(61.1467426998997,-55.8352489588686,-9.85910942295565));
#33888=CARTESIAN_POINT('Ctrl Pts',(60.441918927478,-55.7029192537276,-9.82013721032522));
#33889=CARTESIAN_POINT('Ctrl Pts',(59.7473945386634,-55.7441420953322,-9.78116499769479));
#33890=CARTESIAN_POINT('Ctrl Pts',(59.0528701498489,-55.7853649369367,-9.74219278506436));
#33891=CARTESIAN_POINT('Ctrl Pts',(58.3686451446415,-56.0001403252867,-9.70322057243393));
#33892=CARTESIAN_POINT('Ctrl Pts',(57.7751487508423,-56.3632201670063,-9.6642483598035));
#33893=CARTESIAN_POINT('Ctrl Pts',(57.1816523570431,-56.7263000087259,-9.62527614717308));
#33894=CARTESIAN_POINT('Ctrl Pts',(56.6788845746522,-57.2376843038151,-9.58630393454264));
#33895=CARTESIAN_POINT('Ctrl Pts',(56.325941879404,-57.8372637991282,-9.54733172191221));
#33896=CARTESIAN_POINT('Ctrl Pts',(55.9729991841559,-58.4368432944413,-9.50835950928178));
#33897=CARTESIAN_POINT('Ctrl Pts',(55.7698815760507,-59.1246179899783,-9.46938729665135));
#33898=CARTESIAN_POINT('Ctrl Pts',(55.7404649130753,-59.8197432519075,-9.43041508402093));
#33899=CARTESIAN_POINT('Ctrl Pts',(55.7110482500999,-60.5148685138366,-9.39144287139049));
#33900=CARTESIAN_POINT('Ctrl Pts',(55.8553325322544,-61.217344342158,-9.35247065876006));
#33901=CARTESIAN_POINT('Ctrl Pts',(56.156357704853,-61.8445988379219,-9.31349844612963));
#33902=CARTESIAN_POINT('Ctrl Pts',(56.4573828774516,-62.4718533336857,-9.2745262334992));
#33903=CARTESIAN_POINT('Ctrl Pts',(56.9151489404942,-63.023886496892,-9.23555402086877));
#33904=CARTESIAN_POINT('Ctrl Pts',(57.475848139259,-63.4358097682661,-9.19658180823834));
#33905=CARTESIAN_POINT('Ctrl Pts',(58.0365473380239,-63.8477330396401,-9.15760959560792));
#33906=CARTESIAN_POINT('Ctrl Pts',(58.700179672511,-64.1195464191819,-9.11863738297749));
#33907=CARTESIAN_POINT('Ctrl Pts',(59.3887387787435,-64.2192998103684,-9.07966517034706));
#33908=CARTESIAN_POINT('Ctrl Pts',(60.0772978849761,-64.3190532015549,-9.04069295771663));
#33909=CARTESIAN_POINT('Ctrl Pts',(60.7907837629541,-64.2467466043861,-9.0017207450862));
#33910=CARTESIAN_POINT('Ctrl Pts',(61.445330135215,-64.0108792149673,-8.96274853245577));
#33911=CARTESIAN_POINT('Ctrl Pts',(62.0998765074759,-63.7750118255484,-8.92377631982534));
#33912=CARTESIAN_POINT('Ctrl Pts',(62.6954833740198,-63.3755836438795,-8.88480410719491));
#33913=CARTESIAN_POINT('Ctrl Pts',(63.1621404033453,-62.859545295653,-8.84583189456448));
#33914=CARTESIAN_POINT('Ctrl Pts',(63.6287974326707,-62.3435069474265,-8.80685968193405));
#33915=CARTESIAN_POINT('Ctrl Pts',(63.9665046247778,-61.7108584326424,-8.76788746930362));
#33916=CARTESIAN_POINT('Ctrl Pts',(64.1355664404059,-61.0359639838401,-8.72891525667318));
#33917=CARTESIAN_POINT('Ctrl Pts',(64.2202977762693,-60.6977166510445,-8.70938294758577));
#33918=CARTESIAN_POINT('Ctrl Pts',(64.2626675966367,-60.3488576914975,-8.68985063849835));
#33919=CARTESIAN_POINT('Ctrl Pts',(64.2626697207193,-59.9999992453659,-8.67031832941094));
#33920=CARTESIAN_POINT('Origin',(60.,-60.,-13.3123464956316));
#33921=CARTESIAN_POINT('',(65.0994143001201,-59.9999919030003,-3.68765350436841));
#33922=CARTESIAN_POINT('',(65.0991104689079,-60.0001150498576,-3.56234649563159));
#33923=CARTESIAN_POINT('',(65.099,-60.,-13.3123464956316));
#33924=CARTESIAN_POINT('',(56.3967816198432,-56.392144916311,-3.));
#33925=CARTESIAN_POINT('Ctrl Pts',(65.0991104689079,-60.0001150498576,-3.56234649563159));
#33926=CARTESIAN_POINT('Ctrl Pts',(65.0984616565564,-59.3260858024822,-3.53078651427611));
#33927=CARTESIAN_POINT('Ctrl Pts',(64.7978132229132,-57.8191582297671,-3.4602543202902));
#33928=CARTESIAN_POINT('Ctrl Pts',(63.355584325901,-55.888083148428,-3.35074991367387));
#33929=CARTESIAN_POINT('Ctrl Pts',(61.0270447294087,-54.7929300306235,-3.23383327578258));
#33930=CARTESIAN_POINT('Ctrl Pts',(58.4567444358424,-54.9220255059251,-3.11691663789129));
#33931=CARTESIAN_POINT('Ctrl Pts',(56.9857510552447,-55.8039324061735,-3.03897221263043));
#33932=CARTESIAN_POINT('Ctrl Pts',(56.3967816198431,-56.3921449163111,-3.));
#33933=CARTESIAN_POINT('',(55.0736213077518,-58.683468118019,-3.));
#33934=CARTESIAN_POINT('Origin',(60.,-60.,-3.));
#33935=CARTESIAN_POINT('Ctrl Pts',(65.0994143001201,-59.9999919030003,-3.68765350436841));
#33936=CARTESIAN_POINT('Ctrl Pts',(65.0994150874834,-59.9917925604302,-3.68726952086906));
#33937=CARTESIAN_POINT('Ctrl Pts',(65.0974290916723,-59.151405440399,-3.64791332473929));
#33938=CARTESIAN_POINT('Ctrl Pts',(64.6714138259177,-57.4808672112921,-3.56958491597907));
#33939=CARTESIAN_POINT('Ctrl Pts',(62.9373243124707,-55.5795635648098,-3.45266827808779));
#33940=CARTESIAN_POINT('Ctrl Pts',(60.5127057471208,-54.7174568009332,-3.3357516401965));
#33941=CARTESIAN_POINT('Ctrl Pts',(57.9675484622588,-55.0972147578633,-3.21883500230521));
#33942=CARTESIAN_POINT('Ctrl Pts',(55.9886141307795,-56.5640444741926,-3.10691778890637));
#33943=CARTESIAN_POINT('Ctrl Pts',(55.2615313586432,-57.9827262758446,-3.03397278813797));
#33944=CARTESIAN_POINT('Ctrl Pts',(55.0736213077518,-58.683468118019,-3.));
#33945=CARTESIAN_POINT('Origin',(60.,-60.,-13.3123464956316));
#33946=CARTESIAN_POINT('',(65.0992594641877,-60.00006511688,-5.18765350436841));
#33947=CARTESIAN_POINT('',(65.098727976694,-60.000088054142,-5.06234649563159));
#33948=CARTESIAN_POINT('',(65.099,-60.,-13.3123464956316));
#33949=CARTESIAN_POINT('Ctrl Pts',(65.098727976694,-60.000088054142,-5.06234649563159));
#33950=CARTESIAN_POINT('Ctrl Pts',(65.0983788926485,-59.4677293602239,-5.0374252784717));
#33951=CARTESIAN_POINT('Ctrl Pts',(64.885463906226,-58.1025886458417,-4.97353184868138));
#33952=CARTESIAN_POINT('Ctrl Pts',(63.6865889957319,-56.1819888648126,-4.87066620626063));
#33953=CARTESIAN_POINT('Ctrl Pts',(61.4572741020296,-54.8966206991336,-4.75374956836934));
#33954=CARTESIAN_POINT('Ctrl Pts',(58.885371453618,-54.8109981947122,-4.63683293047805));
#33955=CARTESIAN_POINT('Ctrl Pts',(56.5755050285457,-55.9452536369063,-4.51991629258676));
#33956=CARTESIAN_POINT('Ctrl Pts',(55.0706997941323,-58.0327345420765,-4.40299965469547));
#33957=CARTESIAN_POINT('Ctrl Pts',(54.7247181776535,-60.582698043192,-4.28608301680418));
#33958=CARTESIAN_POINT('Ctrl Pts',(55.6188973116942,-62.9956754944399,-4.16916637891289));
#33959=CARTESIAN_POINT('Ctrl Pts',(57.5430244076546,-64.704403039722,-4.0522497410216));
#33960=CARTESIAN_POINT('Ctrl Pts',(60.0447608860831,-65.3071770970488,-3.93533310313031));
#33961=CARTESIAN_POINT('Ctrl Pts',(62.5359710979979,-64.6622934589222,-3.81841646523902));
#33962=CARTESIAN_POINT('Ctrl Pts',(64.4310101226481,-62.9213544069835,-3.70149982734774));
#33963=CARTESIAN_POINT('Ctrl Pts',(65.0540042410307,-61.148967957511,-3.61614317081192));
#33964=CARTESIAN_POINT('Ctrl Pts',(65.099262850088,-60.158418713328,-3.56975872690654));
#33965=CARTESIAN_POINT('Ctrl Pts',(65.0991104689079,-60.0001150498576,-3.56234649563159));
#33966=CARTESIAN_POINT('Ctrl Pts',(65.0992594641877,-60.00006511688,-5.18765350436841));
#33967=CARTESIAN_POINT('Ctrl Pts',(65.0986258244756,-59.3013381719494,-5.15493607243422));
#33968=CARTESIAN_POINT('Ctrl Pts',(64.7810045336314,-57.7698535833796,-5.0832464278696));
#33969=CARTESIAN_POINT('Ctrl Pts',(63.2955109178121,-55.8396721751708,-4.97258457067455));
#33970=CARTESIAN_POINT('Ctrl Pts',(60.9510823423798,-54.7785639854422,-4.85566793278326));
#33971=CARTESIAN_POINT('Ctrl Pts',(58.3831733906512,-54.9449006048999,-4.73875129489197));
#33972=CARTESIAN_POINT('Ctrl Pts',(56.1953121953125,-56.2996615164319,-4.62183465700068));
#33973=CARTESIAN_POINT('Ctrl Pts',(54.9019142627768,-58.5243188117934,-4.50491801910939));
#33974=CARTESIAN_POINT('Ctrl Pts',(54.8070090534039,-61.0958980757912,-4.3880013812181));
#33975=CARTESIAN_POINT('Ctrl Pts',(55.932923519751,-63.4098412167327,-4.27108474332681));
#33976=CARTESIAN_POINT('Ctrl Pts',(58.0149603071344,-64.9221696503736,-4.15416810543553));
#33977=CARTESIAN_POINT('Ctrl Pts',(60.5636590522025,-65.2773499477182,-4.03725146754423));
#33978=CARTESIAN_POINT('Ctrl Pts',(62.9798472271926,-64.3918839378294,-3.92033482965295));
#33979=CARTESIAN_POINT('Ctrl Pts',(64.6898720416353,-62.4802336033169,-3.803802175261));
#33980=CARTESIAN_POINT('Ctrl Pts',(65.0993351744413,-60.8239807211494,-3.72624173349949));
#33981=CARTESIAN_POINT('Ctrl Pts',(65.0994143001201,-59.9999919030003,-3.68765350436841));
#33982=CARTESIAN_POINT('Origin',(60.,-60.,-13.3123464956316));
#33983=CARTESIAN_POINT('',(65.0984551471835,-60.0005764959704,-6.68765350436841));
#33984=CARTESIAN_POINT('',(65.0986380202759,-59.9935550909786,-6.56234649563159));
#33985=CARTESIAN_POINT('',(65.099,-60.,-13.3123464956316));
#33986=CARTESIAN_POINT('Ctrl Pts',(65.0986380202759,-59.9935550909786,-6.56234649563159));
#33987=CARTESIAN_POINT('Ctrl Pts',(65.1022613065284,-59.6027949249183,-6.54406404266729));
#33988=CARTESIAN_POINT('Ctrl Pts',(64.8866737284852,-57.5511808779631,-6.44783716444213));
#33989=CARTESIAN_POINT('Ctrl Pts',(62.7388651753224,-55.1183365899423,-6.31263807358654));
#33990=CARTESIAN_POINT('Ctrl Pts',(59.3187592643186,-54.7414778160817,-6.15674922306481));
#33991=CARTESIAN_POINT('Ctrl Pts',(56.9266332065095,-55.6714869946495,-6.03983258517353));
#33992=CARTESIAN_POINT('Ctrl Pts',(55.2511528738565,-57.6299781348164,-5.92291594728223));
#33993=CARTESIAN_POINT('Ctrl Pts',(54.6947970697628,-60.1405542822466,-5.80599930939095));
#33994=CARTESIAN_POINT('Ctrl Pts',(55.3843760570615,-62.6204343466251,-5.68908267149966));
#33995=CARTESIAN_POINT('Ctrl Pts',(57.159620885591,-64.483190888477,-5.57216603360837));
#33996=CARTESIAN_POINT('Ctrl Pts',(59.6023371070298,-65.292502635446,-5.45524939571708));
#33997=CARTESIAN_POINT('Ctrl Pts',(62.1386646734039,-64.8573722208712,-5.33833275782579));
#33998=CARTESIAN_POINT('Ctrl Pts',(64.1721578713598,-63.2804354544672,-5.2214161199345));
#33999=CARTESIAN_POINT('Ctrl Pts',(65.0004645952953,-61.4327780814141,-5.1294206992031));
#34000=CARTESIAN_POINT('Ctrl Pts',(65.0989247960673,-60.3002407131776,-5.07639749110213));
#34001=CARTESIAN_POINT('Ctrl Pts',(65.098727976694,-60.000088054142,-5.06234649563159));
#34002=CARTESIAN_POINT('Ctrl Pts',(65.0984551471835,-60.0005764959704,-6.68765350436841));
#34003=CARTESIAN_POINT('Ctrl Pts',(65.0974568125024,-59.4443120828723,-6.66157483662981));
#34004=CARTESIAN_POINT('Ctrl Pts',(64.8688855876321,-58.0563258472263,-6.59652395626078));
#34005=CARTESIAN_POINT('Ctrl Pts',(63.1773262290866,-55.3916806820179,-6.45352865063089));
#34006=CARTESIAN_POINT('Ctrl Pts',(58.6661395049216,-54.1559238915272,-6.25866758747873));
#34007=CARTESIAN_POINT('Ctrl Pts',(54.3971988313774,-57.8690311013926,-6.02483431169616));
#34008=CARTESIAN_POINT('Ctrl Pts',(54.9957837258839,-62.5079530267534,-5.82997324854401));
#34009=CARTESIAN_POINT('Ctrl Pts',(57.6170694121072,-64.7368553395382,-5.67408439802229));
#34010=CARTESIAN_POINT('Ctrl Pts',(60.1194267752203,-65.3072914717773,-5.557167760131));
#34011=CARTESIAN_POINT('Ctrl Pts',(62.6046736799591,-64.6243084010734,-5.44025112223971));
#34012=CARTESIAN_POINT('Ctrl Pts',(64.4724887605417,-62.8568826882213,-5.32333448434842));
#34013=CARTESIAN_POINT('Ctrl Pts',(65.0621164699687,-61.0994766787787,-5.23913527839132));
#34014=CARTESIAN_POINT('Ctrl Pts',(65.0993806007563,-60.1336447882883,-5.19390828506465));
#34015=CARTESIAN_POINT('Ctrl Pts',(65.0992594641877,-60.00006511688,-5.18765350436841));
#34016=CARTESIAN_POINT('Origin',(60.,-60.,-13.3123464956316));
#34017=CARTESIAN_POINT('',(65.0986049509612,-59.9999990973777,-8.18765350436841));
#34018=CARTESIAN_POINT('',(65.0988481317111,-59.9998830050765,-8.06234649563159));
#34019=CARTESIAN_POINT('',(65.099,-60.,-13.3123464956316));
#34020=CARTESIAN_POINT('Ctrl Pts',(65.0988481317111,-59.9998830050765,-8.06234649563159));
#34021=CARTESIAN_POINT('Ctrl Pts',(65.0990615391883,-59.7511708601392,-8.05070280686288));
#34022=CARTESIAN_POINT('Ctrl Pts',(65.0213100778608,-58.6701368189858,-8.00008690546373));
#34023=CARTESIAN_POINT('Ctrl Pts',(64.2694756589632,-56.8472981310306,-7.91049879143416));
#34024=CARTESIAN_POINT('Ctrl Pts',(62.2845938482857,-55.2094519237375,-7.79358215354287));
#34025=CARTESIAN_POINT('Ctrl Pts',(59.7626220066562,-54.6980752792535,-7.67666551565158));
#34026=CARTESIAN_POINT('Ctrl Pts',(57.2964708372155,-55.4325509730806,-7.55974887776029));
#34027=CARTESIAN_POINT('Ctrl Pts',(55.4658552325379,-57.2420179723235,-7.442832239869));
#34028=CARTESIAN_POINT('Ctrl Pts',(54.701239676989,-59.6971936126827,-7.32591560197771));
#34029=CARTESIAN_POINT('Ctrl Pts',(55.1821426669066,-62.2293180577881,-7.20899896408642));
#34030=CARTESIAN_POINT('Ctrl Pts',(56.7959916580377,-64.2249822536134,-7.09208232619513));
#34031=CARTESIAN_POINT('Ctrl Pts',(59.9512920111792,-65.5972893108641,-6.93619347567341));
#34032=CARTESIAN_POINT('Ctrl Pts',(63.964474637114,-64.2336347183845,-6.75961486548557));
#34033=CARTESIAN_POINT('Ctrl Pts',(65.0868139830726,-61.2687407702531,-6.62200846792815));
#34034=CARTESIAN_POINT('Ctrl Pts',(65.0986380202759,-59.9935550909786,-6.56234649563159));
#34035=CARTESIAN_POINT('Ctrl Pts',(65.0986049509612,-59.9999990973777,-8.18765350436841));
#34036=CARTESIAN_POINT('Ctrl Pts',(65.0986074795697,-59.5847014805283,-8.1682136008254));
#34037=CARTESIAN_POINT('Ctrl Pts',(64.9477827615392,-58.3368363840766,-8.10980148465195));
#34038=CARTESIAN_POINT('Ctrl Pts',(63.9406234799139,-56.4447764036095,-8.01241715584808));
#34039=CARTESIAN_POINT('Ctrl Pts',(61.8050635175092,-55.0090188089158,-7.89550051795678));
#34040=CARTESIAN_POINT('Ctrl Pts',(59.2451498180026,-54.7465902155457,-7.7785838800655));
#34041=CARTESIAN_POINT('Ctrl Pts',(56.8627001404056,-55.7191702005741,-7.66166724217421));
#34042=CARTESIAN_POINT('Ctrl Pts',(55.217779590162,-57.6981472392852,-7.54475060428292));
#34043=CARTESIAN_POINT('Ctrl Pts',(54.6971392178688,-60.21821824206,-7.42783396639163));
#34044=CARTESIAN_POINT('Ctrl Pts',(55.4230712207726,-62.6870881580822,-7.31091732850034));
#34045=CARTESIAN_POINT('Ctrl Pts',(57.2251428783372,-64.5240383042407,-7.19400069060906));
#34046=CARTESIAN_POINT('Ctrl Pts',(59.6792195378112,-65.2979014573777,-7.07708405271776));
#34047=CARTESIAN_POINT('Ctrl Pts',(62.2094281655486,-64.8252835759928,-6.96016741482648));
#34048=CARTESIAN_POINT('Ctrl Pts',(64.2186727163164,-63.2204586132884,-6.84325077693518));
#34049=CARTESIAN_POINT('Ctrl Pts',(65.0118135613323,-61.3817369404773,-6.7524128067825));
#34050=CARTESIAN_POINT('Ctrl Pts',(65.09894873348,-60.2755989876827,-6.70054704926024));
#34051=CARTESIAN_POINT('Ctrl Pts',(65.0984551471835,-60.0005764959704,-6.68765350436841));
#34052=CARTESIAN_POINT('Origin',(60.,-60.,-13.3123464956316));
#34053=CARTESIAN_POINT('',(65.0987893869763,-59.9998803238954,-9.68765350436841));
#34054=CARTESIAN_POINT('',(65.0992547697948,-59.9999087515425,-9.56234649563159));
#34055=CARTESIAN_POINT('',(65.099,-60.,-13.3123464956316));
#34056=CARTESIAN_POINT('',(61.322884965569,-64.9244061944433,-10.));
#34057=CARTESIAN_POINT('Ctrl Pts',(61.322884965569,-64.9244061944433,-10.));
#34058=CARTESIAN_POINT('Ctrl Pts',(62.1267766598728,-64.7084499564018,-9.96102778736957));
#34059=CARTESIAN_POINT('Ctrl Pts',(63.6260271020141,-63.8754856296126,-9.88308336210871));
#34060=CARTESIAN_POINT('Ctrl Pts',(64.8700259293115,-61.9507383889051,-9.77896786356485));
#34061=CARTESIAN_POINT('Ctrl Pts',(65.0983672591983,-60.5589068688162,-9.71382457765142));
#34062=CARTESIAN_POINT('Ctrl Pts',(65.0987893869763,-59.9998803238954,-9.68765350436841));
#34063=CARTESIAN_POINT('',(58.6769607093948,-64.9246350255102,-10.));
#34064=CARTESIAN_POINT('Origin',(60.,-60.,-10.));
#34065=CARTESIAN_POINT('Ctrl Pts',(58.6769607093948,-64.9246350255102,-10.));
#34066=CARTESIAN_POINT('Ctrl Pts',(59.3777759715939,-65.1122710698436,-9.96602721186203));
#34067=CARTESIAN_POINT('Ctrl Pts',(60.9699318324407,-65.1919398158278,-9.89308221109363));
#34068=CARTESIAN_POINT('Ctrl Pts',(63.2297107943118,-64.2115472768226,-9.78116499769479));
#34069=CARTESIAN_POINT('Ctrl Pts',(64.7626148130399,-62.283482461386,-9.66925328437663));
#34070=CARTESIAN_POINT('Ctrl Pts',(65.0986449091995,-60.7252905354434,-9.5963137836889));
#34071=CARTESIAN_POINT('Ctrl Pts',(65.0992547697949,-59.9999087515425,-9.56234649563159));
#34072=CARTESIAN_POINT('Origin',(-60.,-60.,-6.));
#34073=CARTESIAN_POINT('',(-55.7372274017113,-60.0000736188739,-4.57968167058906));
#34074=CARTESIAN_POINT('',(-55.7366536901661,-59.9999932304475,-4.17031832941095));
#34075=CARTESIAN_POINT('',(-55.737,-60.,-6.));
#34076=CARTESIAN_POINT('',(-59.1956105045055,-64.1864216867795,-3.));
#34077=CARTESIAN_POINT('Ctrl Pts',(-55.7366536901661,-59.9999932304475,
-4.17031832941095));
#34078=CARTESIAN_POINT('Ctrl Pts',(-55.7366530318933,-59.9931382006682,
-4.1699343459116));
#34079=CARTESIAN_POINT('Ctrl Pts',(-55.7366692316342,-59.9862831740153,
-4.16955036241225));
#34080=CARTESIAN_POINT('Ctrl Pts',(-55.7367023085573,-59.9794282288035,
-4.1691663789129));
#34081=CARTESIAN_POINT('Ctrl Pts',(-55.7400594342771,-59.2836890035115,
-4.13019416628247));
#34082=CARTESIAN_POINT('Ctrl Pts',(-55.9172706620175,-58.5887887151182,
-4.09122195365204));
#34083=CARTESIAN_POINT('Ctrl Pts',(-56.2475061214605,-57.9764089332034,
-4.05224974102161));
#34084=CARTESIAN_POINT('Ctrl Pts',(-56.5777415809036,-57.3640291512886,
-4.01327752839118));
#34085=CARTESIAN_POINT('Ctrl Pts',(-57.0610012720493,-56.8341698758524,
-3.97430531576075));
#34086=CARTESIAN_POINT('Ctrl Pts',(-57.6404800019574,-56.4491133816137,
-3.93533310313032));
#34087=CARTESIAN_POINT('Ctrl Pts',(-58.2199587318654,-56.064056887375,-3.89636089049989));
#34088=CARTESIAN_POINT('Ctrl Pts',(-58.8956565005358,-55.8238031743338,
-3.85738867786946));
#34089=CARTESIAN_POINT('Ctrl Pts',(-59.5881502622955,-55.7565921866708,
-3.81841646523903));
#34090=CARTESIAN_POINT('Ctrl Pts',(-60.2806440240553,-55.6893811990077,
-3.7794442526086));
#34091=CARTESIAN_POINT('Ctrl Pts',(-60.9899337789045,-55.7952129367229,
-3.74047203997817));
#34092=CARTESIAN_POINT('Ctrl Pts',(-61.632643243836,-56.0616486298365,-3.70149982734774));
#34093=CARTESIAN_POINT('Ctrl Pts',(-62.2753527087675,-56.32808432295,-3.66252761471731));
#34094=CARTESIAN_POINT('Ctrl Pts',(-62.8514818837812,-56.7551239714621,
-3.62355540208688));
#34095=CARTESIAN_POINT('Ctrl Pts',(-63.2933169034021,-57.2925688095136,
-3.58458318945645));
#34096=CARTESIAN_POINT('Ctrl Pts',(-63.7351519230229,-57.8300136475652,
-3.54561097682602));
#34097=CARTESIAN_POINT('Ctrl Pts',(-64.0426927872508,-58.4778636751564,
-3.50663876419559));
#34098=CARTESIAN_POINT('Ctrl Pts',(-64.1797749238076,-59.1599729097974,
-3.46766655156516));
#34099=CARTESIAN_POINT('Ctrl Pts',(-64.3168570603643,-59.8420821444384,
-3.42869433893473));
#34100=CARTESIAN_POINT('Ctrl Pts',(-64.2834804692498,-60.5584505861292,
-3.3897221263043));
#34101=CARTESIAN_POINT('Ctrl Pts',(-64.0836009345363,-61.224859865863,-3.35074991367387));
#34102=CARTESIAN_POINT('Ctrl Pts',(-63.8837213998229,-61.8912691455967,
-3.31177770104344));
#34103=CARTESIAN_POINT('Ctrl Pts',(-63.5173389215105,-62.5077192633734,
-3.27280548841301));
#34104=CARTESIAN_POINT('Ctrl Pts',(-63.0274513378467,-63.001770094789,-3.23383327578258));
#34105=CARTESIAN_POINT('Ctrl Pts',(-62.537563754183,-63.4958209262046,-3.19486106315215));
#34106=CARTESIAN_POINT('Ctrl Pts',(-61.9241710651678,-63.8674724712591,
-3.15588885052172));
#34107=CARTESIAN_POINT('Ctrl Pts',(-61.2595373436356,-64.0729510882669,
-3.11691663789129));
#34108=CARTESIAN_POINT('Ctrl Pts',(-60.5949036221034,-64.2784297052747,
-3.07794442526086));
#34109=CARTESIAN_POINT('Ctrl Pts',(-59.8790288680541,-64.3177353942359,
-3.03897221263043));
#34110=CARTESIAN_POINT('Ctrl Pts',(-59.1956105045054,-64.1864216867795,
-3.));
#34111=CARTESIAN_POINT('',(-55.9720760639888,-58.6032685615972,-3.));
#34112=CARTESIAN_POINT('Origin',(-60.,-60.,-3.));
#34113=CARTESIAN_POINT('',(-55.7369076166092,-60.0000961895604,-3.07968167058906));
#34114=CARTESIAN_POINT('Ctrl Pts',(-55.9720760639888,-58.6032685615972,
-3.));
#34115=CARTESIAN_POINT('Ctrl Pts',(-55.8170962955876,-59.0514416515873,
-3.02656055686302));
#34116=CARTESIAN_POINT('Ctrl Pts',(-55.737364127205,-59.5258438267831,-3.05312111372604));
#34117=CARTESIAN_POINT('Ctrl Pts',(-55.7369076166092,-60.0000961895604,
-3.07968167058906));
#34118=CARTESIAN_POINT('',(-55.737,-60.,-2.));
#34119=CARTESIAN_POINT('',(-55.737,-60.,-6.));
#34120=CARTESIAN_POINT('Origin',(-60.,-60.,-2.));
#34121=CARTESIAN_POINT('Ctrl Pts',(-55.7369076166092,-60.0000961895604,
-3.07968167058906));
#34122=CARTESIAN_POINT('Ctrl Pts',(-55.7367802185982,-60.1324453798928,
-3.08709390186401));
#34123=CARTESIAN_POINT('Ctrl Pts',(-55.7428267750975,-60.2647829028978,
-3.09450613313897));
#34124=CARTESIAN_POINT('Ctrl Pts',(-55.7551348310466,-60.396535445299,-3.10191836441392));
#34125=CARTESIAN_POINT('Ctrl Pts',(-55.8198484315432,-61.0892672161508,
-3.14089057704435));
#34126=CARTESIAN_POINT('Ctrl Pts',(-56.0576594342791,-61.7658273617105,
-3.17986278967478));
#34127=CARTESIAN_POINT('Ctrl Pts',(-56.4406216586579,-62.3466917067985,
-3.21883500230521));
#34128=CARTESIAN_POINT('Ctrl Pts',(-56.8235838830368,-62.9275560518864,
-3.25780721493564));
#34129=CARTESIAN_POINT('Ctrl Pts',(-57.3516973290586,-63.4127245965028,
-3.29677942756607));
#34130=CARTESIAN_POINT('Ctrl Pts',(-57.9628818942373,-63.7451676306387,
-3.3357516401965));
#34131=CARTESIAN_POINT('Ctrl Pts',(-58.574066459416,-64.0776106647747,-3.37472385282693));
#34132=CARTESIAN_POINT('Ctrl Pts',(-59.2683221437516,-64.2573281884304,
-3.41369606545736));
#34133=CARTESIAN_POINT('Ctrl Pts',(-59.9640445684965,-64.2631957814501,
-3.45266827808779));
#34134=CARTESIAN_POINT('Ctrl Pts',(-60.6597669932415,-64.2690633744698,
-3.49164049071822));
#34135=CARTESIAN_POINT('Ctrl Pts',(-61.3569561583957,-64.1010810368534,
-3.53061270334865));
#34136=CARTESIAN_POINT('Ctrl Pts',(-61.9736606271436,-63.7789939810841,
-3.56958491597907));
#34137=CARTESIAN_POINT('Ctrl Pts',(-62.5903650958916,-63.4569069253149,
-3.60855712860951));
#34138=CARTESIAN_POINT('Ctrl Pts',(-63.1265848682333,-62.9807151513927,
-3.64752934123993));
#34139=CARTESIAN_POINT('Ctrl Pts',(-63.5192906120051,-62.4063924575338,
-3.68650155387036));
#34140=CARTESIAN_POINT('Ctrl Pts',(-63.9119963557769,-61.8320697636749,
-3.72547376650079));
#34141=CARTESIAN_POINT('Ctrl Pts',(-64.1611880709788,-61.1596161498792,
-3.76444597913122));
#34142=CARTESIAN_POINT('Ctrl Pts',(-64.2375744875774,-60.4680747563421,
-3.80341819176165));
#34143=CARTESIAN_POINT('Ctrl Pts',(-64.313960904176,-59.776533362805,-3.84239040439208));
#34144=CARTESIAN_POINT('Ctrl Pts',(-64.2175420221713,-59.0659041895265,
-3.88136261702251));
#34145=CARTESIAN_POINT('Ctrl Pts',(-63.9596514427128,-58.4197178258067,
-3.92033482965294));
#34146=CARTESIAN_POINT('Ctrl Pts',(-63.7017608632543,-57.773531462087,-3.95930704228337));
#34147=CARTESIAN_POINT('Ctrl Pts',(-63.282398586342,-57.1917879079259,-3.9982792549138));
#34148=CARTESIAN_POINT('Ctrl Pts',(-62.7508582394783,-56.7428677888888,
-4.03725146754424));
#34149=CARTESIAN_POINT('Ctrl Pts',(-62.2193178926146,-56.2939476698518,
-4.07622368017466));
#34150=CARTESIAN_POINT('Ctrl Pts',(-61.5755994757997,-55.9778509859388,
-4.1151958928051));
#34151=CARTESIAN_POINT('Ctrl Pts',(-60.895368656883,-55.8317333733196,-4.15416810543553));
#34152=CARTESIAN_POINT('Ctrl Pts',(-60.2151378379662,-55.6856157607004,
-4.19314031806596));
#34153=CARTESIAN_POINT('Ctrl Pts',(-59.4983946169477,-55.7094772193751,
-4.23211253069638));
#34154=CARTESIAN_POINT('Ctrl Pts',(-58.8293879329443,-55.9005124963388,
-4.27108474332681));
#34155=CARTESIAN_POINT('Ctrl Pts',(-58.1603812489408,-56.0915477733025,
-4.31005695595724));
#34156=CARTESIAN_POINT('Ctrl Pts',(-57.5391111019523,-56.4497568685552,
-4.34902916858767));
#34157=CARTESIAN_POINT('Ctrl Pts',(-57.0386049049034,-56.9330352993155,
-4.3880013812181));
#34158=CARTESIAN_POINT('Ctrl Pts',(-56.5380987078546,-57.4163137300757,
-4.42697359384853));
#34159=CARTESIAN_POINT('Ctrl Pts',(-56.1583564607454,-58.0246614963435,
-4.46594580647896));
#34160=CARTESIAN_POINT('Ctrl Pts',(-55.944013587813,-58.6865684993411,-4.50491801910939));
#34161=CARTESIAN_POINT('Ctrl Pts',(-55.8069496409009,-59.1098323339553,
-4.52983923626928));
#34162=CARTESIAN_POINT('Ctrl Pts',(-55.7375192518995,-59.5549971083828,
-4.55476045342917));
#34163=CARTESIAN_POINT('Ctrl Pts',(-55.7372274017113,-60.0000736188739,
-4.57968167058906));
#34164=CARTESIAN_POINT('Origin',(-60.,-60.,-6.));
#34165=CARTESIAN_POINT('',(-55.7373026458209,-59.9946120201631,-6.07968167058906));
#34166=CARTESIAN_POINT('',(-55.7367829988534,-60.0000543459286,-5.67031832941095));
#34167=CARTESIAN_POINT('',(-55.737,-60.,-6.));
#34168=CARTESIAN_POINT('Ctrl Pts',(-55.7367829988534,-60.0000543459286,
-5.67031832941095));
#34169=CARTESIAN_POINT('Ctrl Pts',(-55.7373127458066,-59.4158862842898,
-5.63760089747676));
#34170=CARTESIAN_POINT('Ctrl Pts',(-55.8585017631583,-58.8315462413849,
-5.60488346554257));
#34171=CARTESIAN_POINT('Ctrl Pts',(-56.091956403473,-58.296147811699,-5.57216603360838));
#34172=CARTESIAN_POINT('Ctrl Pts',(-56.370041917648,-57.658394167535,-5.53319382097794));
#34173=CARTESIAN_POINT('Ctrl Pts',(-56.8074210959631,-57.0900837660379,
-5.49422160834752));
#34174=CARTESIAN_POINT('Ctrl Pts',(-57.3527858412086,-56.6580726588936,
-5.45524939571708));
#34175=CARTESIAN_POINT('Ctrl Pts',(-57.8981505864541,-56.2260615517493,
-5.41627718308665));
#34176=CARTESIAN_POINT('Ctrl Pts',(-58.5515008986299,-55.9303497389577,
-5.37730497045622));
#34177=CARTESIAN_POINT('Ctrl Pts',(-59.235991157749,-55.8056713421077,-5.33833275782579));
#34178=CARTESIAN_POINT('Ctrl Pts',(-59.9204814168682,-55.6809929452577,
-5.29936054519536));
#34179=CARTESIAN_POINT('Ctrl Pts',(-60.6361116229307,-55.7273479643494,
-5.26038833256493));
#34180=CARTESIAN_POINT('Ctrl Pts',(-61.2987855987603,-55.9392992796723,
-5.2214161199345));
#34181=CARTESIAN_POINT('Ctrl Pts',(-61.9614595745898,-56.1512505949953,
-5.18244390730407));
#34182=CARTESIAN_POINT('Ctrl Pts',(-62.5711773201864,-56.5287982065494,
-5.14347169467364));
#34183=CARTESIAN_POINT('Ctrl Pts',(-63.0562596091439,-57.0275580828228,
-5.10449948204321));
#34184=CARTESIAN_POINT('Ctrl Pts',(-63.5413418981015,-57.5263179590961,
-5.06552726941278));
#34185=CARTESIAN_POINT('Ctrl Pts',(-63.90178873042,-58.1462901000886,-5.02655505678236));
#34186=CARTESIAN_POINT('Ctrl Pts',(-64.0952363394269,-58.8146027140363,
-4.98758284415193));
#34187=CARTESIAN_POINT('Ctrl Pts',(-64.2886839484338,-59.4829153279839,
-4.9486106315215));
#34188=CARTESIAN_POINT('Ctrl Pts',(-64.315132334129,-60.1995684148867,-4.90963841889107));
#34189=CARTESIAN_POINT('Ctrl Pts',(-64.171470427582,-60.880322213531,-4.87066620626064));
#34190=CARTESIAN_POINT('Ctrl Pts',(-64.0278085210349,-61.5610760121754,
-4.83169399363021));
#34191=CARTESIAN_POINT('Ctrl Pts',(-63.7140363222456,-62.2059305225613,
-4.79272178099978));
#34192=CARTESIAN_POINT('Ctrl Pts',(-63.2670370412591,-62.7390872025879,
-4.75374956836935));
#34193=CARTESIAN_POINT('Ctrl Pts',(-62.8200377602726,-63.2722438826145,
-4.71477735573892));
#34194=CARTESIAN_POINT('Ctrl Pts',(-62.2398113970889,-63.6937027322818,
-4.67580514310849));
#34195=CARTESIAN_POINT('Ctrl Pts',(-61.5945598683159,-63.9539233508557,
-4.63683293047806));
#34196=CARTESIAN_POINT('Ctrl Pts',(-60.949308339543,-64.2141439694296,-4.59786071784763));
#34197=CARTESIAN_POINT('Ctrl Pts',(-60.2390316451808,-64.3131263569101,
-4.5588885052172));
#34198=CARTESIAN_POINT('Ctrl Pts',(-59.5472191125019,-64.2392357914097,
-4.51991629258677));
#34199=CARTESIAN_POINT('Ctrl Pts',(-58.855406579823,-64.1653452259092,-4.48094407995634));
#34200=CARTESIAN_POINT('Ctrl Pts',(-58.1820582088273,-63.9185817074278,
-4.44197186732591));
#34201=CARTESIAN_POINT('Ctrl Pts',(-57.6063222395974,-63.5279508797756,
-4.40299965469548));
#34202=CARTESIAN_POINT('Ctrl Pts',(-57.0305862703675,-63.1373200521234,
-4.36402744206505));
#34203=CARTESIAN_POINT('Ctrl Pts',(-56.5524627029033,-62.6028219153003,
-4.32505522943462));
#34204=CARTESIAN_POINT('Ctrl Pts',(-56.2281524310208,-61.9872837657933,
-4.28608301680419));
#34205=CARTESIAN_POINT('Ctrl Pts',(-55.9070375074305,-61.3778103602842,
-4.24749478767311));
#34206=CARTESIAN_POINT('Ctrl Pts',(-55.7367198429653,-60.6888860090946,
-4.20890655854203));
#34207=CARTESIAN_POINT('Ctrl Pts',(-55.7366536901661,-59.9999932304475,
-4.17031832941095));
#34208=CARTESIAN_POINT('Ctrl Pts',(-55.7372274017113,-60.0000736188739,
-4.57968167058906));
#34209=CARTESIAN_POINT('Ctrl Pts',(-55.7370628517358,-60.2510151356077,
-4.5937326660596));
#34210=CARTESIAN_POINT('Ctrl Pts',(-55.7588766922514,-60.5019285941948,
-4.60778366153014));
#34211=CARTESIAN_POINT('Ctrl Pts',(-55.8029386627415,-60.7488728439853,
-4.62183465700068));
#34212=CARTESIAN_POINT('Ctrl Pts',(-55.9251501093579,-61.4338039459045,
-4.66080686963111));
#34213=CARTESIAN_POINT('Ctrl Pts',(-56.2185165013463,-62.0881999100153,
-4.69977908226154));
#34214=CARTESIAN_POINT('Ctrl Pts',(-56.6485487731059,-62.6351299192171,
-4.73875129489197));
#34215=CARTESIAN_POINT('Ctrl Pts',(-57.0785810448654,-63.182059928419,-4.7777235075224));
#34216=CARTESIAN_POINT('Ctrl Pts',(-57.6452791963962,-63.6215239827118,
-4.81669572015283));
#34217=CARTESIAN_POINT('Ctrl Pts',(-58.2820428086401,-63.9018875269744,
-4.85566793278326));
#34218=CARTESIAN_POINT('Ctrl Pts',(-58.9188064208841,-64.1822510712369,
-4.89464014541369));
#34219=CARTESIAN_POINT('Ctrl Pts',(-59.6256354938411,-64.3035141054693,
-4.93361235804412));
#34220=CARTESIAN_POINT('Ctrl Pts',(-60.3194206777223,-64.2513752968827,
-4.97258457067455));
#34221=CARTESIAN_POINT('Ctrl Pts',(-61.0132058616034,-64.1992364882962,
-5.01155678330498));
#34222=CARTESIAN_POINT('Ctrl Pts',(-61.6939471564087,-63.9736958368907,
-5.05052899593541));
#34223=CARTESIAN_POINT('Ctrl Pts',(-62.2816822612956,-63.6013670203114,
-5.08950120856584));
#34224=CARTESIAN_POINT('Ctrl Pts',(-62.8694173661825,-63.2290382037321,
-5.12847342119627));
#34225=CARTESIAN_POINT('Ctrl Pts',(-63.3641462811511,-62.709921221979,-5.1674456338267));
#34226=CARTESIAN_POINT('Ctrl Pts',(-63.707597429373,-62.1048137232406,-5.20641784645713));
#34227=CARTESIAN_POINT('Ctrl Pts',(-64.051048577595,-61.4997062245023,-5.24539005908756));
#34228=CARTESIAN_POINT('Ctrl Pts',(-64.2432219590703,-60.8086082087788,
-5.28436227171798));
#34229=CARTESIAN_POINT('Ctrl Pts',(-64.2617853890068,-60.1132327305904,
-5.32333448434842));
#34230=CARTESIAN_POINT('Ctrl Pts',(-64.2803488189434,-59.4178572524019,
-5.36230669697885));
#34231=CARTESIAN_POINT('Ctrl Pts',(-64.125302297341,-58.7182043117486,-5.40127890960928));
#34232=CARTESIAN_POINT('Ctrl Pts',(-63.8143159491228,-58.0954799012611,
-5.44025112223971));
#34233=CARTESIAN_POINT('Ctrl Pts',(-63.5033296009046,-57.4727554907737,
-5.47922333487014));
#34234=CARTESIAN_POINT('Ctrl Pts',(-63.0364034260706,-56.9269596104521,
-5.51819554750057));
#34235=CARTESIAN_POINT('Ctrl Pts',(-62.4696187992193,-56.5244726304014,
-5.557167760131));
#34236=CARTESIAN_POINT('Ctrl Pts',(-61.902834172368,-56.1219856503507,-5.59613997276143));
#34237=CARTESIAN_POINT('Ctrl Pts',(-61.2361910934994,-55.862807570571,-5.63511218539186));
#34238=CARTESIAN_POINT('Ctrl Pts',(-60.5454488737994,-55.7726030381307,
-5.67408439802229));
#34239=CARTESIAN_POINT('Ctrl Pts',(-59.8547066540995,-55.6823985056904,
-5.71305661065272));
#34240=CARTESIAN_POINT('Ctrl Pts',(-59.1398652935682,-55.7611675205897,
-5.75202882328315));
#34241=CARTESIAN_POINT('Ctrl Pts',(-58.4907658812686,-56.0091161201719,
-5.79100103591358));
#34242=CARTESIAN_POINT('Ctrl Pts',(-57.1925670566693,-56.5050133193363,
-5.86894546117443));
#34243=CARTESIAN_POINT('Ctrl Pts',(-56.1573360249965,-57.6776288572327,
-5.9468898864353));
#34244=CARTESIAN_POINT('Ctrl Pts',(-55.8423908354356,-59.0258082047619,
-6.02483431169616));
#34245=CARTESIAN_POINT('Ctrl Pts',(-55.7685180652509,-59.3420338415045,
-6.04311676466046));
#34246=CARTESIAN_POINT('Ctrl Pts',(-55.7342734351814,-59.667918514758,-6.06139921762476));
#34247=CARTESIAN_POINT('Ctrl Pts',(-55.7373026458209,-59.9946120201631,
-6.07968167058906));
#34248=CARTESIAN_POINT('Origin',(-60.,-60.,-6.));
#34249=CARTESIAN_POINT('',(-55.7371269462215,-59.9999021904687,-7.57968167058906));
#34250=CARTESIAN_POINT('',(-55.7374565106948,-60.0004827185225,-7.17031832941094));
#34251=CARTESIAN_POINT('',(-55.737,-60.,-6.));
#34252=CARTESIAN_POINT('Ctrl Pts',(-55.7374565106948,-60.0004827185225,
-7.17031832941094));
#34253=CARTESIAN_POINT('Ctrl Pts',(-55.7382921058495,-59.5354208239183,
-7.14423966167234));
#34254=CARTESIAN_POINT('Ctrl Pts',(-55.8149029736461,-59.070213340202,-7.11816099393374));
#34255=CARTESIAN_POINT('Ctrl Pts',(-55.9641984444257,-58.6286260986936,
-7.09208232619514));
#34256=CARTESIAN_POINT('Ctrl Pts',(-56.187307036103,-57.9687138653137,-7.05311011356471));
#34257=CARTESIAN_POINT('Ctrl Pts',(-56.572739258111,-57.3615517785553,-7.01413790093428));
#34258=CARTESIAN_POINT('Ctrl Pts',(-57.0811317284725,-56.8879006559434,
-6.97516568830384));
#34259=CARTESIAN_POINT('Ctrl Pts',(-58.0979166691954,-55.9405984107196,
-6.89722126304298));
#34260=CARTESIAN_POINT('Ctrl Pts',(-59.6065426033322,-55.5273400220822,
-6.81927683778213));
#34261=CARTESIAN_POINT('Ctrl Pts',(-60.9556943852598,-55.8380992060676,
-6.74133241252127));
#34262=CARTESIAN_POINT('Ctrl Pts',(-62.3048461671874,-56.148858390053,-6.66338798726041));
#34263=CARTESIAN_POINT('Ctrl Pts',(-63.4945237969059,-57.1836351466612,
-6.58544356199955));
#34264=CARTESIAN_POINT('Ctrl Pts',(-63.9892745582629,-58.4766948843557,
-6.50749913673869));
#34265=CARTESIAN_POINT('Ctrl Pts',(-64.48402531962,-59.7697546220501,-6.42955471147783));
#34266=CARTESIAN_POINT('Ctrl Pts',(-64.2838492126156,-61.3210973408307,
-6.35161028621697));
#34267=CARTESIAN_POINT('Ctrl Pts',(-63.4866149367798,-62.4593638601133,
-6.27366586095611));
#34268=CARTESIAN_POINT('Ctrl Pts',(-63.0879977988619,-63.0284971197546,
-6.23469364832568));
#34269=CARTESIAN_POINT('Ctrl Pts',(-62.5401161187362,-63.4943613295214,
-6.19572143569525));
#34270=CARTESIAN_POINT('Ctrl Pts',(-61.9174955417529,-63.8067796653494,
-6.15674922306482));
#34271=CARTESIAN_POINT('Ctrl Pts',(-61.2948749647697,-64.1191980011775,
-6.11777701043439));
#34272=CARTESIAN_POINT('Ctrl Pts',(-60.597515490929,-64.2781704630668,-6.07880479780396));
#34273=CARTESIAN_POINT('Ctrl Pts',(-59.9025382047836,-64.2624886515656,
-6.03983258517353));
#34274=CARTESIAN_POINT('Ctrl Pts',(-59.2075609186382,-64.2468068400645,
-6.0008603725431));
#34275=CARTESIAN_POINT('Ctrl Pts',(-58.5149658201879,-64.0564707551729,
-5.96188815991268));
#34276=CARTESIAN_POINT('Ctrl Pts',(-57.9084053535882,-63.7150280406438,
-5.92291594728225));
#34277=CARTESIAN_POINT('Ctrl Pts',(-57.3018448869884,-63.3735853261147,
-5.88394373465182));
#34278=CARTESIAN_POINT('Ctrl Pts',(-56.781319052239,-62.8810359819482,-5.84497152202138));
#34279=CARTESIAN_POINT('Ctrl Pts',(-56.4069717968208,-62.2947294084888,
-5.80599930939095));
#34280=CARTESIAN_POINT('Ctrl Pts',(-56.0326245414025,-61.7084228350294,
-5.76702709676052));
#34281=CARTESIAN_POINT('Ctrl Pts',(-55.8044558653154,-61.0283590322772,
-5.7280548841301));
#34282=CARTESIAN_POINT('Ctrl Pts',(-55.7497674522892,-60.3347286874856,
-5.68908267149967));
#34283=CARTESIAN_POINT('Ctrl Pts',(-55.7409903260494,-60.2234056345178,
-5.68282789080343));
#34284=CARTESIAN_POINT('Ctrl Pts',(-55.7366817240644,-60.1117331330244,
-5.67657311010719));
#34285=CARTESIAN_POINT('Ctrl Pts',(-55.7367829988534,-60.0000543459286,
-5.67031832941095));
#34286=CARTESIAN_POINT('Ctrl Pts',(-55.7373026458209,-59.9946120201631,
-6.07968167058906));
#34287=CARTESIAN_POINT('Ctrl Pts',(-55.7471880086661,-61.0607260097358,
-6.13934364288562));
#34288=CARTESIAN_POINT('Ctrl Pts',(-56.1540184553338,-62.1354535990912,
-6.19900561518218));
#34289=CARTESIAN_POINT('Ctrl Pts',(-56.8759755604507,-62.9112256731964,
-6.25866758747873));
#34290=CARTESIAN_POINT('Ctrl Pts',(-57.8191648224755,-63.9247206369396,
-6.33661201273959));
#34291=CARTESIAN_POINT('Ctrl Pts',(-59.3002026939739,-64.4279674072641,
-6.41455643800045));
#34292=CARTESIAN_POINT('Ctrl Pts',(-60.6732080679322,-64.2132805110372,
-6.49250086326132));
#34293=CARTESIAN_POINT('Ctrl Pts',(-61.3597107549114,-64.1059370629238,
-6.53147307589175));
#34294=CARTESIAN_POINT('Ctrl Pts',(-62.0192053175055,-63.8191101981725,
-6.57044528852218));
#34295=CARTESIAN_POINT('Ctrl Pts',(-62.5738278800212,-63.3976182232817,
-6.60941750115261));
#34296=CARTESIAN_POINT('Ctrl Pts',(-63.128450442537,-62.976126248391,-6.64838971378304));
#34297=CARTESIAN_POINT('Ctrl Pts',(-63.5782010049745,-62.4199691633608,
-6.68736192641346));
#34298=CARTESIAN_POINT('Ctrl Pts',(-63.8700858607814,-61.7890620281216,
-6.72633413904389));
#34299=CARTESIAN_POINT('Ctrl Pts',(-64.1619707165883,-61.1581548928825,
-6.76530635167432));
#34300=CARTESIAN_POINT('Ctrl Pts',(-64.2959898657645,-60.4524977074343,
-6.80427856430475));
#34301=CARTESIAN_POINT('Ctrl Pts',(-64.2564570806599,-59.7575622002848,
-6.84325077693518));
#34302=CARTESIAN_POINT('Ctrl Pts',(-64.2169242955553,-59.0626266931353,
-6.88222298956561));
#34303=CARTESIAN_POINT('Ctrl Pts',(-64.0038395761699,-58.3784128642844,
-6.92119520219604));
#34304=CARTESIAN_POINT('Ctrl Pts',(-63.6422173312568,-57.7841730064991,
-6.96016741482647));
#34305=CARTESIAN_POINT('Ctrl Pts',(-63.2805950863436,-57.1899331487137,
-6.9991396274569));
#34306=CARTESIAN_POINT('Ctrl Pts',(-62.7704353159028,-56.6856672619939,
-7.03811184008733));
#34307=CARTESIAN_POINT('Ctrl Pts',(-62.1717193363373,-56.3311916604974,
-7.07708405271776));
#34308=CARTESIAN_POINT('Ctrl Pts',(-61.5730033567719,-55.9767160590009,
-7.11605626534819));
#34309=CARTESIAN_POINT('Ctrl Pts',(-60.8857311680819,-55.7720307427277,
-7.15502847797862));
#34310=CARTESIAN_POINT('Ctrl Pts',(-60.190680876938,-55.7409438651642,-7.19400069060905));
#34311=CARTESIAN_POINT('Ctrl Pts',(-59.495630585794,-55.7098569876007,-7.23297290323948));
#34312=CARTESIAN_POINT('Ctrl Pts',(-58.7928021921962,-55.8523685487467,
-7.27194511586991));
#34313=CARTESIAN_POINT('Ctrl Pts',(-58.1648124824129,-56.1518435245449,
-7.31091732850034));
#34314=CARTESIAN_POINT('Ctrl Pts',(-57.5368227726295,-56.451318500343,-7.34988954113077));
#34315=CARTESIAN_POINT('Ctrl Pts',(-56.9836717466607,-56.9077568907933,
-7.3888617537612));
#34316=CARTESIAN_POINT('Ctrl Pts',(-56.5703777608788,-57.4674529656122,
-7.42783396639163));
#34317=CARTESIAN_POINT('Ctrl Pts',(-56.1570837750969,-58.0271490404312,
-7.46680617902206));
#34318=CARTESIAN_POINT('Ctrl Pts',(-55.8836468295019,-58.6901027996189,
-7.50577839165249));
#34319=CARTESIAN_POINT('Ctrl Pts',(-55.7822086101274,-59.3784126697627,
-7.54475060428292));
#34320=CARTESIAN_POINT('Ctrl Pts',(-55.7519020153531,-59.5840583173523,
-7.55639429305163));
#34321=CARTESIAN_POINT('Ctrl Pts',(-55.7369485277219,-59.7919673252401,
-7.56803798182035));
#34322=CARTESIAN_POINT('Ctrl Pts',(-55.7371269462215,-59.9999021904687,
-7.57968167058906));
#34323=CARTESIAN_POINT('Origin',(-60.,-60.,-6.));
#34324=CARTESIAN_POINT('',(-55.7367869775695,-59.9999237120217,-9.07968167058906));
#34325=CARTESIAN_POINT('',(-55.7373303432786,-59.9999992452069,-8.67031832941095));
#34326=CARTESIAN_POINT('',(-55.737,-60.,-6.));
#34327=CARTESIAN_POINT('',(-63.2233527839579,-57.2101674189746,-10.));
#34328=CARTESIAN_POINT('Ctrl Pts',(-55.7367869775695,-59.9999237120217,
-9.07968167058906));
#34329=CARTESIAN_POINT('Ctrl Pts',(-55.7372968491093,-60.6063764601996,
-9.11364895864637));
#34330=CARTESIAN_POINT('Ctrl Pts',(-55.8681266217369,-61.2130420485546,
-9.14761624670367));
#34331=CARTESIAN_POINT('Ctrl Pts',(-56.1191760941168,-61.7650316055626,
-9.18158353476097));
#34332=CARTESIAN_POINT('Ctrl Pts',(-56.4072165582787,-62.3983542997147,
-9.2205557473914));
#34333=CARTESIAN_POINT('Ctrl Pts',(-56.853514419077,-62.9597013825716,-9.25952796002183));
#34334=CARTESIAN_POINT('Ctrl Pts',(-57.4056092377689,-63.3830862709465,
-9.29850017265226));
#34335=CARTESIAN_POINT('Ctrl Pts',(-57.9577040564609,-63.8064711593214,
-9.33747238528269));
#34336=CARTESIAN_POINT('Ctrl Pts',(-58.6155958330465,-64.0918938532141,
-9.37644459791312));
#34337=CARTESIAN_POINT('Ctrl Pts',(-59.301954238806,-64.205811785771,-9.41541681054355));
#34338=CARTESIAN_POINT('Ctrl Pts',(-59.9883126445655,-64.3197297183279,
-9.45438902317399));
#34339=CARTESIAN_POINT('Ctrl Pts',(-60.7031376794989,-64.2621428895488,
-9.49336123580442));
#34340=CARTESIAN_POINT('Ctrl Pts',(-61.3624026668752,-64.039804899767,-9.53233344843485));
#34341=CARTESIAN_POINT('Ctrl Pts',(-62.0216676542516,-63.8174669099853,
-9.57130566106527));
#34342=CARTESIAN_POINT('Ctrl Pts',(-62.6253725940708,-63.4303777592007,
-9.6102778736957));
#34343=CARTESIAN_POINT('Ctrl Pts',(-63.1025601873701,-62.9240723675456,
-9.64925008632613));
#34344=CARTESIAN_POINT('Ctrl Pts',(-63.5797477806694,-62.4177669758905,
-9.68822229895656));
#34345=CARTESIAN_POINT('Ctrl Pts',(-63.9304180274487,-61.7922453433649,
-9.72719451158699));
#34346=CARTESIAN_POINT('Ctrl Pts',(-64.1133346946325,-61.1209649250503,
-9.76616672421742));
#34347=CARTESIAN_POINT('Ctrl Pts',(-64.2962513618163,-60.4496845067356,
-9.80513893684785));
#34348=CARTESIAN_POINT('Ctrl Pts',(-64.3114144494046,-59.7326453026318,
-9.84411114947828));
#34349=CARTESIAN_POINT('Ctrl Pts',(-64.1570473520141,-59.054316233321,-9.88308336210871));
#34350=CARTESIAN_POINT('Ctrl Pts',(-64.0026802546237,-58.3759871640102,
-9.92205557473914));
#34351=CARTESIAN_POINT('Ctrl Pts',(-63.6787829722545,-57.7363682294924,
-9.96102778736957));
#34352=CARTESIAN_POINT('Ctrl Pts',(-63.2233527839579,-57.2101674189746,
-10.));
#34353=CARTESIAN_POINT('',(-56.7764331763494,-57.2100813324657,-10.));
#34354=CARTESIAN_POINT('Origin',(-60.,-60.,-10.));
#34355=CARTESIAN_POINT('Ctrl Pts',(-56.7764331763494,-57.2100813324657,
-10.));
#34356=CARTESIAN_POINT('Ctrl Pts',(-57.1737624330954,-56.751787072741,-9.96602721186202));
#34357=CARTESIAN_POINT('Ctrl Pts',(-57.669807126483,-56.3786504952751,-9.93205442372405));
#34358=CARTESIAN_POINT('Ctrl Pts',(-58.2209772157099,-56.1255712923699,
-9.89808163558608));
#34359=CARTESIAN_POINT('Ctrl Pts',(-58.8532573166438,-55.8352490359833,
-9.85910942295565));
#34360=CARTESIAN_POINT('Ctrl Pts',(-59.5580810781206,-55.7029193217492,
-9.82013721032522));
#34361=CARTESIAN_POINT('Ctrl Pts',(-60.2526054566513,-55.7441421593256,
-9.78116499769479));
#34362=CARTESIAN_POINT('Ctrl Pts',(-60.947129835182,-55.785364996902,-9.74219278506436));
#34363=CARTESIAN_POINT('Ctrl Pts',(-61.6313548307664,-56.0001403862888,
-9.70322057243393));
#34364=CARTESIAN_POINT('Ctrl Pts',(-62.2248512157896,-56.3632202234726,
-9.6642483598035));
#34365=CARTESIAN_POINT('Ctrl Pts',(-62.8183476008128,-56.7263000606564,
-9.62527614717307));
#34366=CARTESIAN_POINT('Ctrl Pts',(-63.3211153752746,-57.2376843456373,
-9.58630393454265));
#34367=CARTESIAN_POINT('Ctrl Pts',(-63.6740580651529,-57.8372638312712,
-9.54733172191222));
#34368=CARTESIAN_POINT('Ctrl Pts',(-64.0270007550312,-58.4368433169052,
-9.50835950928179));
#34369=CARTESIAN_POINT('Ctrl Pts',(-64.2301183603261,-59.1246180031922,
-9.46938729665136));
#34370=CARTESIAN_POINT('Ctrl Pts',(-64.2595350229124,-59.8197432549321,
-9.43041508402093));
#34371=CARTESIAN_POINT('Ctrl Pts',(-64.2889516854988,-60.514868506672,-9.3914428713905));
#34372=CARTESIAN_POINT('Ctrl Pts',(-64.1446674053766,-61.2173443238648,
-9.35247065876007));
#34373=CARTESIAN_POINT('Ctrl Pts',(-63.8436422372794,-61.8445988100496,
-9.31349844612964));
#34374=CARTESIAN_POINT('Ctrl Pts',(-63.5426170691822,-62.4718532962343,
-9.27452623349921));
#34375=CARTESIAN_POINT('Ctrl Pts',(-63.0848510131098,-63.023886451411,-9.23555402086878));
#34376=CARTESIAN_POINT('Ctrl Pts',(-62.5241518227932,-63.4358097166499,
-9.19658180823835));
#34377=CARTESIAN_POINT('Ctrl Pts',(-61.9634526324765,-63.8477329818888,
-9.15760959560792));
#34378=CARTESIAN_POINT('Ctrl Pts',(-61.2998203079155,-64.1195463571897,
-9.11863738297749));
#34379=CARTESIAN_POINT('Ctrl Pts',(-60.6112612120411,-64.2192997468536,
-9.07966517034706));
#34380=CARTESIAN_POINT('Ctrl Pts',(-59.9227021161667,-64.3190531365174,
-9.04069295771663));
#34381=CARTESIAN_POINT('Ctrl Pts',(-59.209216248979,-64.246746540544,-9.0017207450862));
#34382=CARTESIAN_POINT('Ctrl Pts',(-58.5546698865512,-64.0108791546658,
-8.96274853245577));
#34383=CARTESIAN_POINT('Ctrl Pts',(-57.9001235241234,-63.7750117687875,
-8.92377631982534));
#34384=CARTESIAN_POINT('Ctrl Pts',(-57.3045166664556,-63.3755835930045,
-8.88480410719491));
#34385=CARTESIAN_POINT('Ctrl Pts',(-56.8378596441864,-62.8595452525819,
-8.84583189456448));
#34386=CARTESIAN_POINT('Ctrl Pts',(-56.3712026219172,-62.3435069121593,
-8.80685968193405));
#34387=CARTESIAN_POINT('Ctrl Pts',(-56.0334954350465,-61.7108584070972,
-8.76788746930362));
#34388=CARTESIAN_POINT('Ctrl Pts',(-55.864433621884,-61.0359639683527,-8.72891525667319));
#34389=CARTESIAN_POINT('Ctrl Pts',(-55.7797022872564,-60.6977166405979,
-8.70938294758578));
#34390=CARTESIAN_POINT('Ctrl Pts',(-55.7373324674286,-60.3488576861761,
-8.68985063849836));
#34391=CARTESIAN_POINT('Ctrl Pts',(-55.7373303432786,-59.9999992452069,
-8.67031832941095));
#34392=CARTESIAN_POINT('Origin',(-60.,-60.,-13.3123464956316));
#34393=CARTESIAN_POINT('',(-54.9005857767199,-59.9999919028974,-3.68765350436841));
#34394=CARTESIAN_POINT('',(-54.9008894996693,-60.0001150529132,-3.56234649563159));
#34395=CARTESIAN_POINT('',(-54.901,-60.,-13.3123464956316));
#34396=CARTESIAN_POINT('',(-63.6032183801568,-56.3921449163111,-3.));
#34397=CARTESIAN_POINT('Ctrl Pts',(-54.9008894996694,-60.0001150529132,
-3.56234649563159));
#34398=CARTESIAN_POINT('Ctrl Pts',(-54.9015383135063,-59.326085801412,-3.53078651427611));
#34399=CARTESIAN_POINT('Ctrl Pts',(-55.2021867542944,-57.8191582190388,
-3.4602543202902));
#34400=CARTESIAN_POINT('Ctrl Pts',(-56.6444156037563,-55.8880831676333,
-3.35074991367387));
#34401=CARTESIAN_POINT('Ctrl Pts',(-58.972955243809,-54.7929300280156,-3.23383327578258));
#34402=CARTESIAN_POINT('Ctrl Pts',(-61.543255288011,-54.9220257467759,-3.11691663789129));
#34403=CARTESIAN_POINT('Ctrl Pts',(-63.0142489447553,-55.8039324061734,
-3.03897221263043));
#34404=CARTESIAN_POINT('Ctrl Pts',(-63.6032183801568,-56.3921449163111,
-3.));
#34405=CARTESIAN_POINT('',(-64.9263786176897,-58.683468154111,-3.));
#34406=CARTESIAN_POINT('Origin',(-60.,-60.,-3.));
#34407=CARTESIAN_POINT('Ctrl Pts',(-54.90058577672,-59.9999919028974,-3.68765350436841));
#34408=CARTESIAN_POINT('Ctrl Pts',(-54.9005849893558,-59.9917925604521,
-3.68726952086906));
#34409=CARTESIAN_POINT('Ctrl Pts',(-54.9025709850474,-59.1514054532116,
-3.64791332473929));
#34410=CARTESIAN_POINT('Ctrl Pts',(-55.3285862434613,-57.4808672502626,
-3.56958491597908));
#34411=CARTESIAN_POINT('Ctrl Pts',(-57.0626757333642,-55.5795636292569,
-3.45266827808779));
#34412=CARTESIAN_POINT('Ctrl Pts',(-59.4872942572559,-54.7174568855574,
-3.3357516401965));
#34413=CARTESIAN_POINT('Ctrl Pts',(-62.032451512693,-55.097214824058,-3.21883500230521));
#34414=CARTESIAN_POINT('Ctrl Pts',(-64.0113857967048,-56.5640445520485,
-3.10691778890638));
#34415=CARTESIAN_POINT('Ctrl Pts',(-64.738468572607,-57.9827263087995,-3.03397278813797));
#34416=CARTESIAN_POINT('Ctrl Pts',(-64.9263786176897,-58.683468154111,-3.));
#34417=CARTESIAN_POINT('Origin',(-60.,-60.,-13.3123464956316));
#34418=CARTESIAN_POINT('',(-54.9007404436203,-60.0000650034929,-5.18765350436841));
#34419=CARTESIAN_POINT('',(-54.9012719965578,-60.0000880559789,-5.06234649563159));
#34420=CARTESIAN_POINT('',(-54.901,-60.,-13.3123464956316));
#34421=CARTESIAN_POINT('Ctrl Pts',(-54.9012719965578,-60.0000880559789,
-5.06234649563159));
#34422=CARTESIAN_POINT('Ctrl Pts',(-54.9016210803273,-59.4677293585841,
-5.0374252784717));
#34423=CARTESIAN_POINT('Ctrl Pts',(-55.114536066124,-58.1025886329227,-4.97353184868138));
#34424=CARTESIAN_POINT('Ctrl Pts',(-56.3134109850716,-56.1819888457558,
-4.87066620626063));
#34425=CARTESIAN_POINT('Ctrl Pts',(-58.5427258897122,-54.8966206707426,
-4.75374956836934));
#34426=CARTESIAN_POINT('Ctrl Pts',(-61.1146285526069,-54.8109981670255,
-4.63683293047805));
#34427=CARTESIAN_POINT('Ctrl Pts',(-63.424494989862,-55.9452536147892,-4.51991629258676));
#34428=CARTESIAN_POINT('Ctrl Pts',(-64.9293002326319,-58.0327345315151,
-4.40299965469548));
#34429=CARTESIAN_POINT('Ctrl Pts',(-65.2752818507472,-60.5826980463265,
-4.28608301680418));
#34430=CARTESIAN_POINT('Ctrl Pts',(-64.381102712243,-62.9956755106081,-4.16916637891289));
#34431=CARTESIAN_POINT('Ctrl Pts',(-62.4569756051562,-64.7044030653083,
-4.0522497410216));
#34432=CARTESIAN_POINT('Ctrl Pts',(-59.9552391145712,-65.3071771254814,
-3.93533310313031));
#34433=CARTESIAN_POINT('Ctrl Pts',(-57.4640288862619,-64.6622934850025,
-3.81841646523903));
#34434=CARTESIAN_POINT('Ctrl Pts',(-55.5689898565188,-62.921354421668,-3.70149982734774));
#34435=CARTESIAN_POINT('Ctrl Pts',(-54.9459957256052,-61.1489679675317,
-3.61614317081193));
#34436=CARTESIAN_POINT('Ctrl Pts',(-54.9007371181404,-60.1584187173525,
-3.56975872690654));
#34437=CARTESIAN_POINT('Ctrl Pts',(-54.9008894996694,-60.0001150529132,
-3.56234649563159));
#34438=CARTESIAN_POINT('Ctrl Pts',(-54.9007404436203,-60.0000650034929,
-5.18765350436841));
#34439=CARTESIAN_POINT('Ctrl Pts',(-54.9013740771447,-59.3013380632403,
-5.15493607243422));
#34440=CARTESIAN_POINT('Ctrl Pts',(-55.2189957750169,-57.7698537702076,
-5.0832464278696));
#34441=CARTESIAN_POINT('Ctrl Pts',(-56.7044889980166,-55.8396721524265,
-4.97258457067455));
#34442=CARTESIAN_POINT('Ctrl Pts',(-59.0489177395961,-54.7785641063853,
-4.85566793278326));
#34443=CARTESIAN_POINT('Ctrl Pts',(-61.6168265507944,-54.9449006597622,
-4.73875129489197));
#34444=CARTESIAN_POINT('Ctrl Pts',(-63.8046877645853,-56.2996615825733,
-4.62183465700068));
#34445=CARTESIAN_POINT('Ctrl Pts',(-65.0980856519831,-58.5243188288231,
-4.50491801910939));
#34446=CARTESIAN_POINT('Ctrl Pts',(-65.1929908727149,-61.0958980618402,
-4.3880013812181));
#34447=CARTESIAN_POINT('Ctrl Pts',(-64.0670764169607,-63.4098411642031,
-4.27108474332681));
#34448=CARTESIAN_POINT('Ctrl Pts',(-61.9850396640587,-64.922169576908,-4.15416810543552));
#34449=CARTESIAN_POINT('Ctrl Pts',(-59.4363409557176,-65.2773498680853,
-4.03725146754424));
#34450=CARTESIAN_POINT('Ctrl Pts',(-57.0201528179928,-64.3918838717894,
-3.92033482965294));
#34451=CARTESIAN_POINT('Ctrl Pts',(-55.3101280285781,-62.4802335661766,
-3.803802175261));
#34452=CARTESIAN_POINT('Ctrl Pts',(-54.9006649024818,-60.8239807085089,
-3.72624173349949));
#34453=CARTESIAN_POINT('Ctrl Pts',(-54.90058577672,-59.9999919028974,-3.68765350436841));
#34454=CARTESIAN_POINT('Origin',(-60.,-60.,-13.3123464956316));
#34455=CARTESIAN_POINT('',(-54.9015460351941,-60.0005773825349,-6.68765350436841));
#34456=CARTESIAN_POINT('',(-54.9013619964909,-59.993555404835,-6.56234649563159));
#34457=CARTESIAN_POINT('',(-54.901,-60.,-13.3123464956316));
#34458=CARTESIAN_POINT('Ctrl Pts',(-54.9013619964909,-59.993555404835,-6.56234649563159));
#34459=CARTESIAN_POINT('Ctrl Pts',(-54.8977387393831,-59.6027953335095,
-6.54406404266729));
#34460=CARTESIAN_POINT('Ctrl Pts',(-55.1133264945161,-57.5511818397621,
-6.44783716444213));
#34461=CARTESIAN_POINT('Ctrl Pts',(-57.2611355705387,-55.1183391042526,
-6.31263807358654));
#34462=CARTESIAN_POINT('Ctrl Pts',(-60.6812398138874,-54.7414747298955,
-6.15674922306482));
#34463=CARTESIAN_POINT('Ctrl Pts',(-63.0733672306018,-55.6714881210263,
-6.03983258517353));
#34464=CARTESIAN_POINT('Ctrl Pts',(-64.7488468685178,-57.6299773495695,
-5.92291594728224));
#34465=CARTESIAN_POINT('Ctrl Pts',(-65.3052031061324,-60.1405546503375,
-5.80599930939095));
#34466=CARTESIAN_POINT('Ctrl Pts',(-64.6156238857644,-62.6204341592567,
-5.68908267149966));
#34467=CARTESIAN_POINT('Ctrl Pts',(-62.8403791725874,-64.4831910135561,
-5.57216603360837));
#34468=CARTESIAN_POINT('Ctrl Pts',(-60.3976628726492,-65.2925026120897,
-5.45524939571708));
#34469=CARTESIAN_POINT('Ctrl Pts',(-57.8613353265494,-64.8573722732082,
-5.33833275782579));
#34470=CARTESIAN_POINT('Ctrl Pts',(-55.8278421001908,-63.2804354591061,
-5.2214161199345));
#34471=CARTESIAN_POINT('Ctrl Pts',(-54.9995353787376,-61.4327780915017,
-5.1294206992031));
#34472=CARTESIAN_POINT('Ctrl Pts',(-54.9010751773401,-60.3002407169748,
-5.07639749110213));
#34473=CARTESIAN_POINT('Ctrl Pts',(-54.9012719965578,-60.0000880559789,
-5.06234649563159));
#34474=CARTESIAN_POINT('Ctrl Pts',(-54.9015460351941,-60.0005773825349,
-6.68765350436841));
#34475=CARTESIAN_POINT('Ctrl Pts',(-54.9025454955962,-59.4443140467181,
-6.66157483662981));
#34476=CARTESIAN_POINT('Ctrl Pts',(-55.1311200271658,-58.0563310394583,
-6.59652395626078));
#34477=CARTESIAN_POINT('Ctrl Pts',(-56.8226683737146,-55.391675711492,-6.45352865063088));
#34478=CARTESIAN_POINT('Ctrl Pts',(-61.3338598105922,-54.1559235864261,
-6.25866758747874));
#34479=CARTESIAN_POINT('Ctrl Pts',(-65.6028015656481,-57.869031736986,-6.02483431169615));
#34480=CARTESIAN_POINT('Ctrl Pts',(-65.0042219447148,-62.5079576829526,
-5.82997324854401));
#34481=CARTESIAN_POINT('Ctrl Pts',(-62.382923622443,-64.736849642231,-5.67408439802229));
#34482=CARTESIAN_POINT('Ctrl Pts',(-59.8805760101181,-65.3072934023813,
-5.557167760131));
#34483=CARTESIAN_POINT('Ctrl Pts',(-57.3953244921747,-64.6243069865738,
-5.44025112223971));
#34484=CARTESIAN_POINT('Ctrl Pts',(-55.5275122251888,-62.8568832667251,
-5.32333448434841));
#34485=CARTESIAN_POINT('Ctrl Pts',(-54.9378834983018,-61.0994765924383,
-5.23913527839132));
#34486=CARTESIAN_POINT('Ctrl Pts',(-54.9006193082346,-60.1336446740069,
-5.19390828506465));
#34487=CARTESIAN_POINT('Ctrl Pts',(-54.9007404436203,-60.0000650034929,
-5.18765350436841));
#34488=CARTESIAN_POINT('Origin',(-60.,-60.,-13.3123464956316));
#34489=CARTESIAN_POINT('',(-54.901395125587,-59.9999990971874,-8.18765350436841));
#34490=CARTESIAN_POINT('',(-54.9011518411408,-59.9998830094301,-8.06234649563159));
#34491=CARTESIAN_POINT('',(-54.901,-60.,-13.3123464956316));
#34492=CARTESIAN_POINT('Ctrl Pts',(-54.9011518411408,-59.9998830094301,
-8.06234649563159));
#34493=CARTESIAN_POINT('Ctrl Pts',(-54.9009384336978,-59.7511708635701,
-8.05070280686288));
#34494=CARTESIAN_POINT('Ctrl Pts',(-54.9786898953671,-58.6701368161215,
-8.00008690546374));
#34495=CARTESIAN_POINT('Ctrl Pts',(-55.7305243149913,-56.8472980856346,
-7.91049879143416));
#34496=CARTESIAN_POINT('Ctrl Pts',(-57.7154061456845,-55.2094519541036,
-7.79358215354287));
#34497=CARTESIAN_POINT('Ctrl Pts',(-60.2373779816841,-54.6980751417997,
-7.67666551565158));
#34498=CARTESIAN_POINT('Ctrl Pts',(-62.7035292062656,-55.4325511640916,
-7.55974887776029));
#34499=CARTESIAN_POINT('Ctrl Pts',(-64.5341447372141,-57.2420175654881,
-7.442832239869));
#34500=CARTESIAN_POINT('Ctrl Pts',(-65.2987604896043,-59.6971944221457,
-7.32591560197771));
#34501=CARTESIAN_POINT('Ctrl Pts',(-64.8178571527642,-62.229316863103,-7.20899896408642));
#34502=CARTESIAN_POINT('Ctrl Pts',(-63.2040090754463,-64.2249853898932,
-7.09208232619513));
#34503=CARTESIAN_POINT('Ctrl Pts',(-60.048707386807,-65.597286758288,-6.93619347567342));
#34504=CARTESIAN_POINT('Ctrl Pts',(-56.0355251757418,-64.2336342647843,
-6.75961486548556));
#34505=CARTESIAN_POINT('Ctrl Pts',(-54.9131859385852,-61.2687407749573,
-6.62200846792815));
#34506=CARTESIAN_POINT('Ctrl Pts',(-54.9013619964909,-59.993555404835,-6.56234649563159));
#34507=CARTESIAN_POINT('Ctrl Pts',(-54.901395125587,-59.9999990971874,-8.18765350436841));
#34508=CARTESIAN_POINT('Ctrl Pts',(-54.9013925968981,-59.5847014864836,
-8.1682136008254));
#34509=CARTESIAN_POINT('Ctrl Pts',(-55.0522173125255,-58.3368364086299,
-8.10980148465195));
#34510=CARTESIAN_POINT('Ctrl Pts',(-56.0593765808925,-56.444776458995,-8.01241715584808));
#34511=CARTESIAN_POINT('Ctrl Pts',(-58.1949365065413,-55.009018880156,-7.89550051795679));
#34512=CARTESIAN_POINT('Ctrl Pts',(-60.754850176949,-54.7465903023206,-7.7785838800655));
#34513=CARTESIAN_POINT('Ctrl Pts',(-63.1372997996482,-55.7191702494578,
-7.6616672421742));
#34514=CARTESIAN_POINT('Ctrl Pts',(-64.7822203636214,-57.6981473048777,
-7.54475060428292));
#34515=CARTESIAN_POINT('Ctrl Pts',(-65.3028606509933,-60.2182181776382,
-7.42783396639163));
#34516=CARTESIAN_POINT('Ctrl Pts',(-64.5769288134183,-62.6870882382886,
-7.31091732850035));
#34517=CARTESIAN_POINT('Ctrl Pts',(-62.7748568790513,-64.5240380041187,
-7.19400069060905));
#34518=CARTESIAN_POINT('Ctrl Pts',(-60.3207808627358,-65.2979018325692,
-7.07708405271776));
#34519=CARTESIAN_POINT('Ctrl Pts',(-57.7905711249098,-64.8252826799559,
-6.96016741482647));
#34520=CARTESIAN_POINT('Ctrl Pts',(-55.7813289378715,-63.2204602274652,
-6.84325077693518));
#34521=CARTESIAN_POINT('Ctrl Pts',(-54.9881850222051,-61.3817353652472,
-6.7524128067825));
#34522=CARTESIAN_POINT('Ctrl Pts',(-54.9010518923302,-60.2755993416288,
-6.70054704926024));
#34523=CARTESIAN_POINT('Ctrl Pts',(-54.9015460351941,-60.0005773825349,
-6.68765350436841));
#34524=CARTESIAN_POINT('Origin',(-60.,-60.,-13.3123464956316));
#34525=CARTESIAN_POINT('',(-54.9012106606313,-59.9998804662267,-9.68765350436841));
#34526=CARTESIAN_POINT('',(-54.9007452025866,-59.9999087514893,-9.56234649563159));
#34527=CARTESIAN_POINT('',(-54.901,-60.,-13.3123464956316));
#34528=CARTESIAN_POINT('',(-58.6771150344309,-64.9244061944433,-10.));
#34529=CARTESIAN_POINT('Ctrl Pts',(-58.677115034431,-64.9244061944433,-10.));
#34530=CARTESIAN_POINT('Ctrl Pts',(-57.8732233401272,-64.7084499564018,
-9.96102778736957));
#34531=CARTESIAN_POINT('Ctrl Pts',(-56.3739727010425,-63.8754866332611,
-9.88308336210871));
#34532=CARTESIAN_POINT('Ctrl Pts',(-55.1299740881578,-61.950738551684,-9.77896786356485));
#34533=CARTESIAN_POINT('Ctrl Pts',(-54.9016327839252,-60.5589070089215,
-9.71382457765142));
#34534=CARTESIAN_POINT('Ctrl Pts',(-54.9012106606313,-59.9998804662267,
-9.68765350436841));
#34535=CARTESIAN_POINT('',(-61.3230392926944,-64.9246350552985,-10.));
#34536=CARTESIAN_POINT('Origin',(-60.,-60.,-10.));
#34537=CARTESIAN_POINT('Ctrl Pts',(-61.3230392926944,-64.9246350552985,
-10.));
#34538=CARTESIAN_POINT('Ctrl Pts',(-60.6222240304355,-65.1122710972509,
-9.96602721186203));
#34539=CARTESIAN_POINT('Ctrl Pts',(-59.0300681563555,-65.1919398523856,
-9.89308221109362));
#34540=CARTESIAN_POINT('Ctrl Pts',(-56.7702891895575,-64.2115472965565,
-9.78116499769479));
#34541=CARTESIAN_POINT('Ctrl Pts',(-55.2373851602932,-62.2834824754791,
-9.66925328437662));
#34542=CARTESIAN_POINT('Ctrl Pts',(-54.9013550630092,-60.725290539657,-9.5963137836889));
#34543=CARTESIAN_POINT('Ctrl Pts',(-54.9007452025866,-59.9999087514893,
-9.56234649563159));
#34544=CARTESIAN_POINT('Origin',(60.,60.,-6.));
#34545=CARTESIAN_POINT('',(64.2627725569288,59.999926383973,-4.57968167058906));
#34546=CARTESIAN_POINT('',(64.2633463508187,60.0000067694975,-4.17031832941094));
#34547=CARTESIAN_POINT('',(64.263,60.,-6.));
#34548=CARTESIAN_POINT('',(60.8043894954945,55.8135783132205,-3.));
#34549=CARTESIAN_POINT('Ctrl Pts',(64.2633463508187,60.0000067694975,-4.17031832941094));
#34550=CARTESIAN_POINT('Ctrl Pts',(64.2633470090911,60.0068617993432,-4.16993434591159));
#34551=CARTESIAN_POINT('Ctrl Pts',(64.2633308093496,60.0137168260627,-4.16955036241224));
#34552=CARTESIAN_POINT('Ctrl Pts',(64.2632977324257,60.0205717713411,-4.16916637891289));
#34553=CARTESIAN_POINT('Ctrl Pts',(64.2599406066242,60.7163110033908,-4.13019416628246));
#34554=CARTESIAN_POINT('Ctrl Pts',(64.0827293769352,61.4112112987266,-4.09122195365203));
#34555=CARTESIAN_POINT('Ctrl Pts',(63.7524939144254,62.0235910863766,-4.0522497410216));
#34556=CARTESIAN_POINT('Ctrl Pts',(63.4222584519156,62.6359708740266,-4.01327752839118));
#34557=CARTESIAN_POINT('Ctrl Pts',(62.938998756585,63.1658301539908,-3.97430531576075));
#34558=CARTESIAN_POINT('Ctrl Pts',(62.3595200208981,63.5508866522884,-3.93533310313031));
#34559=CARTESIAN_POINT('Ctrl Pts',(61.7800412852112,63.935943150586,-3.89636089049989));
#34560=CARTESIAN_POINT('Ctrl Pts',(61.104343509168,64.176196867217,-3.85738867786946));
#34561=CARTESIAN_POINT('Ctrl Pts',(60.4118497411081,64.243407855033,-3.81841646523903));
#34562=CARTESIAN_POINT('Ctrl Pts',(59.7193559730481,64.3106188428491,-3.7794442526086));
#34563=CARTESIAN_POINT('Ctrl Pts',(59.0100662129713,64.2047871018501,-3.74047203997816));
#34564=CARTESIAN_POINT('Ctrl Pts',(58.367356741015,63.9383514081819,-3.70149982734773));
#34565=CARTESIAN_POINT('Ctrl Pts',(57.7246472690586,63.6719157145136,-3.6625276147173));
#34566=CARTESIAN_POINT('Ctrl Pts',(57.1485180852227,63.2448760681761,-3.62355540208687));
#34567=CARTESIAN_POINT('Ctrl Pts',(56.7066830620729,62.7074312242854,-3.58458318945645));
#34568=CARTESIAN_POINT('Ctrl Pts',(56.2648480389232,62.1699863803947,-3.54561097682602));
#34569=CARTESIAN_POINT('Ctrl Pts',(55.9573071764596,61.5221363389508,-3.50663876419559));
#34570=CARTESIAN_POINT('Ctrl Pts',(55.8202250347853,60.8400271110314,-3.46766655156516));
#34571=CARTESIAN_POINT('Ctrl Pts',(55.683142893111,60.1579178831119,-3.42869433893473));
#34572=CARTESIAN_POINT('Ctrl Pts',(55.7165194722261,59.441549468717,-3.3897221263043));
#34573=CARTESIAN_POINT('Ctrl Pts',(55.9163990068928,58.775140191943,-3.35074991367387));
#34574=CARTESIAN_POINT('Ctrl Pts',(56.1162785415595,58.108730915169,-3.31177770104344));
#34575=CARTESIAN_POINT('Ctrl Pts',(56.4826610317779,57.4922807760161,-3.27280548841301));
#34576=CARTESIAN_POINT('Ctrl Pts',(56.9725486039278,56.9982300189206,-3.23383327578258));
#34577=CARTESIAN_POINT('Ctrl Pts',(57.4624361760777,56.5041792618252,-3.19486106315215));
#34578=CARTESIAN_POINT('Ctrl Pts',(58.0758288301591,56.1325278867873,-3.15588885052172));
#34579=CARTESIAN_POINT('Ctrl Pts',(58.7404625691261,55.927049222772,-3.11691663789129));
#34580=CARTESIAN_POINT('Ctrl Pts',(59.4050963080931,55.7215705587567,-3.07794442526086));
#34581=CARTESIAN_POINT('Ctrl Pts',(60.1209711319459,55.6822646057641,-3.03897221263043));
#34582=CARTESIAN_POINT('Ctrl Pts',(60.8043894954945,55.8135783132205,-3.));
#34583=CARTESIAN_POINT('',(64.0279238903325,61.3967314318666,-3.));
#34584=CARTESIAN_POINT('Origin',(60.,60.,-3.));
#34585=CARTESIAN_POINT('',(64.2630923348121,59.9999038151513,-3.07968167058906));
#34586=CARTESIAN_POINT('Ctrl Pts',(64.0279238903325,61.3967314318666,-3.));
#34587=CARTESIAN_POINT('Ctrl Pts',(64.1829036615969,60.9485583421562,-3.02656055686302));
#34588=CARTESIAN_POINT('Ctrl Pts',(64.2626358261587,60.4741561725529,-3.05312111372604));
#34589=CARTESIAN_POINT('Ctrl Pts',(64.2630923348121,59.9999038151513,-3.07968167058906));
#34590=CARTESIAN_POINT('',(64.263,60.,-2.));
#34591=CARTESIAN_POINT('',(64.263,60.,-6.));
#34592=CARTESIAN_POINT('Origin',(60.,60.,-2.));
#34593=CARTESIAN_POINT('Ctrl Pts',(64.2630923348121,59.9999038151513,-3.07968167058906));
#34594=CARTESIAN_POINT('Ctrl Pts',(64.2632197322811,59.8675546263191,-3.08709390186401));
#34595=CARTESIAN_POINT('Ctrl Pts',(64.257173175386,59.7352171047975,-3.09450613313896));
#34596=CARTESIAN_POINT('Ctrl Pts',(64.2448651193736,59.6034645637425,-3.10191836441392));
#34597=CARTESIAN_POINT('Ctrl Pts',(64.180151518544,58.9107327999692,-3.14089057704435));
#34598=CARTESIAN_POINT('Ctrl Pts',(63.942340524664,58.2341726576991,-3.17986278967478));
#34599=CARTESIAN_POINT('Ctrl Pts',(63.5593783060224,57.6533083171945,-3.21883500230521));
#34600=CARTESIAN_POINT('Ctrl Pts',(63.1764160873809,57.07244397669,-3.25780721493564));
#34601=CARTESIAN_POINT('Ctrl Pts',(62.6483026439779,56.5872754379511,-3.29677942756607));
#34602=CARTESIAN_POINT('Ctrl Pts',(62.0371180843352,56.2548324073596,-3.3357516401965));
#34603=CARTESIAN_POINT('Ctrl Pts',(61.4259335246925,55.9223893767681,-3.37472385282693));
#34604=CARTESIAN_POINT('Ctrl Pts',(60.7316778488101,55.742671854324,-3.41369606545736));
#34605=CARTESIAN_POINT('Ctrl Pts',(60.0359554314242,55.7368042611768,-3.45266827808779));
#34606=CARTESIAN_POINT('Ctrl Pts',(59.3402330140382,55.7309366680297,-3.49164049071822));
#34607=CARTESIAN_POINT('Ctrl Pts',(58.6430438551486,55.8989190041796,-3.53061270334864));
#34608=CARTESIAN_POINT('Ctrl Pts',(58.0263393924009,56.2210060567882,-3.56958491597907));
#34609=CARTESIAN_POINT('Ctrl Pts',(57.4096349296532,56.5430931093967,-3.6085571286095));
#34610=CARTESIAN_POINT('Ctrl Pts',(56.8734151630474,57.019284878464,-3.64752934123993));
#34611=CARTESIAN_POINT('Ctrl Pts',(56.4807094232938,57.5936075665364,-3.68650155387036));
#34612=CARTESIAN_POINT('Ctrl Pts',(56.0880036835401,58.1679302546087,-3.72547376650079));
#34613=CARTESIAN_POINT('Ctrl Pts',(55.8388119706386,58.8403838616862,-3.76444597913122));
#34614=CARTESIAN_POINT('Ctrl Pts',(55.7624255547685,59.5319252483343,-3.80341819176165));
#34615=CARTESIAN_POINT('Ctrl Pts',(55.6860391388985,60.2234666349825,-3.84239040439208));
#34616=CARTESIAN_POINT('Ctrl Pts',(55.7824580200599,60.9340958012014,-3.88136261702251));
#34617=CARTESIAN_POINT('Ctrl Pts',(56.0403485969429,61.580282158413,-3.92033482965294));
#34618=CARTESIAN_POINT('Ctrl Pts',(56.2982391738259,62.2264685156246,-3.95930704228337));
#34619=CARTESIAN_POINT('Ctrl Pts',(56.7176014464305,62.8082120638289,-3.9982792549138));
#34620=CARTESIAN_POINT('Ctrl Pts',(57.2491417880006,63.2571321784525,-4.03725146754423));
#34621=CARTESIAN_POINT('Ctrl Pts',(57.7806821295708,63.706052293076,-4.07622368017466));
#34622=CARTESIAN_POINT('Ctrl Pts',(58.4244005401064,64.0221489741188,-4.11519589280509));
#34623=CARTESIAN_POINT('Ctrl Pts',(59.1046313521504,64.1682665851206,-4.15416810543553));
#34624=CARTESIAN_POINT('Ctrl Pts',(59.7848621641945,64.3143841961224,-4.19314031806595));
#34625=CARTESIAN_POINT('Ctrl Pts',(60.5016053777469,64.2905227370833,-4.23211253069638));
#34626=CARTESIAN_POINT('Ctrl Pts',(61.1706120551988,64.0994874623445,-4.27108474332681));
#34627=CARTESIAN_POINT('Ctrl Pts',(61.8396187326508,63.9084521876057,-4.31005695595724));
#34628=CARTESIAN_POINT('Ctrl Pts',(62.4608888740024,63.5502430971673,-4.34902916858767));
#34629=CARTESIAN_POINT('Ctrl Pts',(62.9613950657551,63.0669646706093,-4.3880013812181));
#34630=CARTESIAN_POINT('Ctrl Pts',(63.4619012575079,62.5836862440512,-4.42697359384853));
#34631=CARTESIAN_POINT('Ctrl Pts',(63.8416434996618,61.9753384813737,-4.46594580647896));
#34632=CARTESIAN_POINT('Ctrl Pts',(64.0559863710237,61.3134314862707,-4.50491801910939));
#34633=CARTESIAN_POINT('Ctrl Pts',(64.1930503169315,60.8901676567048,-4.52983923626928));
#34634=CARTESIAN_POINT('Ctrl Pts',(64.2624807063128,60.4450028890856,-4.55476045342917));
#34635=CARTESIAN_POINT('Ctrl Pts',(64.2627725569288,59.999926383973,-4.57968167058906));
#34636=CARTESIAN_POINT('Origin',(60.,60.,-6.));
#34637=CARTESIAN_POINT('',(64.2626973799646,60.005388464797,-6.07968167058906));
#34638=CARTESIAN_POINT('',(64.2632169517948,59.999945593479,-5.67031832941094));
#34639=CARTESIAN_POINT('',(64.263,60.,-6.));
#34640=CARTESIAN_POINT('Ctrl Pts',(64.2632169517948,59.999945593479,-5.67031832941094));
#34641=CARTESIAN_POINT('Ctrl Pts',(64.2626872015258,60.5841136575979,-5.63760089747675));
#34642=CARTESIAN_POINT('Ctrl Pts',(64.141498283485,61.1684537725971,-5.60488346554256));
#34643=CARTESIAN_POINT('Ctrl Pts',(63.908043668822,61.7038522263494,-5.57216603360837));
#34644=CARTESIAN_POINT('Ctrl Pts',(63.6299581852027,62.3416058991808,-5.53319382097794));
#34645=CARTESIAN_POINT('Ctrl Pts',(63.1925789329281,62.9099162611984,-5.49422160834751));
#34646=CARTESIAN_POINT('Ctrl Pts',(62.6472141655169,63.3419273614047,-5.45524939571708));
#34647=CARTESIAN_POINT('Ctrl Pts',(62.1018493981057,63.773938461611,-5.41627718308665));
#34648=CARTESIAN_POINT('Ctrl Pts',(61.4484991155579,64.0696503000059,-5.37730497045622));
#34649=CARTESIAN_POINT('Ctrl Pts',(60.764008858737,64.1943287037686,-5.33833275782579));
#34650=CARTESIAN_POINT('Ctrl Pts',(60.0795186019162,64.3190071075312,-5.29936054519536));
#34651=CARTESIAN_POINT('Ctrl Pts',(59.3638883708224,64.2726520766615,-5.26038833256493));
#34652=CARTESIAN_POINT('Ctrl Pts',(58.7012143841293,64.0607007564596,-5.2214161199345));
#34653=CARTESIAN_POINT('Ctrl Pts',(58.0385403974362,63.8487494362578,-5.18244390730407));
#34654=CARTESIAN_POINT('Ctrl Pts',(57.4288226551439,63.4712018267237,-5.14347169467364));
#34655=CARTESIAN_POINT('Ctrl Pts',(56.9437403638198,62.9724419470908,-5.10449948204321));
#34656=CARTESIAN_POINT('Ctrl Pts',(56.4586580724957,62.473682067458,-5.06552726941278));
#34657=CARTESIAN_POINT('Ctrl Pts',(56.09821123214,61.8537099177263,-5.02655505678235));
#34658=CARTESIAN_POINT('Ctrl Pts',(55.9047636201273,61.1853972966568,-4.98758284415192));
#34659=CARTESIAN_POINT('Ctrl Pts',(55.7113160081146,60.5170846755874,-4.94861063152149));
#34660=CARTESIAN_POINT('Ctrl Pts',(55.684867624445,59.8004315831803,-4.90963841889106));
#34661=CARTESIAN_POINT('Ctrl Pts',(55.828529532945,59.1196777783533,-4.87066620626063));
#34662=CARTESIAN_POINT('Ctrl Pts',(55.972191441445,58.4389239735264,-4.8316939936302));
#34663=CARTESIAN_POINT('Ctrl Pts',(56.2859636421146,57.7940694562796,-4.79272178099977));
#34664=CARTESIAN_POINT('Ctrl Pts',(56.7329629271073,57.2609127709619,-4.75374956836934));
#34665=CARTESIAN_POINT('Ctrl Pts',(57.1799622121,56.7277560856442,-4.71477735573891));
#34666=CARTESIAN_POINT('Ctrl Pts',(57.7601885814157,56.3062972322555,-4.67580514310848));
#34667=CARTESIAN_POINT('Ctrl Pts',(58.4054401165192,56.0460766112725,-4.63683293047805));
#34668=CARTESIAN_POINT('Ctrl Pts',(59.0506916516226,55.7858559902895,-4.59786071784762));
#34669=CARTESIAN_POINT('Ctrl Pts',(59.7609683525138,55.6868736017121,-4.55888850521719));
#34670=CARTESIAN_POINT('Ctrl Pts',(60.4527808917702,55.7607641678725,-4.51991629258676));
#34671=CARTESIAN_POINT('Ctrl Pts',(61.1445934310265,55.8346547340329,-4.48094407995633));
#34672=CARTESIAN_POINT('Ctrl Pts',(61.8179418086481,56.0814182549311,-4.4419718673259));
#34673=CARTESIAN_POINT('Ctrl Pts',(62.3936777834231,56.4720490863694,-4.40299965469547));
#34674=CARTESIAN_POINT('Ctrl Pts',(62.969413758198,56.8626799178076,-4.36402744206504));
#34675=CARTESIAN_POINT('Ctrl Pts',(63.4475373301263,57.3971780597858,-4.32505522943461));
#34676=CARTESIAN_POINT('Ctrl Pts',(63.7718476051335,58.0127162151568,-4.28608301680418));
#34677=CARTESIAN_POINT('Ctrl Pts',(64.0929625318178,58.6221896264721,-4.2474947876731));
#34678=CARTESIAN_POINT('Ctrl Pts',(64.263280198064,59.3111139841629,-4.20890655854202));
#34679=CARTESIAN_POINT('Ctrl Pts',(64.2633463508187,60.0000067694975,-4.17031832941094));
#34680=CARTESIAN_POINT('Ctrl Pts',(64.2627725569288,59.999926383973,-4.57968167058906));
#34681=CARTESIAN_POINT('Ctrl Pts',(64.2629371071454,59.7489848702717,-4.5937326660596));
#34682=CARTESIAN_POINT('Ctrl Pts',(64.2411232668863,59.4980714142625,-4.60778366153014));
#34683=CARTESIAN_POINT('Ctrl Pts',(64.1970612964284,59.2511271660237,-4.62183465700068));
#34684=CARTESIAN_POINT('Ctrl Pts',(64.0748498499012,58.5661960684082,-4.66080686963111));
#34685=CARTESIAN_POINT('Ctrl Pts',(63.7814834562769,57.9118001007057,-4.69977908226154));
#34686=CARTESIAN_POINT('Ctrl Pts',(63.351451191029,57.3648701020231,-4.73875129489197));
#34687=CARTESIAN_POINT('Ctrl Pts',(62.9214189257811,56.8179401033406,-4.7777235075224));
#34688=CARTESIAN_POINT('Ctrl Pts',(62.3547207889096,56.378476073678,-4.81669572015283));
#34689=CARTESIAN_POINT('Ctrl Pts',(61.7179571787521,56.09811252218,-4.85566793278326));
#34690=CARTESIAN_POINT('Ctrl Pts',(61.0811935685946,55.8177489706819,-4.89464014541369));
#34691=CARTESIAN_POINT('Ctrl Pts',(60.374364485151,55.6964858973485,-4.93361235804412));
#34692=CARTESIAN_POINT('Ctrl Pts',(59.6805793162926,55.7486247247237,-4.97258457067455));
#34693=CARTESIAN_POINT('Ctrl Pts',(58.9867941474342,55.8007635520988,-5.01155678330498));
#34694=CARTESIAN_POINT('Ctrl Pts',(58.3060528931609,56.0263042801826,-5.05052899593541));
#34695=CARTESIAN_POINT('Ctrl Pts',(57.7183177787476,56.3986330544208,-5.08950120856584));
#34696=CARTESIAN_POINT('Ctrl Pts',(57.1305826643343,56.7709618286591,-5.12847342119627));
#34697=CARTESIAN_POINT('Ctrl Pts',(56.6358536897809,57.2900786490518,-5.16744563382669));
#34698=CARTESIAN_POINT('Ctrl Pts',(56.2924025719534,57.8951862105726,-5.20641784645712));
#34699=CARTESIAN_POINT('Ctrl Pts',(55.9489514541259,58.5002937720934,-5.24539005908756));
#34700=CARTESIAN_POINT('Ctrl Pts',(55.7567781930244,59.1913920747422,-5.28436227171799));
#34701=CARTESIAN_POINT('Ctrl Pts',(55.7382147113452,59.886767398621,-5.32333448434842));
#34702=CARTESIAN_POINT('Ctrl Pts',(55.719651229666,60.5821427224998,-5.36230669697885));
#34703=CARTESIAN_POINT('Ctrl Pts',(55.8746975274092,61.2817950676086,-5.40127890960928));
#34704=CARTESIAN_POINT('Ctrl Pts',(56.1856839431124,61.9045196740408,-5.44025112223971));
#34705=CARTESIAN_POINT('Ctrl Pts',(56.4966703588156,62.527244280473,-5.47922333487014));
#34706=CARTESIAN_POINT('Ctrl Pts',(56.9635968924788,63.0730411482287,-5.51819554750057));
#34707=CARTESIAN_POINT('Ctrl Pts',(57.530381347957,63.475527534543,-5.557167760131));
#34708=CARTESIAN_POINT('Ctrl Pts',(58.0971658034351,63.8780139208573,-5.59613997276143));
#34709=CARTESIAN_POINT('Ctrl Pts',(58.7638081807283,64.1371898257302,-5.63511218539186));
#34710=CARTESIAN_POINT('Ctrl Pts',(59.4545503724775,64.2273943548749,-5.67408439802229));
#34711=CARTESIAN_POINT('Ctrl Pts',(60.1452925642268,64.3175988840196,-5.71305661065272));
#34712=CARTESIAN_POINT('Ctrl Pts',(60.8601345704321,64.2388320374361,-5.75202882328315));
#34713=CARTESIAN_POINT('Ctrl Pts',(61.5092343352991,63.9908846520633,-5.79100103591358));
#34714=CARTESIAN_POINT('Ctrl Pts',(62.8074338650331,63.4949898813177,-5.86894546117444));
#34715=CARTESIAN_POINT('Ctrl Pts',(63.8426644294139,62.322372955415,-5.9468898864353));
#34716=CARTESIAN_POINT('Ctrl Pts',(64.1576093504471,60.9741927827568,-6.02483431169616));
#34717=CARTESIAN_POINT('Ctrl Pts',(64.2314820576467,60.6579669524741,-6.04311676466046));
#34718=CARTESIAN_POINT('Ctrl Pts',(64.2657266356665,60.3320821166483,-6.06139921762476));
#34719=CARTESIAN_POINT('Ctrl Pts',(64.2626973799646,60.005388464797,-6.07968167058906));
#34720=CARTESIAN_POINT('Origin',(60.,60.,-6.));
#34721=CARTESIAN_POINT('',(64.2628730117989,60.0000978162778,-7.57968167058906));
#34722=CARTESIAN_POINT('',(64.2625441198806,59.9995177541909,-7.17031832941094));
#34723=CARTESIAN_POINT('',(64.263,60.,-6.));
#34724=CARTESIAN_POINT('Ctrl Pts',(64.2625441198806,59.9995177541909,-7.17031832941094));
#34725=CARTESIAN_POINT('Ctrl Pts',(64.2617091262571,60.464580224433,-7.14423966167234));
#34726=CARTESIAN_POINT('Ctrl Pts',(64.1850989669132,60.929788399807,-7.11816099393374));
#34727=CARTESIAN_POINT('Ctrl Pts',(64.0358034903878,61.3713756586764,-7.09208232619513));
#34728=CARTESIAN_POINT('Ctrl Pts',(63.8126948901237,62.0312879180006,-7.0531101135647));
#34729=CARTESIAN_POINT('Ctrl Pts',(63.4272610645377,62.6384485248234,-7.01413790093427));
#34730=CARTESIAN_POINT('Ctrl Pts',(62.9188676932756,63.112098827234,-6.97516568830384));
#34731=CARTESIAN_POINT('Ctrl Pts',(61.9020809507514,64.0593994320554,-6.89722126304298));
#34732=CARTESIAN_POINT('Ctrl Pts',(60.3934560255232,64.4726588192284,-6.81927683778212));
#34733=CARTESIAN_POINT('Ctrl Pts',(59.0443048432248,64.1619002172936,-6.74133241252127));
#34734=CARTESIAN_POINT('Ctrl Pts',(57.6951536609264,63.8511416153587,-6.66338798726041));
#34735=CARTESIAN_POINT('Ctrl Pts',(56.5054762215579,62.816365024316,-6.58544356199954));
#34736=CARTESIAN_POINT('Ctrl Pts',(56.0107261197417,61.523305799792,-6.50749913673868));
#34737=CARTESIAN_POINT('Ctrl Pts',(55.5159760179255,60.230246575268,-6.42955471147782));
#34738=CARTESIAN_POINT('Ctrl Pts',(55.7161532536617,58.6789047172628,-6.35161028621697));
#34739=CARTESIAN_POINT('Ctrl Pts',(56.5133856551997,57.5406366409267,-6.27366586095611));
#34740=CARTESIAN_POINT('Ctrl Pts',(56.9120018559687,56.9715026027586,-6.23469364832568));
#34741=CARTESIAN_POINT('Ctrl Pts',(57.4598818481882,56.5056370100079,-6.19572143569525));
#34742=CARTESIAN_POINT('Ctrl Pts',(58.0825024496753,56.1932186620801,-6.15674922306482));
#34743=CARTESIAN_POINT('Ctrl Pts',(58.7051230511624,55.8808003141523,-6.11777701043439));
#34744=CARTESIAN_POINT('Ctrl Pts',(59.4024842619172,55.7218292110476,-6.07880479780396));
#34745=CARTESIAN_POINT('Ctrl Pts',(60.0974620054189,55.7375114038248,-6.03983258517353));
#34746=CARTESIAN_POINT('Ctrl Pts',(60.7924397489205,55.753193596602,-6.0008603725431));
#34747=CARTESIAN_POINT('Ctrl Pts',(61.4850340251691,55.943529085261,-5.96188815991267));
#34748=CARTESIAN_POINT('Ctrl Pts',(62.0915943313093,56.2849716792125,-5.92291594728224));
#34749=CARTESIAN_POINT('Ctrl Pts',(62.6981546374495,56.626414273164,-5.88394373465181));
#34750=CARTESIAN_POINT('Ctrl Pts',(63.2186809734814,57.1189639724079,-5.84497152202138));
#34751=CARTESIAN_POINT('Ctrl Pts',(63.5930283536401,57.7052706411259,-5.80599930939095));
#34752=CARTESIAN_POINT('Ctrl Pts',(63.9673757337987,58.2915773098439,-5.76702709676052));
#34753=CARTESIAN_POINT('Ctrl Pts',(64.1955441580842,58.9716409480359,-5.72805488413009));
#34754=CARTESIAN_POINT('Ctrl Pts',(64.2502325127449,59.6652712589544,-5.68908267149966));
#34755=CARTESIAN_POINT('Ctrl Pts',(64.2590096296175,59.7765943064858,-5.68282789080342));
#34756=CARTESIAN_POINT('Ctrl Pts',(64.2633182272178,59.8882668059091,-5.67657311010718));
#34757=CARTESIAN_POINT('Ctrl Pts',(64.2632169517948,59.999945593479,-5.67031832941094));
#34758=CARTESIAN_POINT('Ctrl Pts',(64.2626973799646,60.005388464797,-6.07968167058906));
#34759=CARTESIAN_POINT('Ctrl Pts',(64.252811870065,58.9392739973195,-6.13934364288562));
#34760=CARTESIAN_POINT('Ctrl Pts',(63.8459813507535,57.8645461017925,-6.19900561518218));
#34761=CARTESIAN_POINT('Ctrl Pts',(63.1240241101926,57.0887733774513,-6.25866758747874));
#34762=CARTESIAN_POINT('Ctrl Pts',(62.1808346712192,56.0752775642175,-6.3366120127396));
#34763=CARTESIAN_POINT('Ctrl Pts',(60.6997965155868,55.5720293571637,-6.41455643800045));
#34764=CARTESIAN_POINT('Ctrl Pts',(59.3267917363085,55.7867187111922,-6.49250086326132));
#34765=CARTESIAN_POINT('Ctrl Pts',(58.6402893466693,55.8940633882065,-6.53147307589175));
#34766=CARTESIAN_POINT('Ctrl Pts',(57.9807953011187,56.1808924554913,-6.57044528852218));
#34767=CARTESIAN_POINT('Ctrl Pts',(57.4261727612217,56.6023844136342,-6.60941750115261));
#34768=CARTESIAN_POINT('Ctrl Pts',(56.8715502213248,57.023876371777,-6.64838971378304));
#34769=CARTESIAN_POINT('Ctrl Pts',(56.4217991870814,57.5800312207779,-6.68736192641346));
#34770=CARTESIAN_POINT('Ctrl Pts',(56.1299141849854,58.210937755608,-6.72633413904389));
#34771=CARTESIAN_POINT('Ctrl Pts',(55.8380291828894,58.841844290438,-6.76530635167432));
#34772=CARTESIAN_POINT('Ctrl Pts',(55.7040102129408,59.5475025110972,-6.80427856430475));
#34773=CARTESIAN_POINT('Ctrl Pts',(55.7435430368397,60.2424382218237,-6.84325077693518));
#34774=CARTESIAN_POINT('Ctrl Pts',(55.7830758607386,60.9373739325502,-6.88222298956561));
#34775=CARTESIAN_POINT('Ctrl Pts',(55.9961604784851,61.6215871333439,-6.92119520219604));
#34776=CARTESIAN_POINT('Ctrl Pts',(56.3577826916297,62.2158268315062,-6.96016741482647));
#34777=CARTESIAN_POINT('Ctrl Pts',(56.7194049047743,62.8100665296684,-6.9991396274569));
#34778=CARTESIAN_POINT('Ctrl Pts',(57.229564713317,63.3143327251992,-7.03811184008733));
#34779=CARTESIAN_POINT('Ctrl Pts',(57.8282806977002,63.6688083962819,-7.07708405271776));
#34780=CARTESIAN_POINT('Ctrl Pts',(58.4269966820833,64.0232840673647,-7.11605626534819));
#34781=CARTESIAN_POINT('Ctrl Pts',(59.114268842307,64.2279692139995,-7.15502847797862));
#34782=CARTESIAN_POINT('Ctrl Pts',(59.8093191206801,64.259056050085,-7.19400069060905));
#34783=CARTESIAN_POINT('Ctrl Pts',(60.5043693990532,64.2901428861706,-7.23297290323948));
#34784=CARTESIAN_POINT('Ctrl Pts',(61.2071977955758,64.147631411707,-7.27194511586991));
#34785=CARTESIAN_POINT('Ctrl Pts',(61.8351875016575,63.8481564596784,-7.31091732850034));
#34786=CARTESIAN_POINT('Ctrl Pts',(62.4631772077392,63.5486815076498,-7.34988954113077));
#34787=CARTESIAN_POINT('Ctrl Pts',(63.0163282233802,63.0922430780563,-7.3888617537612));
#34788=CARTESIAN_POINT('Ctrl Pts',(63.4296222037564,62.5325469979949,-7.42783396639163));
#34789=CARTESIAN_POINT('Ctrl Pts',(63.8429161841327,61.9728509179335,-7.46680617902206));
#34790=CARTESIAN_POINT('Ctrl Pts',(64.1163531292443,61.3098971874042,-7.50577839165249));
#34791=CARTESIAN_POINT('Ctrl Pts',(64.2177913481944,60.6215873296248,-7.54475060428292));
#34792=CARTESIAN_POINT('Ctrl Pts',(64.2480979428419,60.4159416857293,-7.55639429305164));
#34793=CARTESIAN_POINT('Ctrl Pts',(64.2630514303516,60.2080326800812,-7.56803798182035));
#34794=CARTESIAN_POINT('Ctrl Pts',(64.2628730117989,60.0000978162778,-7.57968167058906));
#34795=CARTESIAN_POINT('Origin',(60.,60.,-6.));
#34796=CARTESIAN_POINT('',(64.2632129797225,60.0000762878951,-9.07968167058906));
#34797=CARTESIAN_POINT('',(64.2626696975502,60.0000007546914,-8.67031832941094));
#34798=CARTESIAN_POINT('',(64.263,60.,-6.));
#34799=CARTESIAN_POINT('',(56.7766472160421,62.7898325810254,-10.));
#34800=CARTESIAN_POINT('Ctrl Pts',(64.2632129797225,60.0000762878951,-9.07968167058906));
#34801=CARTESIAN_POINT('Ctrl Pts',(64.2627031079153,59.3936235463162,-9.11364895864636));
#34802=CARTESIAN_POINT('Ctrl Pts',(64.1318733360967,58.7869579650774,-9.14761624670367));
#34803=CARTESIAN_POINT('Ctrl Pts',(63.8808238664535,58.2349684131022,-9.18158353476097));
#34804=CARTESIAN_POINT('Ctrl Pts',(63.5927834054316,57.6016457247243,-9.2205557473914));
#34805=CARTESIAN_POINT('Ctrl Pts',(63.1464855503109,57.0402986448989,-9.25952796002183));
#34806=CARTESIAN_POINT('Ctrl Pts',(62.5943907357823,56.6169137625735,-9.29850017265227));
#34807=CARTESIAN_POINT('Ctrl Pts',(62.0422959212538,56.1935288802482,-9.3374723852827));
#34808=CARTESIAN_POINT('Ctrl Pts',(61.3844041473173,55.908106195423,-9.37644459791312));
#34809=CARTESIAN_POINT('Ctrl Pts',(60.6980457486418,55.7941882630383,-9.41541681054355));
#34810=CARTESIAN_POINT('Ctrl Pts',(60.0116873499663,55.6802703306536,-9.45438902317398));
#34811=CARTESIAN_POINT('Ctrl Pts',(59.2968623265517,55.7378571507094,-9.49336123580441));
#34812=CARTESIAN_POINT('Ctrl Pts',(58.6375973357764,55.9601951486079,-9.53233344843484));
#34813=CARTESIAN_POINT('Ctrl Pts',(57.9783323450012,56.1825331465064,-9.57130566106527));
#34814=CARTESIAN_POINT('Ctrl Pts',(57.3746273868654,56.5696223222476,-9.6102778736957));
#34815=CARTESIAN_POINT('Ctrl Pts',(56.8974397908448,57.0759277155521,-9.64925008632613));
#34816=CARTESIAN_POINT('Ctrl Pts',(56.4202521948243,57.5822331088567,-9.68822229895656));
#34817=CARTESIAN_POINT('Ctrl Pts',(56.069581960919,58.2077547197246,-9.72719451158699));
#34818=CARTESIAN_POINT('Ctrl Pts',(55.8866652329043,58.8790351869383,-9.76616672421742));
#34819=CARTESIAN_POINT('Ctrl Pts',(55.7037485048897,59.550315654152,-9.80513893684785));
#34820=CARTESIAN_POINT('Ctrl Pts',(55.6885852827656,60.2673549777114,-9.84411114947828));
#34821=CARTESIAN_POINT('Ctrl Pts',(55.8429524134795,60.9456840068003,-9.88308336210871));
#34822=CARTESIAN_POINT('Ctrl Pts',(55.9973195441935,61.6240130358892,-9.92205557473914));
#34823=CARTESIAN_POINT('Ctrl Pts',(56.3212170277455,62.2636317705077,-9.96102778736957));
#34824=CARTESIAN_POINT('Ctrl Pts',(56.7766472160421,62.7898325810254,-10.));
#34825=CARTESIAN_POINT('',(63.2235668510161,62.7899187021734,-10.));
#34826=CARTESIAN_POINT('Origin',(60.,60.,-10.));
#34827=CARTESIAN_POINT('Ctrl Pts',(63.2235668510161,62.7899187021734,-10.));
#34828=CARTESIAN_POINT('Ctrl Pts',(62.8262375922137,63.2482129590446,-9.96602721186203));
#34829=CARTESIAN_POINT('Ctrl Pts',(62.3301928947912,63.6213495469796,-9.93205442372405));
#34830=CARTESIAN_POINT('Ctrl Pts',(61.7790228005731,63.8744287531187,-9.89808163558608));
#34831=CARTESIAN_POINT('Ctrl Pts',(61.1467426939136,64.1647510132151,-9.85910942295565));
#34832=CARTESIAN_POINT('Ctrl Pts',(60.4419189254527,64.2970807216377,-9.82013721032522));
#34833=CARTESIAN_POINT('Ctrl Pts',(59.7473945403606,64.2558578814904,-9.78116499769479));
#34834=CARTESIAN_POINT('Ctrl Pts',(59.0528701552686,64.2146350413431,-9.74219278506436));
#34835=CARTESIAN_POINT('Ctrl Pts',(58.3686451535453,63.999859652626,-9.70322057243393));
#34836=CARTESIAN_POINT('Ctrl Pts',(57.7751487629232,63.636779812551,-9.6642483598035));
#34837=CARTESIAN_POINT('Ctrl Pts',(57.1816523723011,63.2736999724761,-9.62527614717307));
#34838=CARTESIAN_POINT('Ctrl Pts',(56.6788845927801,62.7623156810432,-9.58630393454264));
#34839=CARTESIAN_POINT('Ctrl Pts',(56.3259418994758,62.1627361892336,-9.54733172191221));
#34840=CARTESIAN_POINT('Ctrl Pts',(55.9729992061715,61.563156697424,-9.50835950928178));
#34841=CARTESIAN_POINT('Ctrl Pts',(55.769881599084,60.8753820052377,-9.46938729665136));
#34842=CARTESIAN_POINT('Ctrl Pts',(55.7404649362495,60.1802567469978,-9.43041508402093));
#34843=CARTESIAN_POINT('Ctrl Pts',(55.711048273415,59.4851314887579,-9.3914428713905));
#34844=CARTESIAN_POINT('Ctrl Pts',(55.8553325548336,58.7826556644645,-9.35247065876007));
#34845=CARTESIAN_POINT('Ctrl Pts',(56.1563577258025,58.1554011721684,-9.31349844612963));
#34846=CARTESIAN_POINT('Ctrl Pts',(56.4573828967714,57.5281466798722,-9.2745262334992));
#34847=CARTESIAN_POINT('Ctrl Pts',(56.9151489572907,56.9761135195733,-9.23555402086877));
#34848=CARTESIAN_POINT('Ctrl Pts',(57.4758481529971,56.5641902504204,-9.19658180823834));
#34849=CARTESIAN_POINT('Ctrl Pts',(58.0365473487036,56.1522669812675,-9.15760959560791));
#34850=CARTESIAN_POINT('Ctrl Pts',(58.7001796795971,55.8804536032608,-9.11863738297749));
#34851=CARTESIAN_POINT('Ctrl Pts',(59.3887387820797,55.7807002126255,-9.07966517034706));
#34852=CARTESIAN_POINT('Ctrl Pts',(60.0772978845623,55.6809468219902,-9.04069295771663));
#34853=CARTESIAN_POINT('Ctrl Pts',(60.7907837586341,55.7532534187264,-9.00172074508619));
#34854=CARTESIAN_POINT('Ctrl Pts',(61.4453301273351,55.9891208068635,-8.96274853245576));
#34855=CARTESIAN_POINT('Ctrl Pts',(62.0998764960362,56.2249881950005,-8.92377631982533));
#34856=CARTESIAN_POINT('Ctrl Pts',(62.6954833593665,56.6244163745384,-8.88480410719491));
#34857=CARTESIAN_POINT('Ctrl Pts',(63.1621403861375,57.1404547199397,-8.84583189456448));
#34858=CARTESIAN_POINT('Ctrl Pts',(63.6287974129085,57.6564930653411,-8.80685968193405));
#34859=CARTESIAN_POINT('Ctrl Pts',(63.9665046031202,58.2891415766059,-8.76788746930362));
#34860=CARTESIAN_POINT('Ctrl Pts',(64.1355664178555,58.9640360217668,-8.72891525667319));
#34861=CARTESIAN_POINT('Ctrl Pts',(64.2202977532714,59.3022833527375,-8.70938294758577));
#34862=CARTESIAN_POINT('Ctrl Pts',(64.2626675734433,59.6511423104289,-8.68985063849836));
#34863=CARTESIAN_POINT('Ctrl Pts',(64.2626696975502,60.0000007546914,-8.67031832941094));
#34864=CARTESIAN_POINT('Origin',(60.,60.,-13.3123464956316));
#34865=CARTESIAN_POINT('',(65.0994142723023,60.0000080970367,-3.68765350436841));
#34866=CARTESIAN_POINT('',(65.0991104422254,59.9998849527226,-3.56234649563159));
#34867=CARTESIAN_POINT('',(65.099,59.9999999999999,-13.3123464956316));
#34868=CARTESIAN_POINT('',(56.3967816198432,63.607855083689,-3.));
#34869=CARTESIAN_POINT('Ctrl Pts',(65.0991104422254,59.9998849527226,-3.56234649563159));
#34870=CARTESIAN_POINT('Ctrl Pts',(65.098461631149,60.6739141965835,-3.53078651427611));
#34871=CARTESIAN_POINT('Ctrl Pts',(64.7978132036202,62.1808417610638,-3.46025432029021));
#34872=CARTESIAN_POINT('Ctrl Pts',(63.3555842661093,64.1119168678935,-3.35074991367387));
#34873=CARTESIAN_POINT('Ctrl Pts',(61.027044706866,65.2070699669712,-3.23383327578258));
#34874=CARTESIAN_POINT('Ctrl Pts',(58.4567442007043,65.0779746991923,-3.11691663789129));
#34875=CARTESIAN_POINT('Ctrl Pts',(56.9857510552448,64.1960675938266,-3.03897221263043));
#34876=CARTESIAN_POINT('Ctrl Pts',(56.3967816198432,63.6078550836889,-3.));
#34877=CARTESIAN_POINT('',(55.0736213347631,61.3165318688511,-3.));
#34878=CARTESIAN_POINT('Origin',(60.,60.,-3.));
#34879=CARTESIAN_POINT('Ctrl Pts',(65.0994142723023,60.0000080970367,-3.68765350436841));
#34880=CARTESIAN_POINT('Ctrl Pts',(65.0994150596659,60.0082074395616,-3.68726952086906));
#34881=CARTESIAN_POINT('Ctrl Pts',(65.097429063898,60.8485945549625,-3.64791332473928));
#34882=CARTESIAN_POINT('Ctrl Pts',(64.6714138007994,62.5191327746011,-3.56958491597908));
#34883=CARTESIAN_POINT('Ctrl Pts',(62.93732429588,64.4204364118546,-3.45266827808779));
#34884=CARTESIAN_POINT('Ctrl Pts',(60.5127057455321,65.2825431684356,-3.3357516401965));
#34885=CARTESIAN_POINT('Ctrl Pts',(57.967548471337,64.9027852181516,-3.2188350023052));
#34886=CARTESIAN_POINT('Ctrl Pts',(55.988614157022,63.4359554976302,-3.10691778890638));
#34887=CARTESIAN_POINT('Ctrl Pts',(55.2615313835496,62.0172737121676,-3.03397278813797));
#34888=CARTESIAN_POINT('Ctrl Pts',(55.0736213347631,61.3165318688511,-3.));
#34889=CARTESIAN_POINT('Origin',(60.,60.,-13.3123464956316));
#34890=CARTESIAN_POINT('',(65.0992594973497,59.9999349240322,-5.18765350436841));
#34891=CARTESIAN_POINT('',(65.0987279539713,59.9999119474263,-5.06234649563159));
#34892=CARTESIAN_POINT('',(65.099,59.9999999999999,-13.3123464956316));
#34893=CARTESIAN_POINT('Ctrl Pts',(65.0987279539713,59.9999119474263,-5.06234649563159));
#34894=CARTESIAN_POINT('Ctrl Pts',(65.0983788696902,60.5322706383878,-5.0374252784717));
#34895=CARTESIAN_POINT('Ctrl Pts',(64.8854638827286,61.8974113431707,-4.97353184868138));
#34896=CARTESIAN_POINT('Ctrl Pts',(63.6865889794253,63.8180111190031,-4.87066620626063));
#34897=CARTESIAN_POINT('Ctrl Pts',(61.4572740950116,65.1033792767411,-4.75374956836934));
#34898=CARTESIAN_POINT('Ctrl Pts',(58.8853714589078,65.189001781766,-4.63683293047805));
#34899=CARTESIAN_POINT('Ctrl Pts',(56.5755050441849,64.0547463443016,-4.51991629258676));
#34900=CARTESIAN_POINT('Ctrl Pts',(55.0706998168725,61.9672654489506,-4.40299965469547));
#34901=CARTESIAN_POINT('Ctrl Pts',(54.7247182017831,59.4173019594712,-4.28608301680418));
#34902=CARTESIAN_POINT('Ctrl Pts',(55.6188973320329,57.0043245192968,-4.16916637891289));
#34903=CARTESIAN_POINT('Ctrl Pts',(57.5430244185373,55.2955969820173,-4.0522497410216));
#34904=CARTESIAN_POINT('Ctrl Pts',(60.0447608866429,54.6928229271066,-3.93533310313032));
#34905=CARTESIAN_POINT('Ctrl Pts',(62.5359710846191,55.3377065632379,-3.81841646523902));
#34906=CARTESIAN_POINT('Ctrl Pts',(64.4310101049653,57.0786456054826,-3.70149982734774));
#34907=CARTESIAN_POINT('Ctrl Pts',(65.0540042126791,58.8510320510013,-3.61614317081192));
#34908=CARTESIAN_POINT('Ctrl Pts',(65.0992628231061,59.8415812900777,-3.56975872690654));
#34909=CARTESIAN_POINT('Ctrl Pts',(65.0991104422254,59.9998849527226,-3.56234649563159));
#34910=CARTESIAN_POINT('Ctrl Pts',(65.0992594973497,59.9999349240322,-5.18765350436841));
#34911=CARTESIAN_POINT('Ctrl Pts',(65.0986258598593,60.6986618672511,-5.15493607243422));
#34912=CARTESIAN_POINT('Ctrl Pts',(64.7810044222689,62.2301463492343,-5.0832464278696));
#34913=CARTESIAN_POINT('Ctrl Pts',(63.2955109480772,64.1603278329295,-4.97258457067455));
#34914=CARTESIAN_POINT('Ctrl Pts',(60.9510823128121,65.2214359708436,-4.85566793278326));
#34915=CARTESIAN_POINT('Ctrl Pts',(58.3831734117936,65.0550993752034,-4.73875129489197));
#34916=CARTESIAN_POINT('Ctrl Pts',(56.1953122098592,63.7003384596412,-4.62183465700068));
#34917=CARTESIAN_POINT('Ctrl Pts',(54.9019142936214,61.4756811820325,-4.50491801910939));
#34918=CARTESIAN_POINT('Ctrl Pts',(54.8070090801581,58.9041019292639,-4.3880013812181));
#34919=CARTESIAN_POINT('Ctrl Pts',(55.9329235426593,56.5901588022821,-4.27108474332681));
#34920=CARTESIAN_POINT('Ctrl Pts',(58.0149603175651,55.0778303762239,-4.15416810543552));
#34921=CARTESIAN_POINT('Ctrl Pts',(60.5636590493342,54.7226500811105,-4.03725146754424));
#34922=CARTESIAN_POINT('Ctrl Pts',(62.9798472108349,55.6081160860788,-3.92033482965294));
#34923=CARTESIAN_POINT('Ctrl Pts',(64.6898720162157,57.5197664101291,-3.803802175261));
#34924=CARTESIAN_POINT('Ctrl Pts',(65.0993351465935,59.1760192834263,-3.72624173349949));
#34925=CARTESIAN_POINT('Ctrl Pts',(65.0994142723023,60.0000080970367,-3.68765350436841));
#34926=CARTESIAN_POINT('Origin',(60.,60.,-13.3123464956316));
#34927=CARTESIAN_POINT('',(65.0984547190409,59.9994231828803,-6.68765350436841));
#34928=CARTESIAN_POINT('',(65.0986380343512,60.0064451752286,-6.56234649563159));
#34929=CARTESIAN_POINT('',(65.099,59.9999999999999,-13.3123464956316));
#34930=CARTESIAN_POINT('Ctrl Pts',(65.0986380343512,60.0064451752286,-6.56234649563159));
#34931=CARTESIAN_POINT('Ctrl Pts',(65.1022613453585,60.3972054217194,-6.54406404266729));
#34932=CARTESIAN_POINT('Ctrl Pts',(64.8866739179056,62.4488199389438,-6.44783716444213));
#34933=CARTESIAN_POINT('Ctrl Pts',(62.7388658113806,64.8816655541704,-6.31263807358654));
#34934=CARTESIAN_POINT('Ctrl Pts',(59.3187584788532,65.2585195543855,-6.15674922306482));
#34935=CARTESIAN_POINT('Ctrl Pts',(56.9266335796149,64.3285139675122,-6.03983258517353));
#34936=CARTESIAN_POINT('Ctrl Pts',(55.2511526541055,62.3700211957414,-5.92291594728224));
#34937=CARTESIAN_POINT('Ctrl Pts',(54.6947972197688,59.8594460319768,-5.80599930939095));
#34938=CARTESIAN_POINT('Ctrl Pts',(55.3843760081973,57.3795654934784,-5.68908267149966));
#34939=CARTESIAN_POINT('Ctrl Pts',(57.1596209351837,55.5168092181914,-5.57216603360837));
#34940=CARTESIAN_POINT('Ctrl Pts',(59.6023370896801,54.7074973445116,-5.45524939571708));
#34941=CARTESIAN_POINT('Ctrl Pts',(62.138664673409,55.1426278237003,-5.33833275782579));
#34942=CARTESIAN_POINT('Ctrl Pts',(64.1721578471653,56.7195645494213,-5.2214161199345));
#34943=CARTESIAN_POINT('Ctrl Pts',(65.0004645732374,58.5672219271665,-5.1294206992031));
#34944=CARTESIAN_POINT('Ctrl Pts',(65.0989247734775,59.6997592900575,-5.07639749110213));
#34945=CARTESIAN_POINT('Ctrl Pts',(65.0987279539713,59.9999119474263,-5.06234649563159));
#34946=CARTESIAN_POINT('Ctrl Pts',(65.0984547190409,59.9994231828803,-6.68765350436841));
#34947=CARTESIAN_POINT('Ctrl Pts',(65.097455978134,60.5556872072211,-6.66157483662981));
#34948=CARTESIAN_POINT('Ctrl Pts',(64.8688835602887,61.943672278096,-6.59652395626078));
#34949=CARTESIAN_POINT('Ctrl Pts',(63.1773281761085,64.6083211110609,-6.45352865063088));
#34950=CARTESIAN_POINT('Ctrl Pts',(58.6661397561353,65.8440762220129,-6.25866758747874));
#34951=CARTESIAN_POINT('Ctrl Pts',(54.3971986841152,62.1309686655549,-6.02483431169616));
#34952=CARTESIAN_POINT('Ctrl Pts',(54.9957816802558,57.4920452935348,-5.82997324854401));
#34953=CARTESIAN_POINT('Ctrl Pts',(57.6170719268681,55.2631467174745,-5.67408439802229));
#34954=CARTESIAN_POINT('Ctrl Pts',(60.1194257717932,54.6927078330755,-5.557167760131));
#34955=CARTESIAN_POINT('Ctrl Pts',(62.6046743394157,55.3756921094109,-5.44025112223971));
#34956=CARTESIAN_POINT('Ctrl Pts',(64.4724884051625,57.1431171033903,-5.32333448434842));
#34957=CARTESIAN_POINT('Ctrl Pts',(65.062116481349,58.900523352424,-5.23913527839132));
#34958=CARTESIAN_POINT('Ctrl Pts',(65.0993806334936,59.8663552529511,-5.19390828506465));
#34959=CARTESIAN_POINT('Ctrl Pts',(65.0992594973497,59.9999349240322,-5.18765350436841));
#34960=CARTESIAN_POINT('Origin',(60.,60.,-13.3123464956316));
#34961=CARTESIAN_POINT('',(65.0986049232486,60.0000009026908,-8.18765350436841));
#34962=CARTESIAN_POINT('',(65.098848108647,60.0001169986396,-8.06234649563159));
#34963=CARTESIAN_POINT('',(65.099,59.9999999999999,-13.3123464956316));
#34964=CARTESIAN_POINT('Ctrl Pts',(65.098848108647,60.0001169986396,-8.06234649563159));
#34965=CARTESIAN_POINT('Ctrl Pts',(65.0990615161536,60.2488291427947,-8.05070280686288));
#34966=CARTESIAN_POINT('Ctrl Pts',(65.0213100551162,61.3298631785982,-8.00008690546373));
#34967=CARTESIAN_POINT('Ctrl Pts',(64.2694756368211,63.1527018302866,-7.91049879143416));
#34968=CARTESIAN_POINT('Ctrl Pts',(62.2845938431877,64.7905481022763,-7.79358215354287));
#34969=CARTESIAN_POINT('Ctrl Pts',(59.7626219966935,65.301924603536,-7.67666551565158));
#34970=CARTESIAN_POINT('Ctrl Pts',(57.2964708742581,64.5674491899606,-7.55974887776029));
#34971=CARTESIAN_POINT('Ctrl Pts',(55.4658552065881,62.7579816804522,-7.442832239869));
#34972=CARTESIAN_POINT('Ctrl Pts',(54.7012398189108,60.3028070774634,-7.32591560197771));
#34973=CARTESIAN_POINT('Ctrl Pts',(55.1821425126253,57.7706809218396,-7.20899896408643));
#34974=CARTESIAN_POINT('Ctrl Pts',(56.7959922829326,55.7750204186338,-7.09208232619513));
#34975=CARTESIAN_POINT('Ctrl Pts',(59.9512914978166,54.4027085123842,-6.93619347567342));
#34976=CARTESIAN_POINT('Ctrl Pts',(63.9644744788023,55.7663648990069,-6.75961486548557));
#34977=CARTESIAN_POINT('Ctrl Pts',(65.0868139163643,58.7312592334816,-6.62200846792815));
#34978=CARTESIAN_POINT('Ctrl Pts',(65.0986380343512,60.0064451752286,-6.56234649563159));
#34979=CARTESIAN_POINT('Ctrl Pts',(65.0986049232486,60.0000009026908,-8.18765350436841));
#34980=CARTESIAN_POINT('Ctrl Pts',(65.098607451886,60.4152985173152,-8.1682136008254));
#34981=CARTESIAN_POINT('Ctrl Pts',(64.9477827347253,61.6631636070336,-8.10980148465196));
#34982=CARTESIAN_POINT('Ctrl Pts',(63.9406234579031,63.5552235763429,-8.01241715584808));
#34983=CARTESIAN_POINT('Ctrl Pts',(61.8050635087969,64.9909811652868,-7.89550051795679));
#34984=CARTESIAN_POINT('Ctrl Pts',(59.2451498198411,65.2534097530527,-7.7785838800655));
#34985=CARTESIAN_POINT('Ctrl Pts',(56.8627001620859,64.2808297817029,-7.66166724217421));
#34986=CARTESIAN_POINT('Ctrl Pts',(55.2177796069362,62.3018527370191,-7.54475060428292));
#34987=CARTESIAN_POINT('Ctrl Pts',(54.6971392652592,59.7817817811634,-7.42783396639163));
#34988=CARTESIAN_POINT('Ctrl Pts',(55.4230712085558,57.3129118130677,-7.31091732850034));
#34989=CARTESIAN_POINT('Ctrl Pts',(57.2251429658425,55.4759618040439,-7.19400069060905));
#34990=CARTESIAN_POINT('Ctrl Pts',(59.6792193933806,54.7020984074429,-7.07708405271776));
#34991=CARTESIAN_POINT('Ctrl Pts',(62.2094284211809,55.174716747074,-6.96016741482647));
#34992=CARTESIAN_POINT('Ctrl Pts',(64.2186721193591,56.7795408043723,-6.84325077693519));
#34993=CARTESIAN_POINT('Ctrl Pts',(65.0118140711112,58.6182636268587,-6.75241280678249));
#34994=CARTESIAN_POINT('Ctrl Pts',(65.0989485061794,59.7244008833735,-6.70054704926024));
#34995=CARTESIAN_POINT('Ctrl Pts',(65.0984547190409,59.9994231828803,-6.68765350436841));
#34996=CARTESIAN_POINT('Origin',(60.,60.,-13.3123464956316));
#34997=CARTESIAN_POINT('',(65.0987893697715,60.0001196244759,-9.68765350436842));
#34998=CARTESIAN_POINT('',(65.0992547463301,60.0000912484111,-9.56234649563159));
#34999=CARTESIAN_POINT('',(65.099,59.9999999999999,-13.3123464956316));
#35000=CARTESIAN_POINT('',(61.322884965569,55.0755938055567,-10.));
#35001=CARTESIAN_POINT('Ctrl Pts',(61.322884965569,55.0755938055567,-10.));
#35002=CARTESIAN_POINT('Ctrl Pts',(62.1267766598728,55.2915500435982,-9.96102778736957));
#35003=CARTESIAN_POINT('Ctrl Pts',(63.6260271731292,56.1245140078271,-9.88308336210872));
#35004=CARTESIAN_POINT('Ctrl Pts',(64.8700259230263,58.049261551967,-9.77896786356485));
#35005=CARTESIAN_POINT('Ctrl Pts',(65.0983672436226,59.4410930803254,-9.71382457765142));
#35006=CARTESIAN_POINT('Ctrl Pts',(65.0987893697715,60.0001196244759,-9.68765350436842));
#35007=CARTESIAN_POINT('',(58.6769607112098,55.0753649997562,-10.));
#35008=CARTESIAN_POINT('Origin',(60.,60.,-10.));
#35009=CARTESIAN_POINT('Ctrl Pts',(58.6769607112098,55.0753649997562,-10.));
#35010=CARTESIAN_POINT('Ctrl Pts',(59.3777759733541,54.8877289534041,-9.96602721186202));
#35011=CARTESIAN_POINT('Ctrl Pts',(60.9699318229197,54.808060215244,-9.89308221109362));
#35012=CARTESIAN_POINT('Ctrl Pts',(63.2297107806181,55.7884527399271,-9.78116499769479));
#35013=CARTESIAN_POINT('Ctrl Pts',(64.7626147903817,57.7165175505922,-9.66925328437663));
#35014=CARTESIAN_POINT('Ctrl Pts',(65.0986448855876,59.2747094681366,-9.5963137836889));
#35015=CARTESIAN_POINT('Ctrl Pts',(65.0992547463301,60.0000912484111,-9.56234649563159));
#35016=CARTESIAN_POINT('Origin',(-60.,60.,-6.));
#35017=CARTESIAN_POINT('',(-55.7372273834134,59.9999263798756,-4.57968167058906));
#35018=CARTESIAN_POINT('',(-55.7366536686051,60.0000067695234,-4.17031832941094));
#35019=CARTESIAN_POINT('',(-55.737,60.,-6.));
#35020=CARTESIAN_POINT('',(-59.1956105045055,55.8135783132205,-3.));
#35021=CARTESIAN_POINT('Ctrl Pts',(-55.7366536686051,60.0000067695234,-4.17031832941094));
#35022=CARTESIAN_POINT('Ctrl Pts',(-55.7366530103325,60.0068617993376,-4.16993434591159));
#35023=CARTESIAN_POINT('Ctrl Pts',(-55.7366692100737,60.0137168260256,-4.16955036241224));
#35024=CARTESIAN_POINT('Ctrl Pts',(-55.7367022869973,60.0205717712724,-4.16916637891289));
#35025=CARTESIAN_POINT('Ctrl Pts',(-55.74005941276,60.7163110001195,-4.13019416628246));
#35026=CARTESIAN_POINT('Ctrl Pts',(-55.9172706415258,61.4112112921654,-4.09122195365204));
#35027=CARTESIAN_POINT('Ctrl Pts',(-56.2475061025821,62.0235910770971,-4.05224974102161));
#35028=CARTESIAN_POINT('Ctrl Pts',(-56.5777415636384,62.6359708620289,-4.01327752839118));
#35029=CARTESIAN_POINT('Ctrl Pts',(-57.0610012569851,63.1658301398464,-3.97430531576075));
#35030=CARTESIAN_POINT('Ctrl Pts',(-57.6404799899334,63.5508866362206,-3.93533310313031));
#35031=CARTESIAN_POINT('Ctrl Pts',(-58.2199587228817,63.9359431325947,-3.89636089049988));
#35032=CARTESIAN_POINT('Ctrl Pts',(-58.8956564954316,64.1761968475256,-3.85738867786946));
#35033=CARTESIAN_POINT('Ctrl Pts',(-59.5881502605052,64.2434078352681,-3.81841646523903));
#35034=CARTESIAN_POINT('Ctrl Pts',(-60.2806440255789,64.3106188230106,-3.7794442526086));
#35035=CARTESIAN_POINT('Ctrl Pts',(-60.9899337831764,64.2047870835648,-3.74047203997817));
#35036=CARTESIAN_POINT('Ctrl Pts',(-61.6326432518039,63.9383513901597,-3.70149982734774));
#35037=CARTESIAN_POINT('Ctrl Pts',(-62.2753527204313,63.6719156967547,-3.66252761471731));
#35038=CARTESIAN_POINT('Ctrl Pts',(-62.8514819000888,63.2448760493903,-3.62355540208688));
#35039=CARTESIAN_POINT('Ctrl Pts',(-63.2933169215645,62.7074312082618,-3.58458318945645));
#35040=CARTESIAN_POINT('Ctrl Pts',(-63.7351519430401,62.1699863671332,-3.54561097682602));
#35041=CARTESIAN_POINT('Ctrl Pts',(-64.0426928063339,61.5221363322404,-3.50663876419559));
#35042=CARTESIAN_POINT('Ctrl Pts',(-64.1797749455836,60.8400271011362,-3.46766655156516));
#35043=CARTESIAN_POINT('Ctrl Pts',(-64.3168570848332,60.1579178700319,-3.42869433893473));
#35044=CARTESIAN_POINT('Ctrl Pts',(-64.2834805000387,59.4415494427162,-3.3897221263043));
#35045=CARTESIAN_POINT('Ctrl Pts',(-64.0836009653472,58.7751401645266,-3.35074991367387));
#35046=CARTESIAN_POINT('Ctrl Pts',(-63.8837214306558,58.1087308863369,-3.31177770104344));
#35047=CARTESIAN_POINT('Ctrl Pts',(-63.5173389460674,57.4922807572733,-3.27280548841301));
#35048=CARTESIAN_POINT('Ctrl Pts',(-63.0274513684703,56.9982299650024,-3.23383327578258));
#35049=CARTESIAN_POINT('Ctrl Pts',(-62.5375637908732,56.5041791727314,-3.19486106315215));
#35050=CARTESIAN_POINT('Ctrl Pts',(-61.9241711202674,56.1325277172532,-3.15588885052172));
#35051=CARTESIAN_POINT('Ctrl Pts',(-61.2595373895626,55.9270490755113,-3.11691663789129));
#35052=CARTESIAN_POINT('Ctrl Pts',(-60.5949036588578,55.7215704337695,-3.07794442526086));
#35053=CARTESIAN_POINT('Ctrl Pts',(-59.8790288680541,55.6822646057641,-3.03897221263043));
#35054=CARTESIAN_POINT('Ctrl Pts',(-59.1956105045055,55.8135783132205,-3.));
#35055=CARTESIAN_POINT('',(-55.972076043732,61.3967314412509,-3.00000000000001));
#35056=CARTESIAN_POINT('Origin',(-60.,60.,-3.));
#35057=CARTESIAN_POINT('',(-55.7369075951045,59.9999038083371,-3.07968167058906));
#35058=CARTESIAN_POINT('Ctrl Pts',(-55.972076043732,61.3967314412509,-3.00000000000001));
#35059=CARTESIAN_POINT('Ctrl Pts',(-55.8170962766014,60.9485583511405,-3.02656055686302));
#35060=CARTESIAN_POINT('Ctrl Pts',(-55.7373641065468,60.4741561734832,-3.05312111372604));
#35061=CARTESIAN_POINT('Ctrl Pts',(-55.7369075951045,59.9999038083371,-3.07968167058906));
#35062=CARTESIAN_POINT('',(-55.737,60.,-2.));
#35063=CARTESIAN_POINT('',(-55.737,60.,-6.));
#35064=CARTESIAN_POINT('Origin',(-60.,60.,-2.));
#35065=CARTESIAN_POINT('Ctrl Pts',(-55.7369075951045,59.9999038083371,-3.07968167058906));
#35066=CARTESIAN_POINT('Ctrl Pts',(-55.7367801968573,59.8675546173436,-3.08709390186401));
#35067=CARTESIAN_POINT('Ctrl Pts',(-55.7428267531846,59.7352170936848,-3.09450613313896));
#35068=CARTESIAN_POINT('Ctrl Pts',(-55.7551348091079,59.6034645506898,-3.10191836441391));
#35069=CARTESIAN_POINT('Ctrl Pts',(-55.8198484094689,58.9107327767164,-3.14089057704434));
#35070=CARTESIAN_POINT('Ctrl Pts',(-56.0576594161103,58.2341726296972,-3.17986278967477));
#35071=CARTESIAN_POINT('Ctrl Pts',(-56.4406216430255,57.6533082825818,-3.2188350023052));
#35072=CARTESIAN_POINT('Ctrl Pts',(-56.8235838699406,57.0724439354665,-3.25780721493563));
#35073=CARTESIAN_POINT('Ctrl Pts',(-57.3516973171296,56.5872753882551,-3.29677942756606));
#35074=CARTESIAN_POINT('Ctrl Pts',(-57.9628818847596,56.254832352553,-3.33575164019649));
#35075=CARTESIAN_POINT('Ctrl Pts',(-58.5740664523896,55.9223893168508,-3.37472385282692));
#35076=CARTESIAN_POINT('Ctrl Pts',(-59.2683221404606,55.742671792658,-3.41369606545735));
#35077=CARTESIAN_POINT('Ctrl Pts',(-59.9640445684598,55.7368041996945,-3.45266827808778));
#35078=CARTESIAN_POINT('Ctrl Pts',(-60.659766996459,55.730936606731,-3.49164049071821));
#35079=CARTESIAN_POINT('Ctrl Pts',(-61.3569561643863,55.8989189449969,-3.53061270334864));
#35080=CARTESIAN_POINT('Ctrl Pts',(-61.9736606357888,56.2210060021645,-3.56958491597907));
#35081=CARTESIAN_POINT('Ctrl Pts',(-62.5903651071913,56.543093059332,-3.6085571286095));
#35082=CARTESIAN_POINT('Ctrl Pts',(-63.1265848820691,57.0192848354013,-3.64752934123993));
#35083=CARTESIAN_POINT('Ctrl Pts',(-63.5192906276179,57.5936075318196,-3.68650155387036));
#35084=CARTESIAN_POINT('Ctrl Pts',(-63.9119963731668,58.1679302282379,-3.72547376650079));
#35085=CARTESIAN_POINT('Ctrl Pts',(-64.1611880893868,58.8403838450051,-3.76444597913122));
#35086=CARTESIAN_POINT('Ctrl Pts',(-64.2375745063077,59.5319252415894,-3.80341819176165));
#35087=CARTESIAN_POINT('Ctrl Pts',(-64.3139609232287,60.2234666381736,-3.84239040439208));
#35088=CARTESIAN_POINT('Ctrl Pts',(-64.2175420408506,60.9340958145749,-3.88136261702251));
#35089=CARTESIAN_POINT('Ctrl Pts',(-63.9596514602529,61.5802821811732,-3.92033482965294));
#35090=CARTESIAN_POINT('Ctrl Pts',(-63.7017608796552,62.2264685477715,-3.95930704228337));
#35091=CARTESIAN_POINT('Ctrl Pts',(-63.2823986008379,62.8082121045669,-3.9982792549138));
#35092=CARTESIAN_POINT('Ctrl Pts',(-62.7508582516328,63.2571322255563,-4.03725146754423));
#35093=CARTESIAN_POINT('Ctrl Pts',(-62.2193179024276,63.7060523465458,-4.07622368017466));
#35094=CARTESIAN_POINT('Ctrl Pts',(-61.5755994828347,64.0221490317292,-4.11519589280509));
#35095=CARTESIAN_POINT('Ctrl Pts',(-60.8953686608783,64.1682666450633,-4.15416810543552));
#35096=CARTESIAN_POINT('Ctrl Pts',(-60.2151378389219,64.3143842583974,-4.19314031806595));
#35097=CARTESIAN_POINT('Ctrl Pts',(-59.4983946146019,64.290522799882,-4.23211253069638));
#35098=CARTESIAN_POINT('Ctrl Pts',(-58.8293879277002,64.0994875219352,-4.27108474332681));
#35099=CARTESIAN_POINT('Ctrl Pts',(-58.1603812407985,63.9084522439884,-4.31005695595724));
#35100=CARTESIAN_POINT('Ctrl Pts',(-57.539111091315,63.5502431466101,-4.34902916858767));
#35101=CARTESIAN_POINT('Ctrl Pts',(-57.0386048919244,63.0669647139892,-4.3880013812181));
#35102=CARTESIAN_POINT('Ctrl Pts',(-56.5380986925339,62.5836862813682,-4.42697359384853));
#35103=CARTESIAN_POINT('Ctrl Pts',(-56.1583564432364,61.9753385135046,-4.46594580647896));
#35104=CARTESIAN_POINT('Ctrl Pts',(-55.9440135696077,61.313431507019,-4.50491801910939));
#35105=CARTESIAN_POINT('Ctrl Pts',(-55.8069496222504,60.8901676701744,-4.52983923626928));
#35106=CARTESIAN_POINT('Ctrl Pts',(-55.7375192334137,60.4450028927427,-4.55476045342917));
#35107=CARTESIAN_POINT('Ctrl Pts',(-55.7372273834134,59.9999263798756,-4.57968167058906));
#35108=CARTESIAN_POINT('Origin',(-60.,60.,-6.));
#35109=CARTESIAN_POINT('',(-55.7373026574226,60.0053877648092,-6.07968167058906));
#35110=CARTESIAN_POINT('',(-55.7367830248949,59.9999456221449,-5.67031832941094));
#35111=CARTESIAN_POINT('',(-55.737,60.,-6.));
#35112=CARTESIAN_POINT('Ctrl Pts',(-55.7367830248949,59.9999456221449,-5.67031832941094));
#35113=CARTESIAN_POINT('Ctrl Pts',(-55.7373127735992,60.5841136850818,-5.63760089747675));
#35114=CARTESIAN_POINT('Ctrl Pts',(-55.8585017386039,61.1684537659817,-5.60488346554256));
#35115=CARTESIAN_POINT('Ctrl Pts',(-56.0919563653973,61.7038522083462,-5.57216603360837));
#35116=CARTESIAN_POINT('Ctrl Pts',(-56.3700418634662,62.3416058676127,-5.53319382097794));
#35117=CARTESIAN_POINT('Ctrl Pts',(-56.807421080765,62.9099162482909,-5.49422160834751));
#35118=CARTESIAN_POINT('Ctrl Pts',(-57.3527858376896,63.3419273517729,-5.45524939571708));
#35119=CARTESIAN_POINT('Ctrl Pts',(-57.8981505946142,63.7739384552549,-5.41627718308665));
#35120=CARTESIAN_POINT('Ctrl Pts',(-58.5515008911646,64.0696502815408,-5.37730497045622));
#35121=CARTESIAN_POINT('Ctrl Pts',(-59.2359911490654,64.1943286820334,-5.33833275782579));
#35122=CARTESIAN_POINT('Ctrl Pts',(-59.9204814069662,64.319007082526,-5.29936054519536));
#35123=CARTESIAN_POINT('Ctrl Pts',(-60.6361116262173,64.2726520572252,-5.26038833256493));
#35124=CARTESIAN_POINT('Ctrl Pts',(-61.2987856077668,64.0607007393324,-5.2214161199345));
#35125=CARTESIAN_POINT('Ctrl Pts',(-61.9614595893163,63.8487494214396,-5.18244390730407));
#35126=CARTESIAN_POINT('Ctrl Pts',(-62.5711773331643,63.4712018109547,-5.14347169467364));
#35127=CARTESIAN_POINT('Ctrl Pts',(-63.0562596233642,62.9724419329156,-5.10449948204321));
#35128=CARTESIAN_POINT('Ctrl Pts',(-63.5413419135642,62.4736820548765,-5.06552726941278));
#35129=CARTESIAN_POINT('Ctrl Pts',(-63.9017887501161,61.8537099092833,-5.02655505678235));
#35130=CARTESIAN_POINT('Ctrl Pts',(-64.0952363607056,61.1853972915882,-4.98758284415192));
#35131=CARTESIAN_POINT('Ctrl Pts',(-64.2886839712951,60.5170846738932,-4.94861063152149));
#35132=CARTESIAN_POINT('Ctrl Pts',(-64.315132355922,59.8004315840964,-4.90963841889106));
#35133=CARTESIAN_POINT('Ctrl Pts',(-64.1714704483469,59.1196777821999,-4.87066620626063));
#35134=CARTESIAN_POINT('Ctrl Pts',(-64.0278085407718,58.4389239803035,-4.8316939936302));
#35135=CARTESIAN_POINT('Ctrl Pts',(-63.7140363409947,57.7940694663075,-4.79272178099977));
#35136=CARTESIAN_POINT('Ctrl Pts',(-63.267037057901,57.2609127834971,-4.75374956836934));
#35137=CARTESIAN_POINT('Ctrl Pts',(-62.8200377748072,56.7277561006868,-4.71477735573891));
#35138=CARTESIAN_POINT('Ctrl Pts',(-62.239811408397,56.3062972490623,-4.67580514310848));
#35139=CARTESIAN_POINT('Ctrl Pts',(-61.5945598762935,56.0460766292211,-4.63683293047805));
#35140=CARTESIAN_POINT('Ctrl Pts',(-60.9493083441901,55.78585600938,-4.59786071784762));
#35141=CARTESIAN_POINT('Ctrl Pts',(-60.2390316463936,55.6868736213223,-4.55888850521719));
#35142=CARTESIAN_POINT('Ctrl Pts',(-59.5472191102546,55.7607641871698,-4.51991629258676));
#35143=CARTESIAN_POINT('Ctrl Pts',(-58.8554065741155,55.8346547530174,-4.48094407995633));
#35144=CARTESIAN_POINT('Ctrl Pts',(-58.1820581996339,56.0814182727702,-4.4419718673259));
#35145=CARTESIAN_POINT('Ctrl Pts',(-57.6063222274869,56.4720491024142,-4.40299965469547));
#35146=CARTESIAN_POINT('Ctrl Pts',(-57.0305862553399,56.8626799320582,-4.36402744206504));
#35147=CARTESIAN_POINT('Ctrl Pts',(-56.5524626855275,57.3971780715933,-4.32505522943461));
#35148=CARTESIAN_POINT('Ctrl Pts',(-56.2281524120011,58.0127162241851,-4.28608301680418));
#35149=CARTESIAN_POINT('Ctrl Pts',(-55.9070374867832,58.6221896327487,-4.2474947876731));
#35150=CARTESIAN_POINT('Ctrl Pts',(-55.7367198213808,59.3111139873581,-4.20890655854202));
#35151=CARTESIAN_POINT('Ctrl Pts',(-55.7366536686051,60.0000067695234,-4.17031832941094));
#35152=CARTESIAN_POINT('Ctrl Pts',(-55.7372273834134,59.9999263798756,-4.57968167058906));
#35153=CARTESIAN_POINT('Ctrl Pts',(-55.7370628335439,59.7489848618022,-4.5937326660596));
#35154=CARTESIAN_POINT('Ctrl Pts',(-55.7588766741727,59.4980714020751,-4.60778366153014));
#35155=CARTESIAN_POINT('Ctrl Pts',(-55.8029386446782,59.2511271515956,-4.62183465700068));
#35156=CARTESIAN_POINT('Ctrl Pts',(-55.9251500913374,58.5661960477653,-4.66080686963111));
#35157=CARTESIAN_POINT('Ctrl Pts',(-56.2185164826157,57.9118000852124,-4.69977908226154));
#35158=CARTESIAN_POINT('Ctrl Pts',(-56.6485487572492,57.3648700713727,-4.73875129489197));
#35159=CARTESIAN_POINT('Ctrl Pts',(-57.0785810318826,56.817940057533,-4.7777235075224));
#35160=CARTESIAN_POINT('Ctrl Pts',(-57.6452791898711,56.3784759924065,-4.81669572015283));
#35161=CARTESIAN_POINT('Ctrl Pts',(-58.2820428030497,56.0981124513163,-4.85566793278326));
#35162=CARTESIAN_POINT('Ctrl Pts',(-58.9188064162282,55.817748910226,-4.89464014541369));
#35163=CARTESIAN_POINT('Ctrl Pts',(-59.6256354845968,55.696485893172,-4.93361235804411));
#35164=CARTESIAN_POINT('Ctrl Pts',(-60.3194206751,55.7486246935045,-4.97258457067455));
#35165=CARTESIAN_POINT('Ctrl Pts',(-61.0132058656032,55.8007634938371,-5.01155678330497));
#35166=CARTESIAN_POINT('Ctrl Pts',(-61.6939471782411,56.0263041115563,-5.05052899593541));
#35167=CARTESIAN_POINT('Ctrl Pts',(-62.2816822789534,56.3986329467664,-5.08950120856583));
#35168=CARTESIAN_POINT('Ctrl Pts',(-62.8694173796658,56.7709617819764,-5.12847342119627));
#35169=CARTESIAN_POINT('Ctrl Pts',(-63.3641462684527,57.2900788346774,-5.16744563382669));
#35170=CARTESIAN_POINT('Ctrl Pts',(-63.7075974300418,57.8951863058555,-5.20641784645712));
#35171=CARTESIAN_POINT('Ctrl Pts',(-64.051048591631,58.5002937770336,-5.24539005908755));
#35172=CARTESIAN_POINT('Ctrl Pts',(-64.2432220260225,59.1913916666888,-5.28436227171798));
#35173=CARTESIAN_POINT('Ctrl Pts',(-64.2617854331837,59.8867672128279,-5.32333448434841));
#35174=CARTESIAN_POINT('Ctrl Pts',(-64.280348840345,60.5821427589669,-5.36230669697884));
#35175=CARTESIAN_POINT('Ctrl Pts',(-64.1253022202761,61.2817959615897,-5.40127890960927));
#35176=CARTESIAN_POINT('Ctrl Pts',(-63.8143159016832,61.9045202861169,-5.4402511222397));
#35177=CARTESIAN_POINT('Ctrl Pts',(-63.5033295830904,62.5272446106442,-5.47922333487013));
#35178=CARTESIAN_POINT('Ctrl Pts',(-63.0364035659737,63.073040057076,-5.51819554750056));
#35179=CARTESIAN_POINT('Ctrl Pts',(-62.4696188635954,63.4755272987511,-5.55716776013099));
#35180=CARTESIAN_POINT('Ctrl Pts',(-61.9028341612172,63.8780145404261,-5.59613997276142));
#35181=CARTESIAN_POINT('Ctrl Pts',(-61.2361907735773,64.1371935773445,-5.63511218539185));
#35182=CARTESIAN_POINT('Ctrl Pts',(-60.5454485416163,64.2273981110301,-5.67408439802228));
#35183=CARTESIAN_POINT('Ctrl Pts',(-59.8547063096553,64.3176026447156,-5.71305661065271));
#35184=CARTESIAN_POINT('Ctrl Pts',(-59.1398652333731,64.2388326751683,-5.75202882328314));
#35185=CARTESIAN_POINT('Ctrl Pts',(-58.4907659763914,63.9908835405709,-5.79100103591357));
#35186=CARTESIAN_POINT('Ctrl Pts',(-57.1925674624281,63.4949852713762,-5.86894546117443));
#35187=CARTESIAN_POINT('Ctrl Pts',(-56.1573362256669,62.3223703419813,-5.94688988643529));
#35188=CARTESIAN_POINT('Ctrl Pts',(-55.8423909177357,60.9741913581959,-6.02483431169615));
#35189=CARTESIAN_POINT('Ctrl Pts',(-55.7685181197862,60.6579658067722,-6.04311676466045));
#35190=CARTESIAN_POINT('Ctrl Pts',(-55.7342734667231,60.3320812053717,-6.06139921762475));
#35191=CARTESIAN_POINT('Ctrl Pts',(-55.7373026574226,60.0053877648092,-6.07968167058906));
#35192=CARTESIAN_POINT('Origin',(-60.,60.,-6.));
#35193=CARTESIAN_POINT('',(-55.7371269276513,60.000097806567,-7.57968167058905));
#35194=CARTESIAN_POINT('',(-55.7374561790016,59.9995175300878,-7.17031832941094));
#35195=CARTESIAN_POINT('',(-55.737,60.,-6.));
#35196=CARTESIAN_POINT('Ctrl Pts',(-55.7374561790016,59.9995175300878,-7.17031832941094));
#35197=CARTESIAN_POINT('Ctrl Pts',(-55.738291457224,60.4645797279776,-7.14423966167234));
#35198=CARTESIAN_POINT('Ctrl Pts',(-55.8149019517132,60.9297875761441,-7.11816099393373));
#35199=CARTESIAN_POINT('Ctrl Pts',(-55.9641974254798,61.3713748268308,-7.09208232619513));
#35200=CARTESIAN_POINT('Ctrl Pts',(-56.187306021621,62.0312870739269,-7.0531101135647));
#35201=CARTESIAN_POINT('Ctrl Pts',(-56.5727390884561,62.6384483809869,-7.01413790093427));
#35202=CARTESIAN_POINT('Ctrl Pts',(-57.0811320333225,63.1120990715827,-6.97516568830384));
#35203=CARTESIAN_POINT('Ctrl Pts',(-58.0979179230553,64.0594004527741,-6.89722126304298));
#35204=CARTESIAN_POINT('Ctrl Pts',(-59.6065433249131,64.4726593681082,-6.81927683778212));
#35205=CARTESIAN_POINT('Ctrl Pts',(-60.9556947910596,64.1619004906492,-6.74133241252127));
#35206=CARTESIAN_POINT('Ctrl Pts',(-62.3048462572061,63.8511416131902,-6.66338798726041));
#35207=CARTESIAN_POINT('Ctrl Pts',(-63.4945237876413,62.8163649429381,-6.58544356199955));
#35208=CARTESIAN_POINT('Ctrl Pts',(-63.9892742016634,61.5233054754929,-6.50749913673869));
#35209=CARTESIAN_POINT('Ctrl Pts',(-64.4840246156856,60.2302460080477,-6.42955471147783));
#35210=CARTESIAN_POINT('Ctrl Pts',(-64.2838479132947,58.6789037434093,-6.35161028621697));
#35211=CARTESIAN_POINT('Ctrl Pts',(-63.4866146246838,57.5406364040299,-6.27366586095611));
#35212=CARTESIAN_POINT('Ctrl Pts',(-63.0879979803783,56.9715027343402,-6.23469364832568));
#35213=CARTESIAN_POINT('Ctrl Pts',(-62.5401171895178,56.5056377959653,-6.19572143569525));
#35214=CARTESIAN_POINT('Ctrl Pts',(-61.9174965995694,56.1932194538155,-6.15674922306481));
#35215=CARTESIAN_POINT('Ctrl Pts',(-61.2948760096211,55.8808011116656,-6.11777701043439));
#35216=CARTESIAN_POINT('Ctrl Pts',(-60.5975156205848,55.7218293657408,-6.07880479780396));
#35217=CARTESIAN_POINT('Ctrl Pts',(-59.9025380935532,55.7375113780632,-6.03983258517353));
#35218=CARTESIAN_POINT('Ctrl Pts',(-59.2075605665216,55.7531933903855,-6.0008603725431));
#35219=CARTESIAN_POINT('Ctrl Pts',(-58.5149659014947,55.943529160955,-5.96188815991267));
#35220=CARTESIAN_POINT('Ctrl Pts',(-57.9084055195204,56.2849718118835,-5.92291594728224));
#35221=CARTESIAN_POINT('Ctrl Pts',(-57.3018451375461,56.6264144628121,-5.88394373465181));
#35222=CARTESIAN_POINT('Ctrl Pts',(-56.7813190386245,57.1189639940998,-5.84497152202137));
#35223=CARTESIAN_POINT('Ctrl Pts',(-56.4069717174883,57.7052706177407,-5.80599930939095));
#35224=CARTESIAN_POINT('Ctrl Pts',(-56.0326243963522,58.2915772413817,-5.76702709676052));
#35225=CARTESIAN_POINT('Ctrl Pts',(-55.8044558530015,58.9716409573759,-5.72805488413009));
#35226=CARTESIAN_POINT('Ctrl Pts',(-55.7497674707456,59.6652712843004,-5.68908267149966));
#35227=CARTESIAN_POINT('Ctrl Pts',(-55.7409903494441,59.7765943344006,-5.68282789080342));
#35228=CARTESIAN_POINT('Ctrl Pts',(-55.7366817497711,59.888266834801,-5.67657311010718));
#35229=CARTESIAN_POINT('Ctrl Pts',(-55.7367830248949,59.9999456221449,-5.67031832941094));
#35230=CARTESIAN_POINT('Ctrl Pts',(-55.7373026574226,60.0053877648092,-6.07968167058906));
#35231=CARTESIAN_POINT('Ctrl Pts',(-55.7471879551968,58.9392739868406,-6.13934364288561));
#35232=CARTESIAN_POINT('Ctrl Pts',(-56.1540183693135,57.8645465344337,-6.19900561518217));
#35233=CARTESIAN_POINT('Ctrl Pts',(-56.8759754147187,57.0887747469718,-6.25866758747873));
#35234=CARTESIAN_POINT('Ctrl Pts',(-57.8191645987341,56.0752801577091,-6.33661201273959));
#35235=CARTESIAN_POINT('Ctrl Pts',(-59.300202345866,55.5720340173595,-6.41455643800045));
#35236=CARTESIAN_POINT('Ctrl Pts',(-60.6732079819148,55.7867198306422,-6.49250086326131));
#35237=CARTESIAN_POINT('Ctrl Pts',(-61.3597107999392,55.8940627372836,-6.53147307589174));
#35238=CARTESIAN_POINT('Ctrl Pts',(-62.0192055901928,56.180888632333,-6.57044528852217));
#35239=CARTESIAN_POINT('Ctrl Pts',(-62.5738281627304,56.6023806143966,-6.6094175011526));
#35240=CARTESIAN_POINT('Ctrl Pts',(-63.1284507352679,57.0238725964602,-6.64838971378303));
#35241=CARTESIAN_POINT('Ctrl Pts',(-63.5782010900893,57.580030665538,-6.68736192641346));
#35242=CARTESIAN_POINT('Ctrl Pts',(-63.8700858814464,58.2109380653483,-6.72633413904389));
#35243=CARTESIAN_POINT('Ctrl Pts',(-64.1619706728036,58.8418454651586,-6.76530635167432));
#35244=CARTESIAN_POINT('Ctrl Pts',(-64.2959899006966,59.5475021957015,-6.80427856430475));
#35245=CARTESIAN_POINT('Ctrl Pts',(-64.2564571325936,60.2424376135327,-6.84325077693518));
#35246=CARTESIAN_POINT('Ctrl Pts',(-64.2169243644906,60.9373730313639,-6.88222298956561));
#35247=CARTESIAN_POINT('Ctrl Pts',(-64.0038396003916,61.6215871364834,-6.92119520219604));
#35248=CARTESIAN_POINT('Ctrl Pts',(-63.6422173414806,62.2158270645543,-6.96016741482647));
#35249=CARTESIAN_POINT('Ctrl Pts',(-63.2805950825697,62.8100669926251,-6.9991396274569));
#35250=CARTESIAN_POINT('Ctrl Pts',(-62.7704353288467,63.3143327436474,-7.03811184008733));
#35251=CARTESIAN_POINT('Ctrl Pts',(-62.1717193513747,63.6688083145846,-7.07708405271776));
#35252=CARTESIAN_POINT('Ctrl Pts',(-61.5730033739028,64.0232838855219,-7.11605626534819));
#35253=CARTESIAN_POINT('Ctrl Pts',(-60.8857311726819,64.2279692763742,-7.15502847797862));
#35254=CARTESIAN_POINT('Ctrl Pts',(-60.1906808759037,64.2590561721801,-7.19400069060905));
#35255=CARTESIAN_POINT('Ctrl Pts',(-59.4956305791255,64.2901430679861,-7.23297290323948));
#35256=CARTESIAN_POINT('Ctrl Pts',(-58.7928021867899,64.1476314687458,-7.2719451158699));
#35257=CARTESIAN_POINT('Ctrl Pts',(-58.1648124753609,63.8481564824943,-7.31091732850033));
#35258=CARTESIAN_POINT('Ctrl Pts',(-57.536822763932,63.5486814962429,-7.34988954113076));
#35259=CARTESIAN_POINT('Ctrl Pts',(-56.9836717334097,63.0922431229803,-7.38886175376119));
#35260=CARTESIAN_POINT('Ctrl Pts',(-56.5703777452405,62.5325470504499,-7.42783396639163));
#35261=CARTESIAN_POINT('Ctrl Pts',(-56.1570837570713,61.9728509779196,-7.46680617902206));
#35262=CARTESIAN_POINT('Ctrl Pts',(-55.8836468112551,61.3098972061215,-7.50577839165248));
#35263=CARTESIAN_POINT('Ctrl Pts',(-55.782208591691,60.6215873305249,-7.54475060428291));
#35264=CARTESIAN_POINT('Ctrl Pts',(-55.75190199686,60.4159416813061,-7.55639429305163));
#35265=CARTESIAN_POINT('Ctrl Pts',(-55.7369485091749,60.2080326724282,-7.56803798182034));
#35266=CARTESIAN_POINT('Ctrl Pts',(-55.7371269276513,60.000097806567,-7.57968167058905));
#35267=CARTESIAN_POINT('Origin',(-60.,60.,-6.));
#35268=CARTESIAN_POINT('',(-55.7367869586782,60.0000762880139,-9.07968167058905));
#35269=CARTESIAN_POINT('',(-55.7373303217998,60.0000007547395,-8.67031832941094));
#35270=CARTESIAN_POINT('',(-55.737,60.,-6.));
#35271=CARTESIAN_POINT('',(-63.2233527839579,62.7898325810254,-10.));
#35272=CARTESIAN_POINT('Ctrl Pts',(-55.7367869586782,60.0000762880139,-9.07968167058905));
#35273=CARTESIAN_POINT('Ctrl Pts',(-55.7372968301002,59.3936235369182,-9.11364895864636));
#35274=CARTESIAN_POINT('Ctrl Pts',(-55.8681266030866,58.786957945418,-9.14761624670367));
#35275=CARTESIAN_POINT('Ctrl Pts',(-56.1191760766754,58.2349683861818,-9.18158353476097));
#35276=CARTESIAN_POINT('Ctrl Pts',(-56.4072165422244,57.6016456894732,-9.2205557473914));
#35277=CARTESIAN_POINT('Ctrl Pts',(-56.8535144055287,57.0402986052668,-9.25952796002183));
#35278=CARTESIAN_POINT('Ctrl Pts',(-57.4056092260623,56.6169137142176,-9.29850017265226));
#35279=CARTESIAN_POINT('Ctrl Pts',(-57.9577040465959,56.1935288231683,-9.33747238528269));
#35280=CARTESIAN_POINT('Ctrl Pts',(-58.6155958243587,55.9081061252761,-9.37644459791312));
#35281=CARTESIAN_POINT('Ctrl Pts',(-59.3019542332415,55.794188192632,-9.41541681054355));
#35282=CARTESIAN_POINT('Ctrl Pts',(-59.9883126421243,55.6802702599879,-9.45438902317398));
#35283=CARTESIAN_POINT('Ctrl Pts',(-60.7031376821272,55.7378570925918,-9.49336123580441));
#35284=CARTESIAN_POINT('Ctrl Pts',(-61.3624026680008,55.9601950787861,-9.53233344843484));
#35285=CARTESIAN_POINT('Ctrl Pts',(-62.0216676538744,56.1825330649805,-9.57130566106527));
#35286=CARTESIAN_POINT('Ctrl Pts',(-62.6253725856187,56.5696222047652,-9.6102778736957));
#35287=CARTESIAN_POINT('Ctrl Pts',(-63.1025601776872,57.0759275956669,-9.64925008632613));
#35288=CARTESIAN_POINT('Ctrl Pts',(-63.5797477697557,57.5822329865685,-9.68822229895656));
#35289=CARTESIAN_POINT('Ctrl Pts',(-63.9304180221485,58.2077546285871,-9.72719451158699));
#35290=CARTESIAN_POINT('Ctrl Pts',(-64.113334662525,58.8790350253607,-9.76616672421742));
#35291=CARTESIAN_POINT('Ctrl Pts',(-64.2962513029015,59.5503154221343,-9.80513893684785));
#35292=CARTESIAN_POINT('Ctrl Pts',(-64.3114143312618,60.267354573663,-9.84411114947828));
#35293=CARTESIAN_POINT('Ctrl Pts',(-64.1570472486001,60.9456836607563,-9.88308336210871));
#35294=CARTESIAN_POINT('Ctrl Pts',(-64.0026801659383,61.6240127478497,-9.92205557473914));
#35295=CARTESIAN_POINT('Ctrl Pts',(-63.6787829722545,62.2636317705077,-9.96102778736957));
#35296=CARTESIAN_POINT('Ctrl Pts',(-63.2233527839579,62.7898325810254,-10.));
#35297=CARTESIAN_POINT('',(-56.7764331619493,62.7899186857328,-10.));
#35298=CARTESIAN_POINT('Origin',(-60.,60.,-10.));
#35299=CARTESIAN_POINT('Ctrl Pts',(-56.7764331619493,62.7899186857328,-10.));
#35300=CARTESIAN_POINT('Ctrl Pts',(-57.1737624197776,63.2482129439588,-9.96602721186203));
#35301=CARTESIAN_POINT('Ctrl Pts',(-57.6698071152885,63.6213495269443,-9.93205442372406));
#35302=CARTESIAN_POINT('Ctrl Pts',(-58.2209772071418,63.8744287315555,-9.89808163558608));
#35303=CARTESIAN_POINT('Ctrl Pts',(-58.8532573110885,64.1647509898991,-9.85910942295565));
#35304=CARTESIAN_POINT('Ctrl Pts',(-59.5580810762401,64.2970807010714,-9.82013721032522));
#35305=CARTESIAN_POINT('Ctrl Pts',(-60.2526054582228,64.2558578621421,-9.78116499769479));
#35306=CARTESIAN_POINT('Ctrl Pts',(-60.9471298402055,64.2146350232128,-9.74219278506436));
#35307=CARTESIAN_POINT('Ctrl Pts',(-61.6313548390192,63.9998596341819,-9.70322057243393));
#35308=CARTESIAN_POINT('Ctrl Pts',(-62.2248512269878,63.6367797954782,-9.6642483598035));
#35309=CARTESIAN_POINT('Ctrl Pts',(-62.8183476149565,63.2736999567746,-9.62527614717307));
#35310=CARTESIAN_POINT('Ctrl Pts',(-63.32111539208,62.7623156683981,-9.58630393454264));
#35311=CARTESIAN_POINT('Ctrl Pts',(-63.6740580837607,62.1627361795151,-9.54733172191221));
#35312=CARTESIAN_POINT('Ctrl Pts',(-64.0270007754414,61.563156690632,-9.50835950928178));
#35313=CARTESIAN_POINT('Ctrl Pts',(-64.2301183816792,60.8753820012424,-9.46938729665135));
#35314=CARTESIAN_POINT('Ctrl Pts',(-64.2595350443961,60.1802567460833,-9.43041508402092));
#35315=CARTESIAN_POINT('Ctrl Pts',(-64.288951707113,59.4851314909241,-9.39144287139049));
#35316=CARTESIAN_POINT('Ctrl Pts',(-64.1446674263089,58.7826556699956,-9.35247065876007));
#35317=CARTESIAN_POINT('Ctrl Pts',(-63.843642256701,58.1554011805957,-9.31349844612963));
#35318=CARTESIAN_POINT('Ctrl Pts',(-63.5426170870931,57.5281466911958,-9.27452623349921));
#35319=CARTESIAN_POINT('Ctrl Pts',(-63.0848510286812,56.9761135333246,-9.23555402086878));
#35320=CARTESIAN_POINT('Ctrl Pts',(-62.5241518355292,56.5641902660268,-9.19658180823834));
#35321=CARTESIAN_POINT('Ctrl Pts',(-61.9634526423771,56.1522669987289,-9.15760959560791));
#35322=CARTESIAN_POINT('Ctrl Pts',(-61.2998203144848,55.8804536220044,-9.11863738297748));
#35323=CARTESIAN_POINT('Ctrl Pts',(-60.611261215134,55.7807002318295,-9.07966517034705));
#35324=CARTESIAN_POINT('Ctrl Pts',(-59.9227021157832,55.6809468416546,-9.04069295771662));
#35325=CARTESIAN_POINT('Ctrl Pts',(-59.2092162449739,55.7532534380294,-9.0017207450862));
#35326=CARTESIAN_POINT('Ctrl Pts',(-58.554669879246,55.9891208250959,-8.96274853245577));
#35327=CARTESIAN_POINT('Ctrl Pts',(-57.900123513518,56.2249882121624,-8.92377631982534));
#35328=CARTESIAN_POINT('Ctrl Pts',(-57.3045166528713,56.6244163899207,-8.88480410719491));
#35329=CARTESIAN_POINT('Ctrl Pts',(-56.8378596282339,57.1404547329625,-8.84583189456448));
#35330=CARTESIAN_POINT('Ctrl Pts',(-56.3712026035963,57.6564930760043,-8.80685968193405));
#35331=CARTESIAN_POINT('Ctrl Pts',(-56.033495414968,58.2891415843297,-8.76788746930362));
#35332=CARTESIAN_POINT('Ctrl Pts',(-55.8644336009782,58.9640360264496,-8.72891525667319));
#35333=CARTESIAN_POINT('Ctrl Pts',(-55.7797022659359,59.3022833558961,-8.70938294758577));
#35334=CARTESIAN_POINT('Ctrl Pts',(-55.7373324459271,59.6511423120379,-8.68985063849836));
#35335=CARTESIAN_POINT('Ctrl Pts',(-55.7373303217998,60.0000007547395,-8.67031832941094));
#35336=CARTESIAN_POINT('Origin',(-60.,60.,-13.3123464956316));
#35337=CARTESIAN_POINT('',(-54.9005857509307,60.0000080970678,-3.68765350436841));
#35338=CARTESIAN_POINT('',(-54.9008894739474,59.9998849445721,-3.56234649563159));
#35339=CARTESIAN_POINT('',(-54.901,59.9999999999999,-13.3123464956316));
#35340=CARTESIAN_POINT('',(-63.6032183801568,63.607855083689,-3.));
#35341=CARTESIAN_POINT('Ctrl Pts',(-54.9008894739474,59.9998849445721,-3.56234649563159));
#35342=CARTESIAN_POINT('Ctrl Pts',(-54.9015382889875,60.6739141994399,-3.53078651427611));
#35343=CARTESIAN_POINT('Ctrl Pts',(-55.2021867355797,62.1808417896872,-3.46025432029021));
#35344=CARTESIAN_POINT('Ctrl Pts',(-56.644415546233,64.1119168166584,-3.35074991367387));
#35345=CARTESIAN_POINT('Ctrl Pts',(-58.9729552216983,65.2070699739396,-3.23383327578258));
#35346=CARTESIAN_POINT('Ctrl Pts',(-61.5432550625777,65.077974056636,-3.11691663789129));
#35347=CARTESIAN_POINT('Ctrl Pts',(-63.0142489447552,64.1960675938266,-3.03897221263043));
#35348=CARTESIAN_POINT('Ctrl Pts',(-63.6032183801568,63.6078550836889,-3.));
#35349=CARTESIAN_POINT('',(-64.9263786426945,61.3165318579407,-3.));
#35350=CARTESIAN_POINT('Origin',(-60.,60.,-3.));
#35351=CARTESIAN_POINT('Ctrl Pts',(-54.9005857509307,60.0000080970678,-3.68765350436841));
#35352=CARTESIAN_POINT('Ctrl Pts',(-54.9005849635668,60.008207439555,-3.68726952086906));
#35353=CARTESIAN_POINT('Ctrl Pts',(-54.9025709592986,60.8485945510885,-3.64791332473928));
#35354=CARTESIAN_POINT('Ctrl Pts',(-55.3285862201775,62.5191327628181,-3.56958491597908));
#35355=CARTESIAN_POINT('Ctrl Pts',(-57.0626757179785,64.4204363923688,-3.45266827808779));
#35356=CARTESIAN_POINT('Ctrl Pts',(-59.487294255791,65.282543142849,-3.3357516401965));
#35357=CARTESIAN_POINT('Ctrl Pts',(-62.0324515210899,64.9027851981381,-3.21883500230521));
#35358=CARTESIAN_POINT('Ctrl Pts',(-64.0113858210523,63.4359554740898,-3.10691778890637));
#35359=CARTESIAN_POINT('Ctrl Pts',(-64.7384685956641,62.0172737022055,-3.03397278813797));
#35360=CARTESIAN_POINT('Ctrl Pts',(-64.9263786426945,61.3165318579407,-3.));
#35361=CARTESIAN_POINT('Origin',(-60.,60.,-13.3123464956316));
#35362=CARTESIAN_POINT('',(-54.9007404747687,59.9999349583197,-5.18765350436841));
#35363=CARTESIAN_POINT('',(-54.9012719746715,59.9999119425253,-5.06234649563159));
#35364=CARTESIAN_POINT('',(-54.901,59.9999999999999,-13.3123464956316));
#35365=CARTESIAN_POINT('Ctrl Pts',(-54.9012719746715,59.9999119425253,-5.06234649563159));
#35366=CARTESIAN_POINT('Ctrl Pts',(-54.9016210582163,60.5322706427621,-5.0374252784717));
#35367=CARTESIAN_POINT('Ctrl Pts',(-55.1145360435078,61.8974113776361,-4.97353184868138));
#35368=CARTESIAN_POINT('Ctrl Pts',(-56.3134109693639,63.8180111698412,-4.87066620626063));
#35369=CARTESIAN_POINT('Ctrl Pts',(-58.5427258829576,65.1033793524814,-4.75374956836935));
#35370=CARTESIAN_POINT('Ctrl Pts',(-61.1146285576988,65.189001855627,-4.63683293047805));
#35371=CARTESIAN_POINT('Ctrl Pts',(-63.4244950049221,64.0547464033043,-4.51991629258676));
#35372=CARTESIAN_POINT('Ctrl Pts',(-64.9293002545277,61.9672654771257,-4.40299965469547));
#35373=CARTESIAN_POINT('Ctrl Pts',(-65.2752818739828,59.417301951109,-4.28608301680418));
#35374=CARTESIAN_POINT('Ctrl Pts',(-64.3811027318255,57.0043244761643,-4.1691663789129));
#35375=CARTESIAN_POINT('Ctrl Pts',(-62.4569756156385,55.2955969137595,-4.0522497410216));
#35376=CARTESIAN_POINT('Ctrl Pts',(-59.9552391151028,54.6928228512559,-3.93533310313032));
#35377=CARTESIAN_POINT('Ctrl Pts',(-57.4640288733897,55.3377064936621,-3.81841646523903));
#35378=CARTESIAN_POINT('Ctrl Pts',(-55.5689898394584,57.0786455663088,-3.70149982734774));
#35379=CARTESIAN_POINT('Ctrl Pts',(-54.9459956983136,58.8510320242688,-3.61614317081192));
#35380=CARTESIAN_POINT('Ctrl Pts',(-54.9007370921359,59.841581279342,-3.56975872690654));
#35381=CARTESIAN_POINT('Ctrl Pts',(-54.9008894739474,59.9998849445721,-3.56234649563159));
#35382=CARTESIAN_POINT('Ctrl Pts',(-54.9007404747687,59.9999349583197,-5.18765350436841));
#35383=CARTESIAN_POINT('Ctrl Pts',(-54.9013741103876,60.6986619001248,-5.15493607243422));
#35384=CARTESIAN_POINT('Ctrl Pts',(-55.2189956710647,62.2301462927378,-5.0832464278696));
#35385=CARTESIAN_POINT('Ctrl Pts',(-56.7044890264666,64.1603278398107,-4.97258457067455));
#35386=CARTESIAN_POINT('Ctrl Pts',(-59.0489177119773,65.2214359342736,-4.85566793278326));
#35387=CARTESIAN_POINT('Ctrl Pts',(-61.6168265705004,65.0550993586167,-4.73875129489197));
#35388=CARTESIAN_POINT('Ctrl Pts',(-63.8046877780167,63.7003384396424,-4.62183465700068));
#35389=CARTESIAN_POINT('Ctrl Pts',(-65.0980856806054,61.4756811768837,-4.50491801910939));
#35390=CARTESIAN_POINT('Ctrl Pts',(-65.1929908975039,58.9041019334819,-4.3880013812181));
#35391=CARTESIAN_POINT('Ctrl Pts',(-64.067076438205,56.5901588181647,-4.27108474332681));
#35392=CARTESIAN_POINT('Ctrl Pts',(-61.9850396737251,55.0778303984365,-4.15416810543552));
#35393=CARTESIAN_POINT('Ctrl Pts',(-59.4363409530604,54.7226501051879,-4.03725146754423));
#35394=CARTESIAN_POINT('Ctrl Pts',(-57.0201528028271,55.6081161060463,-3.92033482965294));
#35395=CARTESIAN_POINT('Ctrl Pts',(-55.3101280050136,57.5197664213586,-3.803802175261));
#35396=CARTESIAN_POINT('Ctrl Pts',(-54.9006648766645,59.1760192872482,-3.72624173349949));
#35397=CARTESIAN_POINT('Ctrl Pts',(-54.9005857509307,60.0000080970678,-3.68765350436841));
#35398=CARTESIAN_POINT('Origin',(-60.,60.,-13.3123464956316));
#35399=CARTESIAN_POINT('',(-54.901545638454,59.9994229148293,-6.68765350436841));
#35400=CARTESIAN_POINT('',(-54.9013620103677,60.006444337969,-6.56234649563159));
#35401=CARTESIAN_POINT('',(-54.901,59.9999999999999,-13.3123464956316));
#35402=CARTESIAN_POINT('Ctrl Pts',(-54.9013620103677,60.0064443379691,-6.56234649563159));
#35403=CARTESIAN_POINT('Ctrl Pts',(-54.8977387771102,60.3972043317359,-6.54406404266729));
#35404=CARTESIAN_POINT('Ctrl Pts',(-55.1133266770003,62.4488173731316,-6.44783716444213));
#35405=CARTESIAN_POINT('Ctrl Pts',(-57.261136178523,64.881658846174,-6.31263807358654));
#35406=CARTESIAN_POINT('Ctrl Pts',(-60.6812390619036,65.2585277879725,-6.15674922306482));
#35407=CARTESIAN_POINT('Ctrl Pts',(-63.0733675865873,64.3285109623237,-6.03983258517352));
#35408=CARTESIAN_POINT('Ctrl Pts',(-64.7488466585635,62.3700232907153,-5.92291594728224));
#35409=CARTESIAN_POINT('Ctrl Pts',(-65.3052032495076,59.8594450499176,-5.80599930939095));
#35410=CARTESIAN_POINT('Ctrl Pts',(-64.6156238392598,57.3795659933714,-5.68908267149965));
#35411=CARTESIAN_POINT('Ctrl Pts',(-62.8403792200309,55.5168088844888,-5.57216603360837));
#35412=CARTESIAN_POINT('Ctrl Pts',(-60.3976628561038,54.7074974068321,-5.45524939571708));
#35413=CARTESIAN_POINT('Ctrl Pts',(-57.8613353264688,55.1426276840725,-5.33833275782579));
#35414=CARTESIAN_POINT('Ctrl Pts',(-55.8278420769378,56.7195645370492,-5.2214161199345));
#35415=CARTESIAN_POINT('Ctrl Pts',(-54.9995353574893,58.5672219002548,-5.1294206992031));
#35416=CARTESIAN_POINT('Ctrl Pts',(-54.9010751555806,59.6997592799271,-5.07639749110213));
#35417=CARTESIAN_POINT('Ctrl Pts',(-54.9012719746715,59.9999119425253,-5.06234649563159));
#35418=CARTESIAN_POINT('Ctrl Pts',(-54.901545638454,59.9994229148293,-6.68765350436841));
#35419=CARTESIAN_POINT('Ctrl Pts',(-54.9025447197713,60.5556866134078,-6.66157483662981));
#35420=CARTESIAN_POINT('Ctrl Pts',(-55.1311181375491,61.9436707080335,-6.59652395626078));
#35421=CARTESIAN_POINT('Ctrl Pts',(-56.822670191795,64.6083226141335,-6.45352865063088));
#35422=CARTESIAN_POINT('Ctrl Pts',(-61.3338600370175,65.8440763141619,-6.25866758747874));
#35423=CARTESIAN_POINT('Ctrl Pts',(-65.6028014358132,62.1309684734756,-6.02483431169615));
#35424=CARTESIAN_POINT('Ctrl Pts',(-65.0042200345167,57.4920438855145,-5.82997324854401));
#35425=CARTESIAN_POINT('Ctrl Pts',(-62.3829259668669,55.2631484402659,-5.67408439802228));
#35426=CARTESIAN_POINT('Ctrl Pts',(-59.8805750705293,54.692707249224,-5.557167760131));
#35427=CARTESIAN_POINT('Ctrl Pts',(-57.3953251078463,55.3756925371435,-5.44025112223971));
#35428=CARTESIAN_POINT('Ctrl Pts',(-55.5275118929263,57.1431169284426,-5.32333448434842));
#35429=CARTESIAN_POINT('Ctrl Pts',(-54.9378835090541,58.9005233785311,-5.23913527839132));
#35430=CARTESIAN_POINT('Ctrl Pts',(-54.9006193389826,59.8663552875089,-5.19390828506465));
#35431=CARTESIAN_POINT('Ctrl Pts',(-54.9007404747687,59.9999349583197,-5.18765350436841));
#35432=CARTESIAN_POINT('Origin',(-60.,60.,-13.3123464956316));
#35433=CARTESIAN_POINT('',(-54.9013950998961,60.0000009027484,-8.18765350436842));
#35434=CARTESIAN_POINT('',(-54.9011518189288,60.0001169870244,-8.06234649563159));
#35435=CARTESIAN_POINT('',(-54.901,59.9999999999999,-13.3123464956316));
#35436=CARTESIAN_POINT('Ctrl Pts',(-54.9011518189288,60.0001169870244,-8.06234649563159));
#35437=CARTESIAN_POINT('Ctrl Pts',(-54.9009384115137,60.2488291336409,-8.05070280686288));
#35438=CARTESIAN_POINT('Ctrl Pts',(-54.978689873463,61.3298631862382,-8.00008690546373));
#35439=CARTESIAN_POINT('Ctrl Pts',(-55.7305242936952,63.1527019513981,-7.91049879143416));
#35440=CARTESIAN_POINT('Ctrl Pts',(-57.7154061407277,64.7905480212547,-7.79358215354287));
#35441=CARTESIAN_POINT('Ctrl Pts',(-60.237377972198,65.3019249702528,-7.67666551565158));
#35442=CARTESIAN_POINT('Ctrl Pts',(-62.7035292417443,64.5674486803472,-7.55974887776029));
#35443=CARTESIAN_POINT('Ctrl Pts',(-64.5341447127037,62.7579827658769,-7.442832239869));
#35444=CARTESIAN_POINT('Ctrl Pts',(-65.2987606255403,60.3028049178794,-7.32591560197772));
#35445=CARTESIAN_POINT('Ctrl Pts',(-64.8178570062396,57.770684109267,-7.20899896408642));
#35446=CARTESIAN_POINT('Ctrl Pts',(-63.2040096739143,55.7750120514012,-7.09208232619513));
#35447=CARTESIAN_POINT('Ctrl Pts',(-60.0487068960553,54.4027153224711,-6.93619347567341));
#35448=CARTESIAN_POINT('Ctrl Pts',(-56.0355250219872,55.7663661089261,-6.75961486548557));
#35449=CARTESIAN_POINT('Ctrl Pts',(-54.9131858746302,58.7312592209477,-6.62200846792815));
#35450=CARTESIAN_POINT('Ctrl Pts',(-54.9013620103677,60.0064443379691,-6.56234649563159));
#35451=CARTESIAN_POINT('Ctrl Pts',(-54.9013950998961,60.0000009027484,-8.18765350436842));
#35452=CARTESIAN_POINT('Ctrl Pts',(-54.9013925712344,60.4152985155146,-8.1682136008254));
#35453=CARTESIAN_POINT('Ctrl Pts',(-55.0522172876686,61.6631635996099,-8.10980148465195));
#35454=CARTESIAN_POINT('Ctrl Pts',(-56.059376560482,63.5552235595967,-8.01241715584808));
#35455=CARTESIAN_POINT('Ctrl Pts',(-58.1949364984747,64.9909811437472,-7.89550051795679));
#35456=CARTESIAN_POINT('Ctrl Pts',(-60.7548501786328,65.2534097268154,-7.7785838800655));
#35457=CARTESIAN_POINT('Ctrl Pts',(-63.1372998197884,64.2808297669235,-7.66166724217421));
#35458=CARTESIAN_POINT('Ctrl Pts',(-64.7822203790914,62.3018527171852,-7.54475060428292));
#35459=CARTESIAN_POINT('Ctrl Pts',(-65.3028606950879,59.7817818006449,-7.42783396639163));
#35460=CARTESIAN_POINT('Ctrl Pts',(-64.5769288017872,57.3129117888108,-7.31091732850034));
#35461=CARTESIAN_POINT('Ctrl Pts',(-62.7748569607921,55.4759618947992,-7.19400069060905));
#35462=CARTESIAN_POINT('Ctrl Pts',(-60.3207807277454,54.7020982939809,-7.07708405271776));
#35463=CARTESIAN_POINT('Ctrl Pts',(-57.7905713642451,55.1747170180384,-6.96016741482648));
#35464=CARTESIAN_POINT('Ctrl Pts',(-55.7813283808542,56.7795403162521,-6.84325077693518));
#35465=CARTESIAN_POINT('Ctrl Pts',(-54.9881855005153,58.6182641032336,-6.75241280678249));
#35466=CARTESIAN_POINT('Ctrl Pts',(-54.9010516830133,59.7244007763825,-6.70054704926024));
#35467=CARTESIAN_POINT('Ctrl Pts',(-54.901545638454,59.9994229148293,-6.68765350436841));
#35468=CARTESIAN_POINT('Origin',(-60.,60.,-13.3123464956316));
#35469=CARTESIAN_POINT('',(-54.9012106446239,60.0001195814448,-9.68765350436841));
#35470=CARTESIAN_POINT('',(-54.9007451799907,60.0000912485532,-9.56234649563159));
#35471=CARTESIAN_POINT('',(-54.901,59.9999999999999,-13.3123464956316));
#35472=CARTESIAN_POINT('',(-58.677115034431,55.0755938055567,-10.));
#35473=CARTESIAN_POINT('Ctrl Pts',(-58.677115034431,55.0755938055567,-10.));
#35474=CARTESIAN_POINT('Ctrl Pts',(-57.8732233401272,55.2915500435982,-9.96102778736957));
#35475=CARTESIAN_POINT('Ctrl Pts',(-56.3739727673179,56.1245137043432,-9.88308336210872));
#35476=CARTESIAN_POINT('Ctrl Pts',(-55.1299740822569,58.0492615027565,-9.77896786356484));
#35477=CARTESIAN_POINT('Ctrl Pts',(-54.9016327694172,59.4410930379684,-9.71382457765142));
#35478=CARTESIAN_POINT('Ctrl Pts',(-54.9012106446239,60.0001195814448,-9.68765350436841));
#35479=CARTESIAN_POINT('',(-61.3230392943658,55.0753649202911,-10.));
#35480=CARTESIAN_POINT('Origin',(-60.,60.,-10.));
#35481=CARTESIAN_POINT('Ctrl Pts',(-61.3230392943658,55.0753649202911,-10.));
#35482=CARTESIAN_POINT('Ctrl Pts',(-60.6222240320617,54.8877288802907,-9.96602721186203));
#35483=CARTESIAN_POINT('Ctrl Pts',(-59.0300681471914,54.8080601177165,-9.89308221109362));
#35484=CARTESIAN_POINT('Ctrl Pts',(-56.77028917635,55.7884526872829,-9.78116499769479));
#35485=CARTESIAN_POINT('Ctrl Pts',(-55.2373851384779,57.7165175129953,-9.66925328437663));
#35486=CARTESIAN_POINT('Ctrl Pts',(-54.9013550402723,59.2747094568956,-9.5963137836889));
#35487=CARTESIAN_POINT('Ctrl Pts',(-54.9007451799907,60.0000912485532,-9.56234649563159));
#35488=CARTESIAN_POINT('Origin',(-60.,60.,-3.));
#35489=CARTESIAN_POINT('Ctrl Pts',(-59.1956105045055,55.8135783132204,-3.));
#35490=CARTESIAN_POINT('Ctrl Pts',(-59.3195769365686,55.7770540578209,-3.));
#35491=CARTESIAN_POINT('Ctrl Pts',(-59.445059760185,55.7463481720298,-3.));
#35492=CARTESIAN_POINT('Ctrl Pts',(-59.5716383186483,55.7213771363331,-3.));
#35493=CARTESIAN_POINT('Ctrl Pts',(-59.7000945008852,55.6960356886894,-3.));
#35494=CARTESIAN_POINT('Ctrl Pts',(-59.8296798459766,55.6766002514243,-3.));
#35495=CARTESIAN_POINT('Ctrl Pts',(-59.959981179512,55.6630301115702,-3.));
#35496=CARTESIAN_POINT('Ctrl Pts',(-60.0181559866187,55.6569715375939,-3.));
#35497=CARTESIAN_POINT('Ctrl Pts',(-60.0764737978558,55.6520827276688,-3.));
#35498=CARTESIAN_POINT('Ctrl Pts',(-60.1348989470971,55.6483631838136,-3.));
#35499=CARTESIAN_POINT('Ctrl Pts',(-60.1584275152761,55.646865275082,-3.));
#35500=CARTESIAN_POINT('Ctrl Pts',(-60.1819734969942,55.6455570175179,-3.));
#35501=CARTESIAN_POINT('Ctrl Pts',(-60.2055345827709,55.6444384689613,-3.));
#35502=CARTESIAN_POINT('Ctrl Pts',(-60.2289638731321,55.6433261773138,-3.));
#35503=CARTESIAN_POINT('Ctrl Pts',(-60.2523986226803,55.6424019433942,-3.));
#35504=CARTESIAN_POINT('Ctrl Pts',(-60.2758336778232,55.6416654642661,-3.));
#35505=CARTESIAN_POINT('Ctrl Pts',(-60.4095527621665,55.6374631564819,-3.));
#35506=CARTESIAN_POINT('Ctrl Pts',(-60.5433094949031,55.6393683817081,-3.));
#35507=CARTESIAN_POINT('Ctrl Pts',(-60.6766724777373,55.6473288482565,-3.));
#35508=CARTESIAN_POINT('Ctrl Pts',(-60.7846049163009,55.6537713598771,-3.));
#35509=CARTESIAN_POINT('Ctrl Pts',(-60.8922801012417,55.6641808613591,-3.));
#35510=CARTESIAN_POINT('Ctrl Pts',(-60.9994758570612,55.6785535027164,-3.));
#35511=CARTESIAN_POINT('Ctrl Pts',(-61.053073734971,55.685739823395,-3.));
#35512=CARTESIAN_POINT('Ctrl Pts',(-61.1065518155819,55.6939172672668,-3.));
#35513=CARTESIAN_POINT('Ctrl Pts',(-61.159882506232,55.7030874102868,-3.));
#35514=CARTESIAN_POINT('Ctrl Pts',(-61.1872713887428,55.7077968930766,-3.));
#35515=CARTESIAN_POINT('Ctrl Pts',(-61.2146213974502,55.7127682237387,-3.));
#35516=CARTESIAN_POINT('Ctrl Pts',(-61.2419287911558,55.7180017588153,-3.));
#35517=CARTESIAN_POINT('Ctrl Pts',(-61.2615202355303,55.7217565115552,-3.));
#35518=CARTESIAN_POINT('Ctrl Pts',(-61.2810875141073,55.7256458533217,-3.));
#35519=CARTESIAN_POINT('Ctrl Pts',(-61.3006183099631,55.7296674434209,-3.));
#35520=CARTESIAN_POINT('Ctrl Pts',(-61.3068720706772,55.7309551565462,-3.));
#35521=CARTESIAN_POINT('Ctrl Pts',(-61.3131224068267,55.7322564887182,-3.));
#35522=CARTESIAN_POINT('Ctrl Pts',(-61.3193692733847,55.7335714316187,-3.));
#35523=CARTESIAN_POINT('Ctrl Pts',(-61.4494244547665,55.760947578659,-3.));
#35524=CARTESIAN_POINT('Ctrl Pts',(-61.577974912008,55.7942188050333,-3.));
#35525=CARTESIAN_POINT('Ctrl Pts',(-61.704692114971,55.8330909005726,-3.));
#35526=CARTESIAN_POINT('Ctrl Pts',(-61.8336752302035,55.8726580931955,-3.));
#35527=CARTESIAN_POINT('Ctrl Pts',(-61.9607596091681,55.91802834131,-3.));
#35528=CARTESIAN_POINT('Ctrl Pts',(-62.0856036012641,55.9689451560091,-3.));
#35529=CARTESIAN_POINT('Ctrl Pts',(-62.2120507894683,56.0205158238717,-3.));
#35530=CARTESIAN_POINT('Ctrl Pts',(-62.3362004369027,56.0777765786684,-3.));
#35531=CARTESIAN_POINT('Ctrl Pts',(-62.4576916079016,56.1405137039557,-3.));
#35532=CARTESIAN_POINT('Ctrl Pts',(-62.5340614666828,56.1799505235957,-3.));
#35533=CARTESIAN_POINT('Ctrl Pts',(-62.6093806902554,56.2215523381483,-3.));
#35534=CARTESIAN_POINT('Ctrl Pts',(-62.6835563590128,56.2652760862483,-3.));
#35535=CARTESIAN_POINT('Ctrl Pts',(-62.7445595014197,56.3012351288372,-3.));
#35536=CARTESIAN_POINT('Ctrl Pts',(-62.8047891530527,56.3386295207014,-3.));
#35537=CARTESIAN_POINT('Ctrl Pts',(-62.8641916904358,56.3774390056312,-3.));
#35538=CARTESIAN_POINT('Ctrl Pts',(-62.8791980541292,56.3872431195843,-3.));
#35539=CARTESIAN_POINT('Ctrl Pts',(-62.8941498090572,56.3971364251801,-3.));
#35540=CARTESIAN_POINT('Ctrl Pts',(-62.9090367420972,56.4071121284225,-3.));
#35541=CARTESIAN_POINT('Ctrl Pts',(-63.0253590231817,56.485059449973,-3.));
#35542=CARTESIAN_POINT('Ctrl Pts',(-63.1378862566305,56.5681385841153,-3.));
#35543=CARTESIAN_POINT('Ctrl Pts',(-63.2462619950014,56.656078356157,-3.));
#35544=CARTESIAN_POINT('Ctrl Pts',(-63.2693908817498,56.6748459240537,-3.));
#35545=CARTESIAN_POINT('Ctrl Pts',(-63.2923306567195,56.6938350587944,-3.));
#35546=CARTESIAN_POINT('Ctrl Pts',(-63.3150777939445,56.7130434235261,-3.));
#35547=CARTESIAN_POINT('Ctrl Pts',(-63.4206898136458,56.8022253796735,-3.));
#35548=CARTESIAN_POINT('Ctrl Pts',(-63.5221511112837,56.8961292683318,-3.));
#35549=CARTESIAN_POINT('Ctrl Pts',(-63.6192855225016,56.9943655518854,-3.));
#35550=CARTESIAN_POINT('Ctrl Pts',(-63.7175323011257,57.0937268213073,-3.));
#35551=CARTESIAN_POINT('Ctrl Pts',(-63.8113530858956,57.1975207545623,-3.));
#35552=CARTESIAN_POINT('Ctrl Pts',(-63.9005375437739,57.305389517552,-3.));
#35553=CARTESIAN_POINT('Ctrl Pts',(-63.9806728177378,57.4023132762423,-3.));
#35554=CARTESIAN_POINT('Ctrl Pts',(-64.0570647960701,57.5025277837558,-3.));
#35555=CARTESIAN_POINT('Ctrl Pts',(-64.1295362219416,57.6057990786673,-3.));
#35556=CARTESIAN_POINT('Ctrl Pts',(-64.1412822857501,57.6225371406694,-3.));
#35557=CARTESIAN_POINT('Ctrl Pts',(-64.1529253027095,57.6393555477934,-3.));
#35558=CARTESIAN_POINT('Ctrl Pts',(-64.1644644511097,57.6562533540464,-3.));
#35559=CARTESIAN_POINT('Ctrl Pts',(-64.1746328838408,57.6711438988445,-3.));
#35560=CARTESIAN_POINT('Ctrl Pts',(-64.1847153144395,57.6860882798462,-3.));
#35561=CARTESIAN_POINT('Ctrl Pts',(-64.1947109245644,57.7010848983457,-3.));
#35562=CARTESIAN_POINT('Ctrl Pts',(-64.2739894697328,57.8200281226444,-3.));
#35563=CARTESIAN_POINT('Ctrl Pts',(-64.3478189157374,57.9422686542718,-3.));
#35564=CARTESIAN_POINT('Ctrl Pts',(-64.4160215894327,58.0673941364165,-3.));
#35565=CARTESIAN_POINT('Ctrl Pts',(-64.4849569820396,58.193863873883,-3.));
#35566=CARTESIAN_POINT('Ctrl Pts',(-64.5481446301058,58.3232814243193,-3.));
#35567=CARTESIAN_POINT('Ctrl Pts',(-64.6053684730552,58.4552626417141,-3.));
#35568=CARTESIAN_POINT('Ctrl Pts',(-64.6262261154663,58.5033687613929,-3.));
#35569=CARTESIAN_POINT('Ctrl Pts',(-64.6462910856029,58.5518158315677,-3.));
#35570=CARTESIAN_POINT('Ctrl Pts',(-64.665551625707,58.6005863831579,-3.));
#35571=CARTESIAN_POINT('Ctrl Pts',(-64.7181182841506,58.7336929790112,-3.));
#35572=CARTESIAN_POINT('Ctrl Pts',(-64.7646963550687,58.8692073663929,-3.));
#35573=CARTESIAN_POINT('Ctrl Pts',(-64.8052734936232,59.0067151216772,-3.));
#35574=CARTESIAN_POINT('Ctrl Pts',(-64.8290066390675,59.0871419746329,-3.));
#35575=CARTESIAN_POINT('Ctrl Pts',(-64.8506860242825,59.1682512449237,-3.));
#35576=CARTESIAN_POINT('Ctrl Pts',(-64.8703015754152,59.2499631360153,-3.));
#35577=CARTESIAN_POINT('Ctrl Pts',(-64.8777895471377,59.2811555468604,-3.));
#35578=CARTESIAN_POINT('Ctrl Pts',(-64.8849767115593,59.3124357915603,-3.));
#35579=CARTESIAN_POINT('Ctrl Pts',(-64.8918622845764,59.3437994898947,-3.));
#35580=CARTESIAN_POINT('Ctrl Pts',(-64.8973648848784,59.3688637649373,-3.));
#35581=CARTESIAN_POINT('Ctrl Pts',(-64.9026757353232,59.3939859734578,-3.));
#35582=CARTESIAN_POINT('Ctrl Pts',(-64.9077887067164,59.4191347884762,-3.));
#35583=CARTESIAN_POINT('Ctrl Pts',(-64.9369315292006,59.5624775524785,-3.));
#35584=CARTESIAN_POINT('Ctrl Pts',(-64.9596873533747,59.7068444160501,-3.));
#35585=CARTESIAN_POINT('Ctrl Pts',(-64.9761061056319,59.8517783133678,-3.));
#35586=CARTESIAN_POINT('Ctrl Pts',(-64.9926869506057,59.9981430580958,-3.));
#35587=CARTESIAN_POINT('Ctrl Pts',(-65.0028052187048,60.1450868049904,-3.));
#35588=CARTESIAN_POINT('Ctrl Pts',(-65.0064655586371,60.2921650192025,-3.));
#35589=CARTESIAN_POINT('Ctrl Pts',(-65.0101294420625,60.4393856165403,-3.));
#35590=CARTESIAN_POINT('Ctrl Pts',(-65.0073230692564,60.586741719856,-3.));
#35591=CARTESIAN_POINT('Ctrl Pts',(-64.9980014221604,60.7338023037548,-3.));
#35592=CARTESIAN_POINT('Ctrl Pts',(-64.9923757401215,60.8225544391829,-3.));
#35593=CARTESIAN_POINT('Ctrl Pts',(-64.9843760879495,60.9111991744113,-3.));
#35594=CARTESIAN_POINT('Ctrl Pts',(-64.9739833939208,60.9996425419769,-3.));
#35595=CARTESIAN_POINT('Ctrl Pts',(-64.9615316541797,61.1056086939404,-3.));
#35596=CARTESIAN_POINT('Ctrl Pts',(-64.9456450378036,61.2112859258266,-3.));
#35597=CARTESIAN_POINT('Ctrl Pts',(-64.9263786426945,61.3165318579407,-3.));
#35598=CARTESIAN_POINT('Ctrl Pts',(-63.6032183801568,63.6078550836889,-3.));
#35599=CARTESIAN_POINT('Ctrl Pts',(-63.4898427047886,63.7040964640175,-3.));
#35600=CARTESIAN_POINT('Ctrl Pts',(-63.3723224036437,63.7951365693987,-3.));
#35601=CARTESIAN_POINT('Ctrl Pts',(-63.2510558032013,63.8807935742749,-3.));
#35602=CARTESIAN_POINT('Ctrl Pts',(-63.1296781818555,63.9665289990789,-3.));
#35603=CARTESIAN_POINT('Ctrl Pts',(-63.0045466465185,64.04687175851,-3.));
#35604=CARTESIAN_POINT('Ctrl Pts',(-62.8760397174998,64.1215919436791,-3.));
#35605=CARTESIAN_POINT('Ctrl Pts',(-62.819687934894,64.1543576136944,-3.));
#35606=CARTESIAN_POINT('Ctrl Pts',(-62.7626868867519,64.1860414629978,-3.));
#35607=CARTESIAN_POINT('Ctrl Pts',(-62.7050677894913,64.216620998216,-3.));
#35608=CARTESIAN_POINT('Ctrl Pts',(-62.6757305642214,64.2321908137112,-3.));
#35609=CARTESIAN_POINT('Ctrl Pts',(-62.6462331101221,64.2474743135493,-3.));
#35610=CARTESIAN_POINT('Ctrl Pts',(-62.6165795271981,64.2624683312761,-3.));
#35611=CARTESIAN_POINT('Ctrl Pts',(-62.59496584419,64.2733970594164,-3.));
#35612=CARTESIAN_POINT('Ctrl Pts',(-62.5732698259174,64.2841716159096,-3.));
#35613=CARTESIAN_POINT('Ctrl Pts',(-62.5515051394286,64.2947850862267,-3.));
#35614=CARTESIAN_POINT('Ctrl Pts',(-62.4199917799758,64.3589170983083,-3.));
#35615=CARTESIAN_POINT('Ctrl Pts',(-62.2858583448011,64.4172297974733,-3.));
#35616=CARTESIAN_POINT('Ctrl Pts',(-62.1494741073268,64.4695125788851,-3.00000000000001));
#35617=CARTESIAN_POINT('Ctrl Pts',(-62.0315668791431,64.514712214504,-3.00000000000001));
#35618=CARTESIAN_POINT('Ctrl Pts',(-61.9119768383841,64.5554044377229,-3.));
#35619=CARTESIAN_POINT('Ctrl Pts',(-61.7909377316812,64.591421820407,-3.));
#35620=CARTESIAN_POINT('Ctrl Pts',(-61.7304181783297,64.6094305117491,-3.));
#35621=CARTESIAN_POINT('Ctrl Pts',(-61.6695363247516,64.6262700253364,-3.));
#35622=CARTESIAN_POINT('Ctrl Pts',(-61.6083214049011,64.6419165450135,-3.));
#35623=CARTESIAN_POINT('Ctrl Pts',(-61.5794890944997,64.649286077035,-3.));
#35624=CARTESIAN_POINT('Ctrl Pts',(-61.550582897767,64.6563909242344,-3.00000000000001));
#35625=CARTESIAN_POINT('Ctrl Pts',(-61.5216058842317,64.6632284448234,-3.00000000000001));
#35626=CARTESIAN_POINT('Ctrl Pts',(-61.4953410603476,64.6694259873636,-3.00000000000001));
#35627=CARTESIAN_POINT('Ctrl Pts',(-61.469014170971,64.6754046622799,-3.00000000000001));
#35628=CARTESIAN_POINT('Ctrl Pts',(-61.4426540829023,64.6811568975394,-3.00000000000001));
#35629=CARTESIAN_POINT('Ctrl Pts',(-61.4363509969477,64.6825323418542,-3.00000000000001));
#35630=CARTESIAN_POINT('Ctrl Pts',(-61.4300457323711,64.6838949091617,-3.));
#35631=CARTESIAN_POINT('Ctrl Pts',(-61.42373832106,64.6852445838374,-3.));
#35632=CARTESIAN_POINT('Ctrl Pts',(-61.2841863671008,64.7151062384725,-3.));
#35633=CARTESIAN_POINT('Ctrl Pts',(-61.1435842168792,64.738661067728,-3.));
#35634=CARTESIAN_POINT('Ctrl Pts',(-61.0023536947464,64.7559647413526,-3.));
#35635=CARTESIAN_POINT('Ctrl Pts',(-60.8601843546744,64.7733834396827,-3.));
#35636=CARTESIAN_POINT('Ctrl Pts',(-60.7173774438576,64.7844675371285,-3.00000000000001));
#35637=CARTESIAN_POINT('Ctrl Pts',(-60.5743624263688,64.7892212361641,-3.));
#35638=CARTESIAN_POINT('Ctrl Pts',(-60.4327942671285,64.793926842847,-3.));
#35639=CARTESIAN_POINT('Ctrl Pts',(-60.2910214307437,64.7924293018697,-3.));
#35640=CARTESIAN_POINT('Ctrl Pts',(-60.1494714253414,64.7846834160485,-3.));
#35641=CARTESIAN_POINT('Ctrl Pts',(-60.0601034197739,64.7797930286181,-3.));
#35642=CARTESIAN_POINT('Ctrl Pts',(-59.9708244934901,64.7724110370496,-3.));
#35643=CARTESIAN_POINT('Ctrl Pts',(-59.8817465640546,64.7625162762205,-3.));
#35644=CARTESIAN_POINT('Ctrl Pts',(-59.814938116978,64.7550952055987,-3.));
#35645=CARTESIAN_POINT('Ctrl Pts',(-59.7482427964903,64.7462605465847,-3.));
#35646=CARTESIAN_POINT('Ctrl Pts',(-59.6817095175338,64.7360006295818,-3.));
#35647=CARTESIAN_POINT('Ctrl Pts',(-59.6640767189296,64.7332815233984,-3.));
#35648=CARTESIAN_POINT('Ctrl Pts',(-59.6464553105021,64.7304622990051,-3.));
#35649=CARTESIAN_POINT('Ctrl Pts',(-59.6288462227171,64.7275427118551,-3.));
#35650=CARTESIAN_POINT('Ctrl Pts',(-59.6106484511471,64.7245255209203,-3.));
#35651=CARTESIAN_POINT('Ctrl Pts',(-59.5924725145907,64.7214025728485,-3.));
#35652=CARTESIAN_POINT('Ctrl Pts',(-59.5743219713167,64.7181743788859,-3.));
#35653=CARTESIAN_POINT('Ctrl Pts',(-59.437011224799,64.6937527560055,-3.));
#35654=CARTESIAN_POINT('Ctrl Pts',(-59.3011032400431,64.6633037588374,-3.));
#35655=CARTESIAN_POINT('Ctrl Pts',(-59.1669957960977,64.6268298783159,-3.));
#35656=CARTESIAN_POINT('Ctrl Pts',(-59.1418079969122,64.6199794250445,-3.));
#35657=CARTESIAN_POINT('Ctrl Pts',(-59.1166837551122,64.6129162986319,-3.));
#35658=CARTESIAN_POINT('Ctrl Pts',(-59.0916257724331,64.6056403204325,-3.));
#35659=CARTESIAN_POINT('Ctrl Pts',(-58.9576617080805,64.5667417536875,-3.));
#35660=CARTESIAN_POINT('Ctrl Pts',(-58.8255893248946,64.5217632196472,-3.));
#35661=CARTESIAN_POINT('Ctrl Pts',(-58.6957822301981,64.4709134387138,-3.));
#35662=CARTESIAN_POINT('Ctrl Pts',(-58.5664088958796,64.4202335762294,-3.));
#35663=CARTESIAN_POINT('Ctrl Pts',(-58.4392850870446,64.3637211364018,-3.));
#35664=CARTESIAN_POINT('Ctrl Pts',(-58.3148123421965,64.30154212406,-3.));
#35665=CARTESIAN_POINT('Ctrl Pts',(-58.2087252528553,64.2485474669124,-3.));
#35666=CARTESIAN_POINT('Ctrl Pts',(-58.104564199881,64.1914357758367,-3.));
#35667=CARTESIAN_POINT('Ctrl Pts',(-58.0026013403148,64.1302904539437,-3.));
#35668=CARTESIAN_POINT('Ctrl Pts',(-57.9842571522572,64.119289769102,-3.));
#35669=CARTESIAN_POINT('Ctrl Pts',(-57.9659841788218,64.1081584832539,-3.));
#35670=CARTESIAN_POINT('Ctrl Pts',(-57.947784091658,64.096897029522,-3.));
#35671=CARTESIAN_POINT('Ctrl Pts',(-57.9313889544622,64.0867524034388,-3.));
#35672=CARTESIAN_POINT('Ctrl Pts',(-57.9150608170848,64.0765069865091,-3.));
#35673=CARTESIAN_POINT('Ctrl Pts',(-57.8988040840088,64.0661635692336,-3.));
#35674=CARTESIAN_POINT('Ctrl Pts',(-57.7839055897439,63.9930589014656,-3.));
#35675=CARTESIAN_POINT('Ctrl Pts',(-57.6725153265955,63.9150275507377,-3.));
#35676=CARTESIAN_POINT('Ctrl Pts',(-57.5649776150316,63.8322713084228,-3.));
#35677=CARTESIAN_POINT('Ctrl Pts',(-57.4583964036554,63.7502511461319,-3.));
#35678=CARTESIAN_POINT('Ctrl Pts',(-57.3555989638067,63.6635892415037,-3.));
#35679=CARTESIAN_POINT('Ctrl Pts',(-57.2569565386241,63.5724461284644,-3.));
#35680=CARTESIAN_POINT('Ctrl Pts',(-57.2241738685229,63.5421557680923,-3.));
#35681=CARTESIAN_POINT('Ctrl Pts',(-57.1918504478657,63.5113702013341,-3.));
#35682=CARTESIAN_POINT('Ctrl Pts',(-57.160000955263,63.4800945823787,-3.));
#35683=CARTESIAN_POINT('Ctrl Pts',(-57.0634278031584,63.385261514103,-3.));
#35684=CARTESIAN_POINT('Ctrl Pts',(-56.9712084001481,63.285924190182,-3.));
#35685=CARTESIAN_POINT('Ctrl Pts',(-56.883615186019,63.182418835288,-3.));
#35686=CARTESIAN_POINT('Ctrl Pts',(-56.8363964827363,63.1266224052846,-3.));
#35687=CARTESIAN_POINT('Ctrl Pts',(-56.7905229461631,63.0696144344366,-3.));
#35688=CARTESIAN_POINT('Ctrl Pts',(-56.746043369936,63.0114459376167,-3.));
#35689=CARTESIAN_POINT('Ctrl Pts',(-56.7284856436537,62.9884846904095,-3.));
#35690=CARTESIAN_POINT('Ctrl Pts',(-56.7111451693665,62.9653426048408,-3.));
#35691=CARTESIAN_POINT('Ctrl Pts',(-56.6940251437079,62.9420227923607,-3.));
#35692=CARTESIAN_POINT('Ctrl Pts',(-56.6800433710512,62.9229777089597,-3.));
#35693=CARTESIAN_POINT('Ctrl Pts',(-56.6662062873437,62.9038106341118,-3.));
#35694=CARTESIAN_POINT('Ctrl Pts',(-56.6525316070086,62.8845461048891,-3.));
#35695=CARTESIAN_POINT('Ctrl Pts',(-56.5757647893409,62.776399035557,-3.));
#35696=CARTESIAN_POINT('Ctrl Pts',(-56.5040156403888,62.6650546667281,-3.));
#35697=CARTESIAN_POINT('Ctrl Pts',(-56.4374818016433,62.5508627236001,-3.));
#35698=CARTESIAN_POINT('Ctrl Pts',(-56.371191044164,62.4370879805415,-3.));
#35699=CARTESIAN_POINT('Ctrl Pts',(-56.3100772593781,62.3204856755393,-3.));
#35700=CARTESIAN_POINT('Ctrl Pts',(-56.2543835497104,62.2013821593283,-3.));
#35701=CARTESIAN_POINT('Ctrl Pts',(-56.199678842756,62.0843936701357,-3.));
#35702=CARTESIAN_POINT('Ctrl Pts',(-56.1502032662197,61.9649913135364,-3.));
#35703=CARTESIAN_POINT('Ctrl Pts',(-56.106236400397,61.8434762599769,-3.));
#35704=CARTESIAN_POINT('Ctrl Pts',(-56.0839234706096,61.7818080740045,-3.));
#35705=CARTESIAN_POINT('Ctrl Pts',(-56.0630301163055,61.7195956965504,-3.));
#35706=CARTESIAN_POINT('Ctrl Pts',(-56.0435980583969,61.6568785281303,-3.));
#35707=CARTESIAN_POINT('Ctrl Pts',(-56.0170092286204,61.5710628042873,-3.));
#35708=CARTESIAN_POINT('Ctrl Pts',(-55.9931559383444,61.4843017840239,-3.));
#35709=CARTESIAN_POINT('Ctrl Pts',(-55.9720760437321,61.396731441251,-3.));
#35710=CARTESIAN_POINT('Origin',(-60.,60.,-13.3123464956316));
#35711=CARTESIAN_POINT('Ctrl Pts',(-54.9007451799907,60.0000912485532,-9.56234649563159));
#35712=CARTESIAN_POINT('Ctrl Pts',(-54.9006553198669,60.1069729386028,-9.55734157105846));
#35713=CARTESIAN_POINT('Ctrl Pts',(-54.9296017816049,61.0460695450124,-9.51336443385491));
#35714=CARTESIAN_POINT('Ctrl Pts',(-55.4826600663013,62.7859966694522,-9.43041508402092));
#35715=CARTESIAN_POINT('Ctrl Pts',(-57.3241694659746,64.5834554691913,-9.31349844612963));
#35716=CARTESIAN_POINT('Ctrl Pts',(-59.7947368645222,65.3033954038122,-9.19658180823834));
#35717=CARTESIAN_POINT('Ctrl Pts',(-62.3135594152741,64.7765654229855,-9.07966517034706));
#35718=CARTESIAN_POINT('Ctrl Pts',(-64.2884897335979,63.1268180153125,-8.96274853245577));
#35719=CARTESIAN_POINT('Ctrl Pts',(-65.2552436145005,60.7419901177753,-8.84583189456448));
#35720=CARTESIAN_POINT('Ctrl Pts',(-64.9865478950058,58.1827288524753,-8.72891525667319));
#35721=CARTESIAN_POINT('Ctrl Pts',(-63.5455699950673,56.0506873380101,-8.61199861878189));
#35722=CARTESIAN_POINT('Ctrl Pts',(-61.2710678117403,54.8470867175201,-8.49508198089061));
#35723=CARTESIAN_POINT('Ctrl Pts',(-58.6977517313953,54.8548763465959,-8.37816534299932));
#35724=CARTESIAN_POINT('Ctrl Pts',(-56.4305796456292,56.0722332088069,-8.26124870510802));
#35725=CARTESIAN_POINT('Ctrl Pts',(-55.1447571773361,57.9997588942346,-8.15597575598546));
#35726=CARTESIAN_POINT('Ctrl Pts',(-54.901652700544,59.4163727828879,-8.08967501949331));
#35727=CARTESIAN_POINT('Ctrl Pts',(-54.9011518189288,60.0001169870244,-8.06234649563159));
#35728=CARTESIAN_POINT('Ctrl Pts',(-54.9012106446239,60.0001195814448,-9.68765350436841));
#35729=CARTESIAN_POINT('Ctrl Pts',(-54.9010041693968,60.2735579920353,-9.67485236502099));
#35730=CARTESIAN_POINT('Ctrl Pts',(-54.988526949539,61.3793291690848,-9.62307901304313));
#35731=CARTESIAN_POINT('Ctrl Pts',(-55.7768178011049,63.214507276628,-9.53233344843484));
#35732=CARTESIAN_POINT('Ctrl Pts',(-57.7853302019076,64.8232034014141,-9.41541681054356));
#35733=CARTESIAN_POINT('Ctrl Pts',(-60.3144620657417,65.2980444973094,-9.29850017265226));
#35734=CARTESIAN_POINT('Ctrl Pts',(-62.769679003779,64.5273620844534,-9.18158353476097));
#35735=CARTESIAN_POINT('Ctrl Pts',(-64.5737697114167,62.6923525936502,-9.06466689686969));
#35736=CARTESIAN_POINT('Ctrl Pts',(-65.3026202914353,60.2243982367199,-8.94775025897839));
#35737=CARTESIAN_POINT('Ctrl Pts',(-64.7848823971216,57.703691543606,-8.83083362108711));
#35738=CARTESIAN_POINT('Ctrl Pts',(-63.1422721706319,55.7228209792253,-8.71391698319582));
#35739=CARTESIAN_POINT('Ctrl Pts',(-60.7609482860978,54.7474681235472,-8.59700034530452));
#35740=CARTESIAN_POINT('Ctrl Pts',(-58.2007340318709,55.0069271910455,-8.48008370741324));
#35741=CARTESIAN_POINT('Ctrl Pts',(-56.0635071617532,56.4402025452955,-8.36316706952194));
#35742=CARTESIAN_POINT('Ctrl Pts',(-55.0531942753161,58.3328863911516,-8.26569033517368));
#35743=CARTESIAN_POINT('Ctrl Pts',(-54.9013976405776,59.5827292162986,-8.20718581345583));
#35744=CARTESIAN_POINT('Ctrl Pts',(-54.9013950998961,60.0000009027484,-8.18765350436842));
#35745=CARTESIAN_POINT('Ctrl Pts',(-63.2233527839579,62.7898325810254,-10.));
#35746=CARTESIAN_POINT('Ctrl Pts',(-63.6787829722545,62.2636317705077,-9.96102778736957));
#35747=CARTESIAN_POINT('Ctrl Pts',(-64.3265773596221,60.9843937251917,-9.88308336210871));
#35748=CARTESIAN_POINT('Ctrl Pts',(-64.2810882745412,58.8332762706057,-9.76616672421742));
#35749=CARTESIAN_POINT('Ctrl Pts',(-63.229077517363,56.9567113445499,-9.64925008632613));
#35750=CARTESIAN_POINT('Ctrl Pts',(-61.41796272213,55.7954439251957,-9.53233344843485));
#35751=CARTESIAN_POINT('Ctrl Pts',(-59.2734876021215,55.622683427384,-9.41541681054355));
#35752=CARTESIAN_POINT('Ctrl Pts',(-57.2998122688331,56.4789515210604,-9.29850017265226));
#35753=CARTESIAN_POINT('Ctrl Pts',(-55.96091867892,58.1629927736796,-9.18158353476098));
#35754=CARTESIAN_POINT('Ctrl Pts',(-55.5715694755394,60.2788877013121,-9.06466689686968));
#35755=CARTESIAN_POINT('Ctrl Pts',(-56.223294736741,62.3292221615758,-8.94775025897839));
#35756=CARTESIAN_POINT('Ctrl Pts',(-57.7628818265247,63.8319809109948,-8.8308336210871));
#35757=CARTESIAN_POINT('Ctrl Pts',(-59.8283905184268,64.433884017739,-8.71391698319582));
#35758=CARTESIAN_POINT('Ctrl Pts',(-61.9342427509931,63.9934297701877,-8.59700034530453));
#35759=CARTESIAN_POINT('Ctrl Pts',(-63.585375903967,62.6141645811487,-8.48008370741324));
#35760=CARTESIAN_POINT('Ctrl Pts',(-64.393626893237,60.6203380804229,-8.36316706952195));
#35761=CARTESIAN_POINT('Ctrl Pts',(-64.1689848355383,58.4806772108457,-8.24625043163066));
#35762=CARTESIAN_POINT('Ctrl Pts',(-62.9642606175665,56.6981918262281,-8.12933379373937));
#35763=CARTESIAN_POINT('Ctrl Pts',(-61.06267152019,55.6919260005468,-8.01241715584808));
#35764=CARTESIAN_POINT('Ctrl Pts',(-58.9112601747281,55.6984384909861,-7.89550051795679));
#35765=CARTESIAN_POINT('Ctrl Pts',(-57.0157993781756,56.7162051714344,-7.7785838800655));
#35766=CARTESIAN_POINT('Ctrl Pts',(-55.8218913855027,58.5059454961382,-7.66166724217421));
#35767=CARTESIAN_POINT('Ctrl Pts',(-55.610209865439,60.6469434343234,-7.54475060428292));
#35768=CARTESIAN_POINT('Ctrl Pts',(-56.4305207028874,62.6358047497177,-7.42783396639163));
#35769=CARTESIAN_POINT('Ctrl Pts',(-58.0899737944543,64.0051198695055,-7.31091732850034));
#35770=CARTESIAN_POINT('Ctrl Pts',(-60.1984589714611,64.4326546672265,-7.19400069060905));
#35771=CARTESIAN_POINT('Ctrl Pts',(-62.2602755751237,63.8185984946696,-7.07708405271776));
#35772=CARTESIAN_POINT('Ctrl Pts',(-63.7907548362926,62.3058012416029,-6.96016741482647));
#35773=CARTESIAN_POINT('Ctrl Pts',(-64.4300091285896,60.2531589262444,-6.84325077693518));
#35774=CARTESIAN_POINT('Ctrl Pts',(-64.0279514449107,58.1361887346157,-6.72633413904389));
#35775=CARTESIAN_POINT('Ctrl Pts',(-62.6787003804465,56.4677145273824,-6.60941750115261));
#35776=CARTESIAN_POINT('Ctrl Pts',(-60.040721219432,55.3204109471847,-6.45352865063089));
#35777=CARTESIAN_POINT('Ctrl Pts',(-56.3381268516022,56.5785262980586,-6.25866758747874));
#35778=CARTESIAN_POINT('Ctrl Pts',(-55.1221049889056,61.1497554125864,-6.02483431169616));
#35779=CARTESIAN_POINT('Ctrl Pts',(-57.7101830808087,64.0812927360737,-5.82997324854401));
#35780=CARTESIAN_POINT('Ctrl Pts',(-60.5695473859375,64.3963726142629,-5.67408439802229));
#35781=CARTESIAN_POINT('Ctrl Pts',(-62.569477548857,63.6188355035077,-5.557167760131));
#35782=CARTESIAN_POINT('Ctrl Pts',(-63.9702556002071,61.9814491642124,-5.44025112223971));
#35783=CARTESIAN_POINT('Ctrl Pts',(-64.435395460414,59.8824895563441,-5.32333448434842));
#35784=CARTESIAN_POINT('Ctrl Pts',(-63.8588751572395,57.8091958873783,-5.20641784645713));
#35785=CARTESIAN_POINT('Ctrl Pts',(-62.374688490879,56.2518447292755,-5.08950120856584));
#35786=CARTESIAN_POINT('Ctrl Pts',(-60.3324645529654,55.5752228761179,-4.97258457067455));
#35787=CARTESIAN_POINT('Ctrl Pts',(-58.2119773478597,55.93901192728,-4.85566793278326));
#35788=CARTESIAN_POINT('Ctrl Pts',(-56.5118828738941,57.2574041226595,-4.73875129489197));
#35789=CARTESIAN_POINT('Ctrl Pts',(-55.631783700059,59.2205920103183,-4.62183465700068));
#35790=CARTESIAN_POINT('Ctrl Pts',(-55.778614193939,61.366990745641,-4.50491801910939));
#35791=CARTESIAN_POINT('Ctrl Pts',(-56.9178409418314,63.1920340492318,-4.3880013812181));
#35792=CARTESIAN_POINT('Ctrl Pts',(-58.781651390282,64.2666613413666,-4.27108474332681));
#35793=CARTESIAN_POINT('Ctrl Pts',(-60.9318810632418,64.3382457169127,-4.15416810543552));
#35794=CARTESIAN_POINT('Ctrl Pts',(-62.8630363220205,63.3899556613623,-4.03725146754423));
#35795=CARTESIAN_POINT('Ctrl Pts',(-64.1211231584726,61.6447249909761,-3.92033482965295));
#35796=CARTESIAN_POINT('Ctrl Pts',(-64.4103798056068,59.5128374617724,-3.80341819176165));
#35797=CARTESIAN_POINT('Ctrl Pts',(-63.6628046569468,57.4954766114706,-3.68650155387037));
#35798=CARTESIAN_POINT('Ctrl Pts',(-62.0541453323136,56.0669012832628,-3.56958491597908));
#35799=CARTESIAN_POINT('Ctrl Pts',(-59.9625778285317,55.5629542684651,-3.45266827808779));
#35800=CARTESIAN_POINT('Ctrl Pts',(-57.8798107643185,56.1021068410437,-3.3357516401965));
#35801=CARTESIAN_POINT('Ctrl Pts',(-56.2954704227517,57.5576124826779,-3.21883500230521));
#35802=CARTESIAN_POINT('Ctrl Pts',(-55.5820374028276,59.5872929237356,-3.10191836441392));
#35803=CARTESIAN_POINT('Ctrl Pts',(-55.9071888205857,61.7140031265185,-2.98500172652263));
#35804=CARTESIAN_POINT('Ctrl Pts',(-57.1945760881725,63.437752772978,-2.86808508863134));
#35805=CARTESIAN_POINT('Ctrl Pts',(-59.1413430300255,64.3533515000793,-2.75116845074005));
#35806=CARTESIAN_POINT('Ctrl Pts',(-61.2902326596918,64.2454213381917,-2.63425181284876));
#35807=CARTESIAN_POINT('Ctrl Pts',(-62.5200516280627,63.5081067174902,-2.5563073875879));
#35808=CARTESIAN_POINT('Ctrl Pts',(-63.0124573356753,63.0163338344314,-2.51733517495747));
#35809=CARTESIAN_POINT('Ctrl Pts',(-63.4340590883905,62.9722002436837,-10.1608882750142));
#35810=CARTESIAN_POINT('Ctrl Pts',(-63.9192601452004,62.4116023827638,-10.1219160623837));
#35811=CARTESIAN_POINT('Ctrl Pts',(-64.609399994124,61.0487422398731,-10.0439716371229));
#35812=CARTESIAN_POINT('Ctrl Pts',(-64.5609373477695,58.7570090849169,-9.9270549992316));
#35813=CARTESIAN_POINT('Ctrl Pts',(-63.44015804004,56.7577755938301,-9.81013836134031));
#35814=CARTESIAN_POINT('Ctrl Pts',(-61.5106530681853,55.5205976605514,-9.69322172344902));
#35815=CARTESIAN_POINT('Ctrl Pts',(-59.2259964484248,55.336544037697,-9.57630508555773));
#35816=CARTESIAN_POINT('Ctrl Pts',(-57.1233045713387,56.2487852431346,-9.45938844766644));
#35817=CARTESIAN_POINT('Ctrl Pts',(-55.6968892798722,58.0429100431139,-9.34247180977516));
#35818=CARTESIAN_POINT('Ctrl Pts',(-55.2820888344847,60.297118221157,-9.22555517188385));
#35819=CARTESIAN_POINT('Ctrl Pts',(-55.9764165132611,62.4814803308679,-9.10863853399257));
#35820=CARTESIAN_POINT('Ctrl Pts',(-57.616644373008,64.0824724303936,-8.99172189610128));
#35821=CARTESIAN_POINT('Ctrl Pts',(-59.817172633792,64.7237211464301,-8.87480525820999));
#35822=CARTESIAN_POINT('Ctrl Pts',(-62.0606816390868,64.254474987787,-8.7578886203187));
#35823=CARTESIAN_POINT('Ctrl Pts',(-63.8197471805106,62.7850490592033,-8.64097198242742));
#35824=CARTESIAN_POINT('Ctrl Pts',(-64.6808324669915,60.6608887595404,-8.52405534453612));
#35825=CARTESIAN_POINT('Ctrl Pts',(-64.4415058553609,58.3813610913889,-8.40713870664483));
#35826=CARTESIAN_POINT('Ctrl Pts',(-63.1580304100668,56.4823569968221,-8.29022206875354));
#35827=CARTESIAN_POINT('Ctrl Pts',(-61.1321369507068,55.4103129062046,-8.17330543086225));
#35828=CARTESIAN_POINT('Ctrl Pts',(-58.8400906936171,55.4172511095227,-8.05638879297097));
#35829=CARTESIAN_POINT('Ctrl Pts',(-56.8207261339935,56.5015478505586,-7.93947215507967));
#35830=CARTESIAN_POINT('Ctrl Pts',(-55.5487739563277,58.408281131041,-7.82255551718839));
#35831=CARTESIAN_POINT('Ctrl Pts',(-55.3232550955201,60.6892332702054,-7.70563887929709));
#35832=CARTESIAN_POINT('Ctrl Pts',(-56.19718856649,62.8081038169445,-7.58872224140581));
#35833=CARTESIAN_POINT('Ctrl Pts',(-57.9651179098787,64.2669292534219,-7.47180560351451));
#35834=CARTESIAN_POINT('Ctrl Pts',(-60.2114319717067,64.7224114349019,-7.35488896562323));
#35835=CARTESIAN_POINT('Ctrl Pts',(-62.4080267973306,64.0682152232288,-7.23797232773193));
#35836=CARTESIAN_POINT('Ctrl Pts',(-64.038551461763,62.4565284163609,-7.12105568984065));
#35837=CARTESIAN_POINT('Ctrl Pts',(-64.7195929609065,60.2697075901227,-7.00413905194936));
#35838=CARTESIAN_POINT('Ctrl Pts',(-64.291253298687,58.0143538594995,-6.88722241405807));
#35839=CARTESIAN_POINT('Ctrl Pts',(-62.8538034782691,56.2368137020554,-6.77030577616678));
#35840=CARTESIAN_POINT('Ctrl Pts',(-60.0433831116398,55.0145124056135,-6.61441692564506));
#35841=CARTESIAN_POINT('Ctrl Pts',(-56.0987550514566,56.3548690914888,-6.41955586249291));
#35842=CARTESIAN_POINT('Ctrl Pts',(-54.803243449358,61.224913401868,-6.18572258671033));
#35843=CARTESIAN_POINT('Ctrl Pts',(-57.5605007800468,64.3480814394404,-5.99086152355819));
#35844=CARTESIAN_POINT('Ctrl Pts',(-60.6067779445929,64.6837576721661,-5.83497267303646));
#35845=CARTESIAN_POINT('Ctrl Pts',(-62.7374408947671,63.8553939897797,-5.71805603514517));
#35846=CARTESIAN_POINT('Ctrl Pts',(-64.2297859529926,62.1109738730467,-5.60113939725388));
#35847=CARTESIAN_POINT('Ctrl Pts',(-64.7253313901119,59.8748080542019,-5.48422275936259));
#35848=CARTESIAN_POINT('Ctrl Pts',(-64.1111247179129,57.6659859227094,-5.36730612147131));
#35849=CARTESIAN_POINT('Ctrl Pts',(-62.5299187339296,56.0068327810132,-5.25038948358002));
#35850=CARTESIAN_POINT('Ctrl Pts',(-60.3541973206782,55.2859810530227,-5.13347284568872));
#35851=CARTESIAN_POINT('Ctrl Pts',(-58.0950966740627,55.6735505128775,-5.01655620779744));
#35852=CARTESIAN_POINT('Ctrl Pts',(-56.2838692749086,57.0781242607894,-4.89963956990615));
#35853=CARTESIAN_POINT('Ctrl Pts',(-55.3462391831499,59.1696431418083,-4.78272293201486));
#35854=CARTESIAN_POINT('Ctrl Pts',(-55.5026677920415,61.4563491210696,-4.66580629412357));
#35855=CARTESIAN_POINT('Ctrl Pts',(-56.7163642843423,63.400693089435,-4.54888965623228));
#35856=CARTESIAN_POINT('Ctrl Pts',(-58.7020095545072,64.5455673450715,-4.43197301834099));
#35857=CARTESIAN_POINT('Ctrl Pts',(-60.9927968947275,64.6218310964842,-4.3150563804497));
#35858=CARTESIAN_POINT('Ctrl Pts',(-63.0501892163211,63.611552575343,-4.19813974255841));
#35859=CARTESIAN_POINT('Ctrl Pts',(-64.3905155238243,61.7522384863594,-4.08122310466712));
#35860=CARTESIAN_POINT('Ctrl Pts',(-64.6986804950654,59.4809922915512,-3.96430646677583));
#35861=CARTESIAN_POINT('Ctrl Pts',(-63.9022373485731,57.3317592330352,-3.84738982888454));
#35862=CARTESIAN_POINT('Ctrl Pts',(-62.1884220934219,55.8097998267617,-3.73047319099325));
#35863=CARTESIAN_POINT('Ctrl Pts',(-59.960131590722,55.2729104627288,-3.61355655310196));
#35864=CARTESIAN_POINT('Ctrl Pts',(-57.7412168006756,55.8473067252498,-3.49663991521067));
#35865=CARTESIAN_POINT('Ctrl Pts',(-56.0533102283206,57.3979568438882,-3.37972327731939));
#35866=CARTESIAN_POINT('Ctrl Pts',(-55.2932410363222,59.5603148084993,-3.2628066394281));
#35867=CARTESIAN_POINT('Ctrl Pts',(-55.6396471718258,61.8260452419121,-3.1458900015368));
#35868=CARTESIAN_POINT('Ctrl Pts',(-57.0111892408593,63.6624741208715,-3.02897336364552));
#35869=CARTESIAN_POINT('Ctrl Pts',(-59.0852137605831,64.6379243246994,-2.91205672575423));
#35870=CARTESIAN_POINT('Ctrl Pts',(-61.3745734606538,64.5229389110065,-2.79514008786294));
#35871=CARTESIAN_POINT('Ctrl Pts',(-62.6847840669602,63.7374270096023,-2.71719566260208));
#35872=CARTESIAN_POINT('Ctrl Pts',(-63.2093776838358,63.2135075841839,-2.67822344997165));
#35873=CARTESIAN_POINT('Ctrl Pts',(-63.6447653928231,63.154567906342,-10.3217765500284));
#35874=CARTESIAN_POINT('Ctrl Pts',(-64.1597373181463,62.55957299502,-10.2828043373979));
#35875=CARTESIAN_POINT('Ctrl Pts',(-64.8922226286258,61.1130907545544,-10.2048599121371));
#35876=CARTESIAN_POINT('Ctrl Pts',(-64.8407864209977,58.6807418992281,-10.0879432742458));
#35877=CARTESIAN_POINT('Ctrl Pts',(-63.6512385627169,56.5588398431102,-9.97102663635448));
#35878=CARTESIAN_POINT('Ctrl Pts',(-61.6033434142406,55.2457513959071,-9.8541099984632));
#35879=CARTESIAN_POINT('Ctrl Pts',(-59.1785052947282,55.05040464801,-9.73719336057191));
#35880=CARTESIAN_POINT('Ctrl Pts',(-56.9467968738444,56.0186189652088,-9.62027672268061));
#35881=CARTESIAN_POINT('Ctrl Pts',(-55.4328598808243,57.9228273125483,-9.50336008478933));
#35882=CARTESIAN_POINT('Ctrl Pts',(-54.9926081934299,60.315348741002,-9.38644344689803));
#35883=CARTESIAN_POINT('Ctrl Pts',(-55.7295382897812,62.63373850016,-9.26952680900674));
#35884=CARTESIAN_POINT('Ctrl Pts',(-57.4704069194913,64.3329639497925,-9.15261017111546));
#35885=CARTESIAN_POINT('Ctrl Pts',(-59.8059547491571,65.0135582751211,-9.03569353322417));
#35886=CARTESIAN_POINT('Ctrl Pts',(-62.1871205271805,64.5155202053863,-8.91877689533288));
#35887=CARTESIAN_POINT('Ctrl Pts',(-64.0541184570542,62.9559335372579,-8.80186025744159));
#35888=CARTESIAN_POINT('Ctrl Pts',(-64.968038040746,60.7014394386578,-8.6849436195503));
#35889=CARTESIAN_POINT('Ctrl Pts',(-64.7140268751833,58.2820449719321,-8.56802698165901));
#35890=CARTESIAN_POINT('Ctrl Pts',(-63.351800202567,56.2665221674161,-8.45111034376772));
#35891=CARTESIAN_POINT('Ctrl Pts',(-61.2016023812236,55.1286998118624,-8.33419370587643));
#35892=CARTESIAN_POINT('Ctrl Pts',(-58.7689212125062,55.1360637280593,-8.21727706798515));
#35893=CARTESIAN_POINT('Ctrl Pts',(-56.6256528898113,56.2868905296827,-8.10036043009385));
#35894=CARTESIAN_POINT('Ctrl Pts',(-55.2756565271526,58.3106167659438,-7.98344379220257));
#35895=CARTESIAN_POINT('Ctrl Pts',(-55.0363003256012,60.7315231060873,-7.86652715431127));
#35896=CARTESIAN_POINT('Ctrl Pts',(-55.9638564300926,62.9804028841713,-7.74961051641998));
#35897=CARTESIAN_POINT('Ctrl Pts',(-57.8402620253032,64.5287386373382,-7.63269387852869));
#35898=CARTESIAN_POINT('Ctrl Pts',(-60.2244049719524,65.0121682025774,-7.51577724063741));
#35899=CARTESIAN_POINT('Ctrl Pts',(-62.5557780195374,64.317831951788,-7.39886060274611));
#35900=CARTESIAN_POINT('Ctrl Pts',(-64.2863480872334,62.6072555911189,-7.28194396485483));
#35901=CARTESIAN_POINT('Ctrl Pts',(-65.0091767932234,60.2862562540011,-7.16502732696354));
#35902=CARTESIAN_POINT('Ctrl Pts',(-64.5545551524633,57.8925189843833,-7.04811068907224));
#35903=CARTESIAN_POINT('Ctrl Pts',(-63.0289065760917,56.0059128767283,-6.93119405118096));
#35904=CARTESIAN_POINT('Ctrl Pts',(-60.0460450038475,54.7086138640423,-6.77530520065924));
#35905=CARTESIAN_POINT('Ctrl Pts',(-55.8593832513112,56.1312118849188,-6.58044413750709));
#35906=CARTESIAN_POINT('Ctrl Pts',(-54.4843819098103,61.3000713911496,-6.34661086172451));
#35907=CARTESIAN_POINT('Ctrl Pts',(-57.4108184792849,64.6148701428072,-6.15174979857236));
#35908=CARTESIAN_POINT('Ctrl Pts',(-60.6440085032482,64.9711427300693,-5.99586094805064));
#35909=CARTESIAN_POINT('Ctrl Pts',(-62.9054042406772,64.0919524760517,-5.87894431015935));
#35910=CARTESIAN_POINT('Ctrl Pts',(-64.489316305778,62.240498581881,-5.76202767226806));
#35911=CARTESIAN_POINT('Ctrl Pts',(-65.0152673198098,59.8671265520597,-5.64511103437677));
#35912=CARTESIAN_POINT('Ctrl Pts',(-64.3633742785863,57.5227759580404,-5.52819439648548));
#35913=CARTESIAN_POINT('Ctrl Pts',(-62.6851489769803,55.761820832751,-5.41127775859419));
#35914=CARTESIAN_POINT('Ctrl Pts',(-60.375930088391,54.9967392299274,-5.2943611207029));
#35915=CARTESIAN_POINT('Ctrl Pts',(-57.9782160002658,55.408089098475,-5.17744448281162));
#35916=CARTESIAN_POINT('Ctrl Pts',(-56.0558556759232,56.8988443989193,-5.06052784492033));
#35917=CARTESIAN_POINT('Ctrl Pts',(-55.0606946662407,59.1186942732983,-4.94361120702903));
#35918=CARTESIAN_POINT('Ctrl Pts',(-55.226721390144,61.5457074964981,-4.82669456913774));
#35919=CARTESIAN_POINT('Ctrl Pts',(-56.5148876268531,63.609352129638,-4.70977793124646));
#35920=CARTESIAN_POINT('Ctrl Pts',(-58.6223677187324,64.8244733487765,-4.59286129335517));
#35921=CARTESIAN_POINT('Ctrl Pts',(-61.0537127262131,64.9054164760556,-4.47594465546388));
#35922=CARTESIAN_POINT('Ctrl Pts',(-63.2373421106216,63.8331494893237,-4.35902801757258));
#35923=CARTESIAN_POINT('Ctrl Pts',(-64.659907889176,61.8597519817425,-4.2421113796813));
#35924=CARTESIAN_POINT('Ctrl Pts',(-64.9869811845242,59.4491471213301,-4.12519474179001));
#35925=CARTESIAN_POINT('Ctrl Pts',(-64.1416700401993,57.1680418545997,-4.00827810389872));
#35926=CARTESIAN_POINT('Ctrl Pts',(-62.3226988545302,55.5526983702606,-3.89136146600743));
#35927=CARTESIAN_POINT('Ctrl Pts',(-59.9576853529124,54.9828666569923,-3.77444482811614));
#35928=CARTESIAN_POINT('Ctrl Pts',(-57.6026228370326,55.592506609456,-3.65752819022485));
#35929=CARTESIAN_POINT('Ctrl Pts',(-55.8111500338895,57.2383012050985,-3.54061155233356));
#35930=CARTESIAN_POINT('Ctrl Pts',(-55.0044446698169,59.533336693263,-3.42369491444227));
#35931=CARTESIAN_POINT('Ctrl Pts',(-55.3721055230659,61.9380873573058,-3.30677827655098));
#35932=CARTESIAN_POINT('Ctrl Pts',(-56.8278023935462,63.8871954687649,-3.18986163865969));
#35933=CARTESIAN_POINT('Ctrl Pts',(-59.0290844911407,64.9224971493195,-3.0729450007684));
#35934=CARTESIAN_POINT('Ctrl Pts',(-61.4589142616157,64.8004564838213,-2.95602836287711));
#35935=CARTESIAN_POINT('Ctrl Pts',(-62.8495165058577,63.9667473017145,-2.87808393761625));
#35936=CARTESIAN_POINT('Ctrl Pts',(-63.4062980319963,63.4106813339364,-2.83911172498582));
#35937=CARTESIAN_POINT('Ctrl Pts',(-63.8554716972558,63.3369355690004,-10.4826648250425));
#35938=CARTESIAN_POINT('Ctrl Pts',(-64.4002144910922,62.7075436072762,-10.4436926124121));
#35939=CARTESIAN_POINT('Ctrl Pts',(-65.1750452631277,61.1774392692358,-10.3657481871512));
#35940=CARTESIAN_POINT('Ctrl Pts',(-65.120635494226,58.6044747135393,-10.24883154926));
#35941=CARTESIAN_POINT('Ctrl Pts',(-63.8623190853939,56.3599040923904,-10.1319149113687));
#35942=CARTESIAN_POINT('Ctrl Pts',(-61.6960337602958,54.9709051312627,-10.0149982734774));
#35943=CARTESIAN_POINT('Ctrl Pts',(-59.1310141410315,54.764265258323,-9.89808163558608));
#35944=CARTESIAN_POINT('Ctrl Pts',(-56.77028917635,55.7884526872829,-9.78116499769479));
#35945=CARTESIAN_POINT('Ctrl Pts',(-55.1688304817765,57.8027445819827,-9.6642483598035));
#35946=CARTESIAN_POINT('Ctrl Pts',(-54.7031275523752,60.3335792608469,-9.54733172191221));
#35947=CARTESIAN_POINT('Ctrl Pts',(-55.4826600663013,62.7859966694522,-9.43041508402092));
#35948=CARTESIAN_POINT('Ctrl Pts',(-57.3241694659746,64.5834554691913,-9.31349844612963));
#35949=CARTESIAN_POINT('Ctrl Pts',(-59.7947368645222,65.3033954038122,-9.19658180823834));
#35950=CARTESIAN_POINT('Ctrl Pts',(-62.3135594152741,64.7765654229855,-9.07966517034706));
#35951=CARTESIAN_POINT('Ctrl Pts',(-64.2884897335979,63.1268180153125,-8.96274853245577));
#35952=CARTESIAN_POINT('Ctrl Pts',(-65.2552436145005,60.7419901177753,-8.84583189456448));
#35953=CARTESIAN_POINT('Ctrl Pts',(-64.9865478950058,58.1827288524753,-8.72891525667319));
#35954=CARTESIAN_POINT('Ctrl Pts',(-63.5455699950673,56.0506873380101,-8.61199861878189));
#35955=CARTESIAN_POINT('Ctrl Pts',(-61.2710678117403,54.8470867175201,-8.49508198089061));
#35956=CARTESIAN_POINT('Ctrl Pts',(-58.6977517313953,54.8548763465959,-8.37816534299932));
#35957=CARTESIAN_POINT('Ctrl Pts',(-56.4305796456292,56.0722332088069,-8.26124870510802));
#35958=CARTESIAN_POINT('Ctrl Pts',(-55.0025390979776,58.2129524008466,-8.14433206721674));
#35959=CARTESIAN_POINT('Ctrl Pts',(-54.7493455556822,60.7738129419693,-8.02741542932545));
#35960=CARTESIAN_POINT('Ctrl Pts',(-55.7305242936952,63.1527019513981,-7.91049879143416));
#35961=CARTESIAN_POINT('Ctrl Pts',(-57.7154061407277,64.7905480212547,-7.79358215354287));
#35962=CARTESIAN_POINT('Ctrl Pts',(-60.237377972198,65.3019249702528,-7.67666551565158));
#35963=CARTESIAN_POINT('Ctrl Pts',(-62.7035292417443,64.5674486803472,-7.55974887776029));
#35964=CARTESIAN_POINT('Ctrl Pts',(-64.5341447127037,62.7579827658769,-7.442832239869));
#35965=CARTESIAN_POINT('Ctrl Pts',(-65.2987606255403,60.3028049178794,-7.32591560197772));
#35966=CARTESIAN_POINT('Ctrl Pts',(-64.8178570062396,57.770684109267,-7.20899896408642));
#35967=CARTESIAN_POINT('Ctrl Pts',(-63.2040096739143,55.7750120514012,-7.09208232619513));
#35968=CARTESIAN_POINT('Ctrl Pts',(-60.0487068960553,54.4027153224711,-6.93619347567341));
#35969=CARTESIAN_POINT('Ctrl Pts',(-55.6200114511657,55.9075546783489,-6.74133241252127));
#35970=CARTESIAN_POINT('Ctrl Pts',(-54.1655203702626,61.3752293804312,-6.50749913673868));
#35971=CARTESIAN_POINT('Ctrl Pts',(-57.261136178523,64.881658846174,-6.31263807358654));
#35972=CARTESIAN_POINT('Ctrl Pts',(-60.6812390619036,65.2585277879725,-6.15674922306482));
#35973=CARTESIAN_POINT('Ctrl Pts',(-63.0733675865873,64.3285109623237,-6.03983258517352));
#35974=CARTESIAN_POINT('Ctrl Pts',(-64.7488466585635,62.3700232907153,-5.92291594728224));
#35975=CARTESIAN_POINT('Ctrl Pts',(-65.3052032495076,59.8594450499176,-5.80599930939095));
#35976=CARTESIAN_POINT('Ctrl Pts',(-64.6156238392598,57.3795659933714,-5.68908267149965));
#35977=CARTESIAN_POINT('Ctrl Pts',(-62.8403792200309,55.5168088844888,-5.57216603360837));
#35978=CARTESIAN_POINT('Ctrl Pts',(-60.3976628561038,54.7074974068321,-5.45524939571708));
#35979=CARTESIAN_POINT('Ctrl Pts',(-57.8613353264688,55.1426276840725,-5.33833275782579));
#35980=CARTESIAN_POINT('Ctrl Pts',(-55.8278420769378,56.7195645370492,-5.2214161199345));
#35981=CARTESIAN_POINT('Ctrl Pts',(-54.7751501493316,59.0677454047883,-5.10449948204321));
#35982=CARTESIAN_POINT('Ctrl Pts',(-54.9507749882465,61.6350658719267,-4.98758284415192));
#35983=CARTESIAN_POINT('Ctrl Pts',(-56.3134109693639,63.8180111698412,-4.87066620626063));
#35984=CARTESIAN_POINT('Ctrl Pts',(-58.5427258829576,65.1033793524814,-4.75374956836935));
#35985=CARTESIAN_POINT('Ctrl Pts',(-61.1146285576988,65.189001855627,-4.63683293047805));
#35986=CARTESIAN_POINT('Ctrl Pts',(-63.4244950049221,64.0547464033043,-4.51991629258676));
#35987=CARTESIAN_POINT('Ctrl Pts',(-64.9293002545277,61.9672654771257,-4.40299965469547));
#35988=CARTESIAN_POINT('Ctrl Pts',(-65.2752818739828,59.417301951109,-4.28608301680418));
#35989=CARTESIAN_POINT('Ctrl Pts',(-64.3811027318255,57.0043244761643,-4.1691663789129));
#35990=CARTESIAN_POINT('Ctrl Pts',(-62.4569756156385,55.2955969137595,-4.0522497410216));
#35991=CARTESIAN_POINT('Ctrl Pts',(-59.9552391151028,54.6928228512559,-3.93533310313032));
#35992=CARTESIAN_POINT('Ctrl Pts',(-57.4640288733897,55.3377064936621,-3.81841646523903));
#35993=CARTESIAN_POINT('Ctrl Pts',(-55.5689898394584,57.0786455663088,-3.70149982734774));
#35994=CARTESIAN_POINT('Ctrl Pts',(-54.7156483033116,59.5063585780268,-3.58458318945645));
#35995=CARTESIAN_POINT('Ctrl Pts',(-55.104563874306,62.0501294726994,-3.46766655156516));
#35996=CARTESIAN_POINT('Ctrl Pts',(-56.644415546233,64.1119168166584,-3.35074991367387));
#35997=CARTESIAN_POINT('Ctrl Pts',(-58.9729552216983,65.2070699739396,-3.23383327578258));
#35998=CARTESIAN_POINT('Ctrl Pts',(-61.5432550625777,65.077974056636,-3.11691663789129));
#35999=CARTESIAN_POINT('Ctrl Pts',(-63.0142489447552,64.1960675938266,-3.03897221263043));
#36000=CARTESIAN_POINT('Ctrl Pts',(-63.6032183801568,63.6078550836889,-3.));
#36001=CARTESIAN_POINT('Ctrl Pts',(-63.2233527839579,62.7898325810254,-10.));
#36002=CARTESIAN_POINT('Ctrl Pts',(-63.3163082252117,62.7013635452477,-10.));
#36003=CARTESIAN_POINT('Ctrl Pts',(-63.4049730364641,62.6087978162202,-10.));
#36004=CARTESIAN_POINT('Ctrl Pts',(-63.489228887801,62.5125540616361,-10.));
#36005=CARTESIAN_POINT('Ctrl Pts',(-63.5750437123066,62.4145295235377,-10.));
#36006=CARTESIAN_POINT('Ctrl Pts',(-63.6562854342097,62.3126891791932,-10.));
#36007=CARTESIAN_POINT('Ctrl Pts',(-63.7328061009133,62.2074264239704,-10.));
#36008=CARTESIAN_POINT('Ctrl Pts',(-63.8104263008827,62.1006511374799,-10.));
#36009=CARTESIAN_POINT('Ctrl Pts',(-63.8831893713456,61.9903538684369,-10.));
#36010=CARTESIAN_POINT('Ctrl Pts',(-63.9509091476781,61.8769024196434,-10.));
#36011=CARTESIAN_POINT('Ctrl Pts',(-64.0184810129676,61.7636987673289,-10.));
#36012=CARTESIAN_POINT('Ctrl Pts',(-64.0810321009563,61.647354054786,-10.));
#36013=CARTESIAN_POINT('Ctrl Pts',(-64.1383380480206,61.5282002475095,-10.));
#36014=CARTESIAN_POINT('Ctrl Pts',(-64.1498926000478,61.5041753611593,-10.));
#36015=CARTESIAN_POINT('Ctrl Pts',(-64.1612337714855,61.4800361822972,-10.));
#36016=CARTESIAN_POINT('Ctrl Pts',(-64.1723594994649,61.4557853033111,-10.));
#36017=CARTESIAN_POINT('Ctrl Pts',(-64.1825650553464,61.4335401341746,-10.));
#36018=CARTESIAN_POINT('Ctrl Pts',(-64.192591209754,61.4111964786891,-10.));
#36019=CARTESIAN_POINT('Ctrl Pts',(-64.2024244346998,61.3887840242283,-10.));
#36020=CARTESIAN_POINT('Ctrl Pts',(-64.2596369074205,61.2583820506629,-10.));
#36021=CARTESIAN_POINT('Ctrl Pts',(-64.3103965387496,61.1254981286836,-10.));
#36022=CARTESIAN_POINT('Ctrl Pts',(-64.3545197254654,60.9906065311624,-10.));
#36023=CARTESIAN_POINT('Ctrl Pts',(-64.3960228498109,60.8637248809054,-10.));
#36024=CARTESIAN_POINT('Ctrl Pts',(-64.4316548200294,60.7350659665181,-10.));
#36025=CARTESIAN_POINT('Ctrl Pts',(-64.4614760030326,60.6050515502419,-10.));
#36026=CARTESIAN_POINT('Ctrl Pts',(-64.4916766813467,60.4733826100211,-10.));
#36027=CARTESIAN_POINT('Ctrl Pts',(-64.5159179809605,60.3403227556477,-10.));
#36028=CARTESIAN_POINT('Ctrl Pts',(-64.5342155848992,60.2062848307327,-10.));
#36029=CARTESIAN_POINT('Ctrl Pts',(-64.5504250806423,60.0875432085724,-10.));
#36030=CARTESIAN_POINT('Ctrl Pts',(-64.5619694608586,59.9680332992326,-10.));
#36031=CARTESIAN_POINT('Ctrl Pts',(-64.568827180765,59.8480327443896,-10.));
#36032=CARTESIAN_POINT('Ctrl Pts',(-64.5705438281414,59.8179938042673,-10.));
#36033=CARTESIAN_POINT('Ctrl Pts',(-64.5719666480006,59.7879240952274,-10.));
#36034=CARTESIAN_POINT('Ctrl Pts',(-64.5730949929817,59.7578279370814,-10.));
#36035=CARTESIAN_POINT('Ctrl Pts',(-64.5739023538582,59.7362933346079,-10.));
#36036=CARTESIAN_POINT('Ctrl Pts',(-64.5745589112559,59.7147434601342,-10.));
#36037=CARTESIAN_POINT('Ctrl Pts',(-64.5750641121509,59.6932014838883,-10.));
#36038=CARTESIAN_POINT('Ctrl Pts',(-64.5783093817702,59.5548218377918,-10.));
#36039=CARTESIAN_POINT('Ctrl Pts',(-64.5753216210849,59.4165720657667,-10.));
#36040=CARTESIAN_POINT('Ctrl Pts',(-64.5661669353703,59.2788928886624,-10.));
#36041=CARTESIAN_POINT('Ctrl Pts',(-64.5569092713095,59.1396649993025,-10.));
#36042=CARTESIAN_POINT('Ctrl Pts',(-64.5413453776093,59.0010198399725,-10.));
#36043=CARTESIAN_POINT('Ctrl Pts',(-64.5194941179384,58.8633947014968,-10.));
#36044=CARTESIAN_POINT('Ctrl Pts',(-64.5146773775864,58.8330575690879,-10.));
#36045=CARTESIAN_POINT('Ctrl Pts',(-64.5095549335052,58.802769955891,-10.));
#36046=CARTESIAN_POINT('Ctrl Pts',(-64.5041266528052,58.7725364859968,-10.));
#36047=CARTESIAN_POINT('Ctrl Pts',(-64.4796517796898,58.6362207019781,-10.));
#36048=CARTESIAN_POINT('Ctrl Pts',(-64.4489637483093,58.5010054273352,-10.));
#36049=CARTESIAN_POINT('Ctrl Pts',(-64.4122746888345,58.3672428220256,-10.));
#36050=CARTESIAN_POINT('Ctrl Pts',(-64.3910362571152,58.2898108027772,-10.));
#36051=CARTESIAN_POINT('Ctrl Pts',(-64.3677859044126,58.2128655794348,-10.));
#36052=CARTESIAN_POINT('Ctrl Pts',(-64.3425569213142,58.1364765318665,-10.));
#36053=CARTESIAN_POINT('Ctrl Pts',(-64.3288268949054,58.094904359244,-10.));
#36054=CARTESIAN_POINT('Ctrl Pts',(-64.3145107565515,58.0534969305004,-10.));
#36055=CARTESIAN_POINT('Ctrl Pts',(-64.2996131836605,58.0122656222771,-10.));
#36056=CARTESIAN_POINT('Ctrl Pts',(-64.2935454822379,57.995472331894,-10.));
#36057=CARTESIAN_POINT('Ctrl Pts',(-64.2873813217626,57.9787082598248,-10.));
#36058=CARTESIAN_POINT('Ctrl Pts',(-64.281120995717,57.9619741830157,-10.));
#36059=CARTESIAN_POINT('Ctrl Pts',(-64.2745734675927,57.9444724047148,-10.));
#36060=CARTESIAN_POINT('Ctrl Pts',(-64.2679239845411,57.9270121153241,-10.));
#36061=CARTESIAN_POINT('Ctrl Pts',(-64.2611740923314,57.9095963866901,-10.));
#36062=CARTESIAN_POINT('Ctrl Pts',(-64.2098991560052,57.7772994034123,-10.));
#36063=CARTESIAN_POINT('Ctrl Pts',(-64.1528186249486,57.6475317114888,-10.));
#36064=CARTESIAN_POINT('Ctrl Pts',(-64.0902108000695,57.5206511899074,-10.));
#36065=CARTESIAN_POINT('Ctrl Pts',(-64.0269891381023,57.3925266709493,-10.));
#36066=CARTESIAN_POINT('Ctrl Pts',(-63.958131089877,57.2673454677456,-10.));
#36067=CARTESIAN_POINT('Ctrl Pts',(-63.8838698934635,57.1454790252293,-10.));
#36068=CARTESIAN_POINT('Ctrl Pts',(-63.8095390881361,57.0234983509056,-10.));
#36069=CARTESIAN_POINT('Ctrl Pts',(-63.7297947443748,56.9048378848756,-10.));
#36070=CARTESIAN_POINT('Ctrl Pts',(-63.644820966864,56.7898844568111,-10.));
#36071=CARTESIAN_POINT('Ctrl Pts',(-63.6122160516634,56.7457761814837,-10.));
#36072=CARTESIAN_POINT('Ctrl Pts',(-63.5788407066558,56.7022139043511,-10.));
#36073=CARTESIAN_POINT('Ctrl Pts',(-63.5447035113608,56.6592204097588,-10.));
#36074=CARTESIAN_POINT('Ctrl Pts',(-63.4815422486248,56.5796730601769,-10.));
#36075=CARTESIAN_POINT('Ctrl Pts',(-63.4157735403968,56.5020723187067,-10.));
#36076=CARTESIAN_POINT('Ctrl Pts',(-63.3475133873057,56.4265027019109,-10.));
#36077=CARTESIAN_POINT('Ctrl Pts',(-63.3334676224538,56.4109528822957,-10.));
#36078=CARTESIAN_POINT('Ctrl Pts',(-63.3193163336919,56.3954890903373,-10.));
#36079=CARTESIAN_POINT('Ctrl Pts',(-63.3050604789436,56.380112108533,-10.));
#36080=CARTESIAN_POINT('Ctrl Pts',(-63.2906483358829,56.3645665473919,-10.));
#36081=CARTESIAN_POINT('Ctrl Pts',(-63.2761359893981,56.3491169160922,-10.));
#36082=CARTESIAN_POINT('Ctrl Pts',(-63.2615262143732,56.3337653362877,-10.));
#36083=CARTESIAN_POINT('Ctrl Pts',(-63.1618951178549,56.2290755154917,-10.));
#36084=CARTESIAN_POINT('Ctrl Pts',(-63.0577151863935,56.1289202614804,-10.));
#36085=CARTESIAN_POINT('Ctrl Pts',(-62.9493854884616,56.0334960532877,-10.));
#36086=CARTESIAN_POINT('Ctrl Pts',(-62.8507323432671,55.9465956146673,-10.));
#36087=CARTESIAN_POINT('Ctrl Pts',(-62.7486367809699,55.8636187255677,-10.));
#36088=CARTESIAN_POINT('Ctrl Pts',(-62.6433691001371,55.7847332403089,-10.));
#36089=CARTESIAN_POINT('Ctrl Pts',(-62.587860446671,55.7431361705331,-10.));
#36090=CARTESIAN_POINT('Ctrl Pts',(-62.5314693058621,55.7026770787173,-10.));
#36091=CARTESIAN_POINT('Ctrl Pts',(-62.47423249159,55.6633831252636,-10.));
#36092=CARTESIAN_POINT('Ctrl Pts',(-62.4525293449788,55.6484835812623,-10.));
#36093=CARTESIAN_POINT('Ctrl Pts',(-62.4307045902376,55.633751578947,-10.));
#36094=CARTESIAN_POINT('Ctrl Pts',(-62.4087601696795,55.619188673283,-10.));
#36095=CARTESIAN_POINT('Ctrl Pts',(-62.3869959955472,55.6047453839783,-10.));
#36096=CARTESIAN_POINT('Ctrl Pts',(-62.3651201281095,55.5904724631012,-10.));
#36097=CARTESIAN_POINT('Ctrl Pts',(-62.3431409641125,55.5763751194668,-10.));
#36098=CARTESIAN_POINT('Ctrl Pts',(-62.2178093976035,55.4959879781926,-10.));
#36099=CARTESIAN_POINT('Ctrl Pts',(-62.0890600516578,55.4212658232662,-10.));
#36100=CARTESIAN_POINT('Ctrl Pts',(-61.9572867186068,55.3524361931912,-10.));
#36101=CARTESIAN_POINT('Ctrl Pts',(-61.8473201865616,55.2949969864408,-10.));
#36102=CARTESIAN_POINT('Ctrl Pts',(-61.7352467486275,55.2416617648057,-10.));
#36103=CARTESIAN_POINT('Ctrl Pts',(-61.6212758664505,55.1925826499274,-10.));
#36104=CARTESIAN_POINT('Ctrl Pts',(-61.5232159559749,55.1503552536024,-10.));
#36105=CARTESIAN_POINT('Ctrl Pts',(-61.4237510391233,55.1112787685727,-10.));
#36106=CARTESIAN_POINT('Ctrl Pts',(-61.3230392943658,55.0753649202911,-10.));
#36107=CARTESIAN_POINT('Ctrl Pts',(-55.7371269276513,60.000097806567,-7.57968167058905));
#36108=CARTESIAN_POINT('Ctrl Pts',(-55.7375456878641,59.5120606341344,-7.60701019445077));
#36109=CARTESIAN_POINT('Ctrl Pts',(-55.8213219729741,59.0238810226661,-7.63433871831249));
#36110=CARTESIAN_POINT('Ctrl Pts',(-55.9855957976042,58.5644884317184,-7.6616672421742));
#36111=CARTESIAN_POINT('Ctrl Pts',(-56.2198607163937,57.9093653879036,-7.70063945480463));
#36112=CARTESIAN_POINT('Ctrl Pts',(-56.6178300472846,57.312785279669,-7.73961166743506));
#36113=CARTESIAN_POINT('Ctrl Pts',(-57.1327248454888,56.844867445477,-7.77858388006549));
#36114=CARTESIAN_POINT('Ctrl Pts',(-57.6476196436931,56.376949611285,-7.81755609269592));
#36115=CARTESIAN_POINT('Ctrl Pts',(-58.2794399092106,56.0376940511356,-7.85652830532636));
#36116=CARTESIAN_POINT('Ctrl Pts',(-58.9539185995463,55.8669808559876,-7.89550051795679));
#36117=CARTESIAN_POINT('Ctrl Pts',(-59.6283972898821,55.6962676608397,-7.93447273058721));
#36118=CARTESIAN_POINT('Ctrl Pts',(-60.345534405036,55.6940968306933,-7.97344494321764));
#36119=CARTESIAN_POINT('Ctrl Pts',(-61.0210344788425,55.8607223865669,-8.01241715584807));
#36120=CARTESIAN_POINT('Ctrl Pts',(-61.6965345526489,56.0273479424406,-8.0513893684785));
#36121=CARTESIAN_POINT('Ctrl Pts',(-62.3303975851077,56.3627698843344,-8.09036158110893));
#36122=CARTESIAN_POINT('Ctrl Pts',(-62.8481164709991,56.8275617527175,-8.12933379373936));
#36123=CARTESIAN_POINT('Ctrl Pts',(-63.3658353568905,57.2923536211006,-8.16830600636979));
#36124=CARTESIAN_POINT('Ctrl Pts',(-63.7674100962144,57.8865154159731,-8.20727821900022));
#36125=CARTESIAN_POINT('Ctrl Pts',(-64.0056378088262,58.5402064583389,-8.24625043163065));
#36126=CARTESIAN_POINT('Ctrl Pts',(-64.2438655214379,59.1938975007047,-8.28522264426108));
#36127=CARTESIAN_POINT('Ctrl Pts',(-64.3187462073375,59.9071177905638,-8.32419485689151));
#36128=CARTESIAN_POINT('Ctrl Pts',(-64.2214780520756,60.596032352281,-8.36316706952194));
#36129=CARTESIAN_POINT('Ctrl Pts',(-64.1242098968137,61.2849469139981,-8.40213928215237));
#36130=CARTESIAN_POINT('Ctrl Pts',(-63.8547929003903,61.9495557475734,-8.4411114947828));
#36131=CARTESIAN_POINT('Ctrl Pts',(-63.4448955433497,62.5117376958675,-8.48008370741323));
#36132=CARTESIAN_POINT('Ctrl Pts',(-63.034998186309,63.0739196441617,-8.51905592004366));
#36133=CARTESIAN_POINT('Ctrl Pts',(-62.4846204686511,63.5336747071747,-8.55802813267409));
#36134=CARTESIAN_POINT('Ctrl Pts',(-61.8584562377277,63.8369612799398,-8.59700034530452));
#36135=CARTESIAN_POINT('Ctrl Pts',(-61.2322920068043,64.1402478527048,-8.63597255793495));
#36136=CARTESIAN_POINT('Ctrl Pts',(-60.5303412626156,64.2870659352219,-8.67494477056538));
#36137=CARTESIAN_POINT('Ctrl Pts',(-59.8351144418708,64.2601577920231,-8.71391698319581));
#36138=CARTESIAN_POINT('Ctrl Pts',(-59.1398876211261,64.2332496488243,-8.75288919582624));
#36139=CARTESIAN_POINT('Ctrl Pts',(-58.4513847238254,64.0326152799095,-8.79186140845667));
#36140=CARTESIAN_POINT('Ctrl Pts',(-57.8505354268778,63.6818383038823,-8.8308336210871));
#36141=CARTESIAN_POINT('Ctrl Pts',(-57.2496861299302,63.3310613278551,-8.86980583371753));
#36142=CARTESIAN_POINT('Ctrl Pts',(-56.7364904333356,62.8301417447155,-8.90877804634796));
#36143=CARTESIAN_POINT('Ctrl Pts',(-56.3712717081713,62.2379595431017,-8.94775025897839));
#36144=CARTESIAN_POINT('Ctrl Pts',(-56.0060529830071,61.6457773414879,-8.98672247160882));
#36145=CARTESIAN_POINT('Ctrl Pts',(-55.7888112292733,60.9623325214,-9.02569468423925));
#36146=CARTESIAN_POINT('Ctrl Pts',(-55.7450818863031,60.2679609567506,-9.06466689686968));
#36147=CARTESIAN_POINT('Ctrl Pts',(-55.7394660372551,60.1787877466035,-9.0696718214428));
#36148=CARTESIAN_POINT('Ctrl Pts',(-55.7367118314557,60.0894343277631,-9.07467674601593));
#36149=CARTESIAN_POINT('Ctrl Pts',(-55.7367869586782,60.0000762880139,-9.07968167058905));
#36150=CARTESIAN_POINT('Ctrl Pts',(-58.677115034431,55.0755938055567,-10.));
#36151=CARTESIAN_POINT('Ctrl Pts',(-57.8732233401272,55.2915500435982,-9.96102778736957));
#36152=CARTESIAN_POINT('Ctrl Pts',(-56.3739727673179,56.1245137043432,-9.88308336210872));
#36153=CARTESIAN_POINT('Ctrl Pts',(-54.9770227854932,58.2859118105468,-9.76616672421742));
#36154=CARTESIAN_POINT('Ctrl Pts',(-54.7611834123237,60.8500627421559,-9.64925008632613));
#36155=CARTESIAN_POINT('Ctrl Pts',(-55.7768178011049,63.214507276628,-9.53233344843484));
#36156=CARTESIAN_POINT('Ctrl Pts',(-57.7853302019076,64.8232034014141,-9.41541681054356));
#36157=CARTESIAN_POINT('Ctrl Pts',(-60.3144620657417,65.2980444973094,-9.29850017265226));
#36158=CARTESIAN_POINT('Ctrl Pts',(-62.769679003779,64.5273620844534,-9.18158353476097));
#36159=CARTESIAN_POINT('Ctrl Pts',(-64.5737697114167,62.6923525936502,-9.06466689686969));
#36160=CARTESIAN_POINT('Ctrl Pts',(-65.3026202914353,60.2243982367199,-8.94775025897839));
#36161=CARTESIAN_POINT('Ctrl Pts',(-64.7848823971216,57.703691543606,-8.83083362108711));
#36162=CARTESIAN_POINT('Ctrl Pts',(-63.1422721706319,55.7228209792253,-8.71391698319582));
#36163=CARTESIAN_POINT('Ctrl Pts',(-60.7609482860978,54.7474681235472,-8.59700034530452));
#36164=CARTESIAN_POINT('Ctrl Pts',(-58.2007340318709,55.0069271910455,-8.48008370741324));
#36165=CARTESIAN_POINT('Ctrl Pts',(-56.0635071617532,56.4402025452955,-8.36316706952194));
#36166=CARTESIAN_POINT('Ctrl Pts',(-54.8517063490748,58.7103466297086,-8.24625043163066));
#36167=CARTESIAN_POINT('Ctrl Pts',(-54.8502120322186,61.2836744106993,-8.12933379373937));
#36168=CARTESIAN_POINT('Ctrl Pts',(-56.059376560482,63.5552235595967,-8.01241715584808));
#36169=CARTESIAN_POINT('Ctrl Pts',(-58.1949364984747,64.9909811437472,-7.89550051795679));
#36170=CARTESIAN_POINT('Ctrl Pts',(-60.7548501786328,65.2534097268154,-7.7785838800655));
#36171=CARTESIAN_POINT('Ctrl Pts',(-63.1372998197884,64.2808297669235,-7.66166724217421));
#36172=CARTESIAN_POINT('Ctrl Pts',(-64.7822203790914,62.3018527171852,-7.54475060428292));
#36173=CARTESIAN_POINT('Ctrl Pts',(-65.3028606950879,59.7817818006449,-7.42783396639163));
#36174=CARTESIAN_POINT('Ctrl Pts',(-64.5769288017872,57.3129117888108,-7.31091732850034));
#36175=CARTESIAN_POINT('Ctrl Pts',(-62.7748569607921,55.4759618947992,-7.19400069060905));
#36176=CARTESIAN_POINT('Ctrl Pts',(-60.3207807277454,54.7020982939809,-7.07708405271776));
#36177=CARTESIAN_POINT('Ctrl Pts',(-57.7905713642451,55.1747170180384,-6.96016741482648));
#36178=CARTESIAN_POINT('Ctrl Pts',(-55.7813283808542,56.7795403162521,-6.84325077693518));
#36179=CARTESIAN_POINT('Ctrl Pts',(-54.7604821556384,59.1461432117513,-6.72633413904389));
#36180=CARTESIAN_POINT('Ctrl Pts',(-54.9785949323137,61.7034054152601,-6.60941750115261));
#36181=CARTESIAN_POINT('Ctrl Pts',(-56.822670191795,64.6083226141335,-6.45352865063088));
#36182=CARTESIAN_POINT('Ctrl Pts',(-61.3338600370175,65.8440763141619,-6.25866758747874));
#36183=CARTESIAN_POINT('Ctrl Pts',(-65.6028014358132,62.1309684734756,-6.02483431169615));
#36184=CARTESIAN_POINT('Ctrl Pts',(-65.0042200345167,57.4920438855145,-5.82997324854401));
#36185=CARTESIAN_POINT('Ctrl Pts',(-62.3829259668669,55.2631484402659,-5.67408439802228));
#36186=CARTESIAN_POINT('Ctrl Pts',(-59.8805750705293,54.692707249224,-5.557167760131));
#36187=CARTESIAN_POINT('Ctrl Pts',(-57.3953251078463,55.3756925371435,-5.44025112223971));
#36188=CARTESIAN_POINT('Ctrl Pts',(-55.5275118929263,57.1431169284426,-5.32333448434842));
#36189=CARTESIAN_POINT('Ctrl Pts',(-54.7087705821979,59.5834018600784,-5.20641784645713));
#36190=CARTESIAN_POINT('Ctrl Pts',(-55.1350332706562,62.1210494224441,-5.08950120856584));
#36191=CARTESIAN_POINT('Ctrl Pts',(-56.7044890264666,64.1603278398107,-4.97258457067455));
#36192=CARTESIAN_POINT('Ctrl Pts',(-59.0489177119773,65.2214359342736,-4.85566793278326));
#36193=CARTESIAN_POINT('Ctrl Pts',(-61.6168265705004,65.0550993586167,-4.73875129489197));
#36194=CARTESIAN_POINT('Ctrl Pts',(-63.8046877780167,63.7003384396424,-4.62183465700068));
#36195=CARTESIAN_POINT('Ctrl Pts',(-65.0980856806054,61.4756811768837,-4.50491801910939));
#36196=CARTESIAN_POINT('Ctrl Pts',(-65.1929908975039,58.9041019334819,-4.3880013812181));
#36197=CARTESIAN_POINT('Ctrl Pts',(-64.067076438205,56.5901588181647,-4.27108474332681));
#36198=CARTESIAN_POINT('Ctrl Pts',(-61.9850396737251,55.0778303984365,-4.15416810543552));
#36199=CARTESIAN_POINT('Ctrl Pts',(-59.4363409530604,54.7226501051879,-4.03725146754423));
#36200=CARTESIAN_POINT('Ctrl Pts',(-57.0201528028271,55.6081161060463,-3.92033482965294));
#36201=CARTESIAN_POINT('Ctrl Pts',(-55.3044933499955,57.526065446996,-3.80341819176166));
#36202=CARTESIAN_POINT('Ctrl Pts',(-54.6926959629807,60.0256094770039,-3.68650155387036));
#36203=CARTESIAN_POINT('Ctrl Pts',(-55.3285862201775,62.5191327628181,-3.56958491597908));
#36204=CARTESIAN_POINT('Ctrl Pts',(-57.0626757179785,64.4204363923688,-3.45266827808779));
#36205=CARTESIAN_POINT('Ctrl Pts',(-59.487294255791,65.282543142849,-3.3357516401965));
#36206=CARTESIAN_POINT('Ctrl Pts',(-62.0324515210899,64.9027851981381,-3.21883500230521));
#36207=CARTESIAN_POINT('Ctrl Pts',(-64.0997862762435,63.3704311081236,-3.10191836441392));
#36208=CARTESIAN_POINT('Ctrl Pts',(-65.2033407181402,61.045739110996,-2.98500172652263));
#36209=CARTESIAN_POINT('Ctrl Pts',(-65.083574915278,58.4751813271234,-2.86808508863134));
#36210=CARTESIAN_POINT('Ctrl Pts',(-63.7688780194889,56.2631621799769,-2.75116845074005));
#36211=CARTESIAN_POINT('Ctrl Pts',(-61.5678300058233,54.9295585406499,-2.63425181284876));
#36212=CARTESIAN_POINT('Ctrl Pts',(-59.8553056997907,54.8355306649757,-2.5563073875879));
#36213=CARTESIAN_POINT('Ctrl Pts',(-59.0378648750817,54.9925957821044,-2.51733517495747));
#36214=CARTESIAN_POINT('Ctrl Pts',(-58.7494123365958,55.344718704462,-10.1608882750142));
#36215=CARTESIAN_POINT('Ctrl Pts',(-57.9894543192508,55.5488726665669,-10.1219160623837));
#36216=CARTESIAN_POINT('Ctrl Pts',(-56.5721396475246,56.3363138313726,-10.0439716371229));
#36217=CARTESIAN_POINT('Ctrl Pts',(-55.2515347127552,58.3795888535214,-9.92705499923159));
#36218=CARTESIAN_POINT('Ctrl Pts',(-55.0474912287124,60.8036057602351,-9.81013836134031));
#36219=CARTESIAN_POINT('Ctrl Pts',(-56.0076199399737,63.0388304718126,-9.69322172344902));
#36220=CARTESIAN_POINT('Ctrl Pts',(-57.9063646499174,64.5596093605183,-9.57630508555773));
#36221=CARTESIAN_POINT('Ctrl Pts',(-60.2972763242917,65.0084998022875,-9.45938844766644));
#36222=CARTESIAN_POINT('Ctrl Pts',(-62.6183126151303,64.2799361380192,-9.34247180977515));
#36223=CARTESIAN_POINT('Ctrl Pts',(-64.323807530679,62.5452121891074,-9.22555517188386));
#36224=CARTESIAN_POINT('Ctrl Pts',(-65.0128255235959,60.2121345950975,-9.10863853399257));
#36225=CARTESIAN_POINT('Ctrl Pts',(-64.5233826465826,57.8291876454264,-8.99172189610128));
#36226=CARTESIAN_POINT('Ctrl Pts',(-62.9705431038444,55.9565741113013,-8.87480525820999));
#36227=CARTESIAN_POINT('Ctrl Pts',(-60.719361519596,55.0345254974581,-8.7578886203187));
#36228=CARTESIAN_POINT('Ctrl Pts',(-58.2990661459689,55.2798048054984,-8.64097198242741));
#36229=CARTESIAN_POINT('Ctrl Pts',(-56.2786413719103,56.63474988609,-8.52405534453612));
#36230=CARTESIAN_POINT('Ctrl Pts',(-55.1330669748298,58.7808277840241,-8.40713870664484));
#36231=CARTESIAN_POINT('Ctrl Pts',(-55.1316543242409,61.2135200139323,-8.29022206875354));
#36232=CARTESIAN_POINT('Ctrl Pts',(-56.2747365131157,63.360926187836,-8.17330543086225));
#36233=CARTESIAN_POINT('Ctrl Pts',(-58.2935854549548,64.7182178413891,-8.05638879297096));
#36234=CARTESIAN_POINT('Ctrl Pts',(-60.7135966812584,64.9663043772948,-7.93947215507967));
#36235=CARTESIAN_POINT('Ctrl Pts',(-62.9658424981343,64.0468771170479,-7.82255551718839));
#36236=CARTESIAN_POINT('Ctrl Pts',(-64.5208661111355,62.1760536146444,-7.70563887929709));
#36237=CARTESIAN_POINT('Ctrl Pts',(-65.013052788891,59.7937076955695,-7.58872224140581));
#36238=CARTESIAN_POINT('Ctrl Pts',(-64.3267939728473,57.4597644883305,-7.47180560351452));
#36239=CARTESIAN_POINT('Ctrl Pts',(-62.6232075903782,55.7232061816494,-7.35488896562323));
#36240=CARTESIAN_POINT('Ctrl Pts',(-60.3032496635893,54.9916351852819,-7.23797232773194));
#36241=CARTESIAN_POINT('Ctrl Pts',(-57.9113193762403,55.4384247105873,-7.12105568984065));
#36242=CARTESIAN_POINT('Ctrl Pts',(-56.011884010952,56.9555424274904,-7.00413905194936));
#36243=CARTESIAN_POINT('Ctrl Pts',(-55.0468282965736,59.1928075429912,-6.88722241405807));
#36244=CARTESIAN_POINT('Ctrl Pts',(-55.2530209398044,61.610312199129,-6.77030577616678));
#36245=CARTESIAN_POINT('Ctrl Pts',(-56.9963152019055,64.356472074458,-6.61441692564506));
#36246=CARTESIAN_POINT('Ctrl Pts',(-61.260962933602,65.5246903039221,-6.41955586249292));
#36247=CARTESIAN_POINT('Ctrl Pts',(-65.2966013965676,62.0145084065457,-6.18572258671033));
#36248=CARTESIAN_POINT('Ctrl Pts',(-64.7307332103775,57.6291067940397,-5.99086152355819));
#36249=CARTESIAN_POINT('Ctrl Pts',(-62.252696110797,55.5220232460408,-5.83497267303646));
#36250=CARTESIAN_POINT('Ctrl Pts',(-59.8871017908691,54.9827573727547,-5.71805603514517));
#36251=CARTESIAN_POINT('Ctrl Pts',(-57.5376738173867,55.6284166686038,-5.60113939725388));
#36252=CARTESIAN_POINT('Ctrl Pts',(-55.7719389085185,57.2992491274242,-5.48422275936259));
#36253=CARTESIAN_POINT('Ctrl Pts',(-54.9979428246821,59.606169464509,-5.36730612147131));
#36254=CARTESIAN_POINT('Ctrl Pts',(-55.40090972916,62.0051314439409,-5.25038948358002));
#36255=CARTESIAN_POINT('Ctrl Pts',(-56.8845927836657,63.9329607695301,-5.13347284568873));
#36256=CARTESIAN_POINT('Ctrl Pts',(-59.1008955372232,64.9360779921247,-5.01655620779744));
#36257=CARTESIAN_POINT('Ctrl Pts',(-61.5284649954897,64.7788319163859,-4.89963956990615));
#36258=CARTESIAN_POINT('Ctrl Pts',(-63.5967568776818,63.4981103599182,-4.78272293201486));
#36259=CARTESIAN_POINT('Ctrl Pts',(-64.8194689826264,61.3950333724858,-4.66580629412357));
#36260=CARTESIAN_POINT('Ctrl Pts',(-64.9091875118522,58.9639941204211,-4.54888965623228));
#36261=CARTESIAN_POINT('Ctrl Pts',(-63.8448056725426,56.7765108628803,-4.43197301834099));
#36262=CARTESIAN_POINT('Ctrl Pts',(-61.8765547964789,55.3468330647702,-4.3150563804497));
#36263=CARTESIAN_POINT('Ctrl Pts',(-59.4671456182393,55.0110638145468,-4.19813974255841));
#36264=CARTESIAN_POINT('Ctrl Pts',(-57.1830051436022,55.8481380015386,-4.08122310466712));
#36265=CARTESIAN_POINT('Ctrl Pts',(-55.5611086052354,57.6612690350401,-3.96430646677583));
#36266=CARTESIAN_POINT('Ctrl Pts',(-54.9827467033185,60.0242098873605,-3.84738982888454));
#36267=CARTESIAN_POINT('Ctrl Pts',(-55.5838847702156,62.3814590366158,-3.73047319099325));
#36268=CARTESIAN_POINT('Ctrl Pts',(-57.2232041287629,64.1788540674672,-3.61355655310196));
#36269=CARTESIAN_POINT('Ctrl Pts',(-59.5153142598545,64.9938456160515,-3.49663991521067));
#36270=CARTESIAN_POINT('Ctrl Pts',(-61.9213755276512,64.634841913465,-3.37972327731938));
#36271=CARTESIAN_POINT('Ctrl Pts',(-63.8757278774111,63.1862328727577,-3.26280663942809));
#36272=CARTESIAN_POINT('Ctrl Pts',(-64.9189717019694,60.9885881731132,-3.1458900015368));
#36273=CARTESIAN_POINT('Ctrl Pts',(-64.8057512486,58.5585145565491,-3.02897336364551));
#36274=CARTESIAN_POINT('Ctrl Pts',(-63.5629041668189,56.4673849960545,-2.91205672575423));
#36275=CARTESIAN_POINT('Ctrl Pts',(-61.4821461537694,55.2066644476915,-2.79514008786293));
#36276=CARTESIAN_POINT('Ctrl Pts',(-59.8632134225452,55.1177753119051,-2.71719566260207));
#36277=CARTESIAN_POINT('Ctrl Pts',(-59.0904467515563,55.2662566258098,-2.67822344997165));
#36278=CARTESIAN_POINT('Ctrl Pts',(-58.8217096387607,55.6138436033673,-10.3217765500284));
#36279=CARTESIAN_POINT('Ctrl Pts',(-58.1056852983744,55.8061952895356,-10.2828043373979));
#36280=CARTESIAN_POINT('Ctrl Pts',(-56.7703065277313,56.548113958402,-10.2048599121371));
#36281=CARTESIAN_POINT('Ctrl Pts',(-55.5260466400173,58.473265896496,-10.0879432742458));
#36282=CARTESIAN_POINT('Ctrl Pts',(-55.333799045101,60.7571487783143,-9.97102663635449));
#36283=CARTESIAN_POINT('Ctrl Pts',(-56.2384220788426,62.8631536669972,-9.85410999846319));
#36284=CARTESIAN_POINT('Ctrl Pts',(-58.0273990979271,64.2960153196226,-9.73719336057191));
#36285=CARTESIAN_POINT('Ctrl Pts',(-60.2800905828417,64.7189551072656,-9.62027672268061));
#36286=CARTESIAN_POINT('Ctrl Pts',(-62.4669462264816,64.0325101915851,-9.50336008478932));
#36287=CARTESIAN_POINT('Ctrl Pts',(-64.0738453499413,62.3980717845645,-9.38644344689804));
#36288=CARTESIAN_POINT('Ctrl Pts',(-64.7230307557564,60.1998709534751,-9.26952680900674));
#36289=CARTESIAN_POINT('Ctrl Pts',(-64.2618828960438,57.9546837472467,-9.15261017111546));
#36290=CARTESIAN_POINT('Ctrl Pts',(-62.7988140370569,56.1903272433774,-9.03569353322417));
#36291=CARTESIAN_POINT('Ctrl Pts',(-60.6777747530942,55.321582871369,-8.91877689533288));
#36292=CARTESIAN_POINT('Ctrl Pts',(-58.3973982600668,55.5526824199513,-8.80186025744159));
#36293=CARTESIAN_POINT('Ctrl Pts',(-56.4937755820675,56.8292972268845,-8.6849436195503));
#36294=CARTESIAN_POINT('Ctrl Pts',(-55.4144276005848,58.8513089383396,-8.56802698165902));
#36295=CARTESIAN_POINT('Ctrl Pts',(-55.4130966162632,61.1433656171654,-8.45111034376772));
#36296=CARTESIAN_POINT('Ctrl Pts',(-56.4900964657494,63.1666288160754,-8.33419370587643));
#36297=CARTESIAN_POINT('Ctrl Pts',(-58.3922344114348,64.4454545390309,-8.21727706798514));
#36298=CARTESIAN_POINT('Ctrl Pts',(-60.6723431838839,64.6791990277741,-8.10036043009385));
#36299=CARTESIAN_POINT('Ctrl Pts',(-62.7943851764801,63.8129244671722,-7.98344379220257));
#36300=CARTESIAN_POINT('Ctrl Pts',(-64.2595118431797,62.0502545121036,-7.86652715431127));
#36301=CARTESIAN_POINT('Ctrl Pts',(-64.7232448826942,59.805633590494,-7.74961051641999));
#36302=CARTESIAN_POINT('Ctrl Pts',(-64.0766591439074,57.6066171878503,-7.63269387852869));
#36303=CARTESIAN_POINT('Ctrl Pts',(-62.4715582199642,55.9704504684996,-7.5157772406374));
#36304=CARTESIAN_POINT('Ctrl Pts',(-60.2857185994333,55.2811720765829,-7.39886060274612));
#36305=CARTESIAN_POINT('Ctrl Pts',(-58.0320673882356,55.7021324031362,-7.28194396485482));
#36306=CARTESIAN_POINT('Ctrl Pts',(-56.2424396410498,57.1315445387288,-7.16502732696353));
#36307=CARTESIAN_POINT('Ctrl Pts',(-55.3331744375089,59.239471874231,-7.04811068907225));
#36308=CARTESIAN_POINT('Ctrl Pts',(-55.5274469472951,61.5172189829979,-6.93119405118096));
#36309=CARTESIAN_POINT('Ctrl Pts',(-57.1699602120159,64.1046215347825,-6.77530520065924));
#36310=CARTESIAN_POINT('Ctrl Pts',(-61.1880658301865,65.2053042936822,-6.58044413750709));
#36311=CARTESIAN_POINT('Ctrl Pts',(-64.9904013573221,61.8980483396159,-6.34661086172452));
#36312=CARTESIAN_POINT('Ctrl Pts',(-64.4572463862384,57.7661697025649,-6.15174979857236));
#36313=CARTESIAN_POINT('Ctrl Pts',(-62.1224662547272,55.7808980518156,-5.99586094805064));
#36314=CARTESIAN_POINT('Ctrl Pts',(-59.8936285112088,55.2728074962854,-5.87894431015935));
#36315=CARTESIAN_POINT('Ctrl Pts',(-57.6800225269272,55.8811408000641,-5.76202767226806));
#36316=CARTESIAN_POINT('Ctrl Pts',(-56.0163659241107,57.4553813264059,-5.64511103437677));
#36317=CARTESIAN_POINT('Ctrl Pts',(-55.2871150671665,59.6289370689395,-5.52819439648548));
#36318=CARTESIAN_POINT('Ctrl Pts',(-55.6667861876637,61.8892134654378,-5.41127775859419));
#36319=CARTESIAN_POINT('Ctrl Pts',(-57.0646965408647,63.7055936992496,-5.2943611207029));
#36320=CARTESIAN_POINT('Ctrl Pts',(-59.1528733624691,64.6507200499757,-5.17744448281161));
#36321=CARTESIAN_POINT('Ctrl Pts',(-61.440103420479,64.5025644741552,-5.06052784492032));
#36322=CARTESIAN_POINT('Ctrl Pts',(-63.388825977347,63.295882280194,-4.94361120702904));
#36323=CARTESIAN_POINT('Ctrl Pts',(-64.5408522846473,61.3143855680879,-4.82669456913774));
#36324=CARTESIAN_POINT('Ctrl Pts',(-64.6253841262005,59.0238863073603,-4.70977793124646));
#36325=CARTESIAN_POINT('Ctrl Pts',(-63.6225349068801,56.9628629075959,-4.59286129335516));
#36326=CARTESIAN_POINT('Ctrl Pts',(-61.7680699192328,55.615835731104,-4.47594465546388));
#36327=CARTESIAN_POINT('Ctrl Pts',(-59.4979502834182,55.2994775239056,-4.35902801757258));
#36328=CARTESIAN_POINT('Ctrl Pts',(-57.3458574843773,56.0881598970308,-4.2421113796813));
#36329=CARTESIAN_POINT('Ctrl Pts',(-55.8177238604752,57.7964726230843,-4.12519474179001));
#36330=CARTESIAN_POINT('Ctrl Pts',(-55.2727974436564,60.0228102977171,-4.00827810389872));
#36331=CARTESIAN_POINT('Ctrl Pts',(-55.8391833202536,62.2437853104136,-3.89136146600743));
#36332=CARTESIAN_POINT('Ctrl Pts',(-57.3837325395474,63.9372717425656,-3.77444482811614));
#36333=CARTESIAN_POINT('Ctrl Pts',(-59.543334263918,64.7051480892539,-3.65752819022485));
#36334=CARTESIAN_POINT('Ctrl Pts',(-61.8102995342126,64.366898628792,-3.54061155233356));
#36335=CARTESIAN_POINT('Ctrl Pts',(-63.6516694785787,63.0020346373919,-3.42369491444227));
#36336=CARTESIAN_POINT('Ctrl Pts',(-64.6346026857985,60.9314372352304,-3.30677827655098));
#36337=CARTESIAN_POINT('Ctrl Pts',(-64.5279275819221,58.6418477859748,-3.18986163865969));
#36338=CARTESIAN_POINT('Ctrl Pts',(-63.3569303141489,56.6716078121321,-3.0729450007684));
#36339=CARTESIAN_POINT('Ctrl Pts',(-61.3964623017155,55.4837703547332,-2.95602836287711));
#36340=CARTESIAN_POINT('Ctrl Pts',(-59.8711211452996,55.4000199588346,-2.87808393761625));
#36341=CARTESIAN_POINT('Ctrl Pts',(-59.1430286280309,55.5399174695151,-2.83911172498582));
#36342=CARTESIAN_POINT('Ctrl Pts',(-58.8940069409255,55.8829685022727,-10.4826648250425));
#36343=CARTESIAN_POINT('Ctrl Pts',(-58.221916277498,56.0635179125043,-10.4436926124121));
#36344=CARTESIAN_POINT('Ctrl Pts',(-56.9684734079381,56.7599140854314,-10.3657481871512));
#36345=CARTESIAN_POINT('Ctrl Pts',(-55.8005585672793,58.5669429394706,-10.2488315492599));
#36346=CARTESIAN_POINT('Ctrl Pts',(-55.6201068614897,60.7106917963935,-10.1319149113687));
#36347=CARTESIAN_POINT('Ctrl Pts',(-56.4692242177114,62.6874768621819,-10.0149982734774));
#36348=CARTESIAN_POINT('Ctrl Pts',(-58.1484335459369,64.0324212787269,-9.89808163558609));
#36349=CARTESIAN_POINT('Ctrl Pts',(-60.2629048413918,64.4294104122436,-9.78116499769479));
#36350=CARTESIAN_POINT('Ctrl Pts',(-62.3155798378329,63.785084245151,-9.6642483598035));
#36351=CARTESIAN_POINT('Ctrl Pts',(-63.8238831692036,62.2509313800217,-9.54733172191221));
#36352=CARTESIAN_POINT('Ctrl Pts',(-64.433235987917,60.1876073118527,-9.43041508402092));
#36353=CARTESIAN_POINT('Ctrl Pts',(-64.0003831455049,58.080179849067,-9.31349844612964));
#36354=CARTESIAN_POINT('Ctrl Pts',(-62.6270849702694,56.4240803754535,-9.19658180823835));
#36355=CARTESIAN_POINT('Ctrl Pts',(-60.6361879865924,55.6086402452798,-9.07966517034705));
#36356=CARTESIAN_POINT('Ctrl Pts',(-58.4957303741647,55.8255600344042,-8.96274853245577));
#36357=CARTESIAN_POINT('Ctrl Pts',(-56.7089097922247,57.0238445676789,-8.84583189456447));
#36358=CARTESIAN_POINT('Ctrl Pts',(-55.6957882263397,58.921790092655,-8.72891525667319));
#36359=CARTESIAN_POINT('Ctrl Pts',(-55.6945389082855,61.0732112203983,-8.6119986187819));
#36360=CARTESIAN_POINT('Ctrl Pts',(-56.705456418383,62.9723314443147,-8.49508198089061));
#36361=CARTESIAN_POINT('Ctrl Pts',(-58.4908833679148,64.1726912366728,-8.37816534299932));
#36362=CARTESIAN_POINT('Ctrl Pts',(-60.6310896865095,64.3920936782534,-8.26124870510802));
#36363=CARTESIAN_POINT('Ctrl Pts',(-62.622927854826,63.5789718172965,-8.14433206721674));
#36364=CARTESIAN_POINT('Ctrl Pts',(-63.9981575752239,61.9244554095628,-8.02741542932544));
#36365=CARTESIAN_POINT('Ctrl Pts',(-64.4334369764973,59.8175594854186,-7.91049879143416));
#36366=CARTESIAN_POINT('Ctrl Pts',(-63.8265243149675,57.7534698873702,-7.79358215354287));
#36367=CARTESIAN_POINT('Ctrl Pts',(-62.3199088495502,56.2176947553498,-7.67666551565158));
#36368=CARTESIAN_POINT('Ctrl Pts',(-60.2681875352772,55.570708967884,-7.55974887776029));
#36369=CARTESIAN_POINT('Ctrl Pts',(-58.1528154002308,55.965840095685,-7.442832239869));
#36370=CARTESIAN_POINT('Ctrl Pts',(-56.4729952711476,57.3075466499671,-7.32591560197771));
#36371=CARTESIAN_POINT('Ctrl Pts',(-55.6195205784441,59.2861362054709,-7.20899896408642));
#36372=CARTESIAN_POINT('Ctrl Pts',(-55.8018729547859,61.4241257668668,-7.09208232619513));
#36373=CARTESIAN_POINT('Ctrl Pts',(-57.3436052221264,63.8527709951071,-6.93619347567341));
#36374=CARTESIAN_POINT('Ctrl Pts',(-61.115168726771,64.8859182834423,-6.74133241252127));
#36375=CARTESIAN_POINT('Ctrl Pts',(-64.6842013180765,61.7815882726861,-6.50749913673869));
#36376=CARTESIAN_POINT('Ctrl Pts',(-64.1837595620993,57.9032326110901,-6.31263807358654));
#36377=CARTESIAN_POINT('Ctrl Pts',(-61.9922363986573,56.0397728575904,-6.15674922306481));
#36378=CARTESIAN_POINT('Ctrl Pts',(-59.9001552315486,55.562857619816,-6.03983258517353));
#36379=CARTESIAN_POINT('Ctrl Pts',(-57.8223712364677,56.1338649315244,-5.92291594728224));
#36380=CARTESIAN_POINT('Ctrl Pts',(-56.2607929397029,57.6115135253875,-5.80599930939094));
#36381=CARTESIAN_POINT('Ctrl Pts',(-55.5762873096508,59.6517046733701,-5.68908267149966));
#36382=CARTESIAN_POINT('Ctrl Pts',(-55.9326626461674,61.7732954869346,-5.57216603360837));
#36383=CARTESIAN_POINT('Ctrl Pts',(-57.2448002980638,63.4782266289691,-5.45524939571708));
#36384=CARTESIAN_POINT('Ctrl Pts',(-59.2048511877151,64.3653621078267,-5.33833275782579));
#36385=CARTESIAN_POINT('Ctrl Pts',(-61.3517418454684,64.2262970319245,-5.2214161199345));
#36386=CARTESIAN_POINT('Ctrl Pts',(-63.1808950770122,63.0936542004698,-5.10449948204321));
#36387=CARTESIAN_POINT('Ctrl Pts',(-64.2622355866681,61.23373776369,-4.98758284415192));
#36388=CARTESIAN_POINT('Ctrl Pts',(-64.341580740549,59.0837784942996,-4.87066620626063));
#36389=CARTESIAN_POINT('Ctrl Pts',(-63.4002641412175,57.1492149523114,-4.75374956836934));
#36390=CARTESIAN_POINT('Ctrl Pts',(-61.6595850419867,55.8848383974377,-4.63683293047805));
#36391=CARTESIAN_POINT('Ctrl Pts',(-59.5287549485971,55.5878912332645,-4.51991629258676));
#36392=CARTESIAN_POINT('Ctrl Pts',(-57.5087098251523,56.3281817925231,-4.40299965469547));
#36393=CARTESIAN_POINT('Ctrl Pts',(-56.074339115715,57.9316762111284,-4.28608301680419));
#36394=CARTESIAN_POINT('Ctrl Pts',(-55.5628481839942,60.0214107080737,-4.16916637891289));
#36395=CARTESIAN_POINT('Ctrl Pts',(-56.0944818702916,62.1061115842113,-4.05224974102161));
#36396=CARTESIAN_POINT('Ctrl Pts',(-57.5442609503319,63.6956894176639,-3.93533310313031));
#36397=CARTESIAN_POINT('Ctrl Pts',(-59.5713542679814,64.4164505624564,-3.81841646523903));
#36398=CARTESIAN_POINT('Ctrl Pts',(-61.6992235407739,64.0989553441189,-3.70149982734774));
#36399=CARTESIAN_POINT('Ctrl Pts',(-63.4276110797463,62.817836402026,-3.58458318945645));
#36400=CARTESIAN_POINT('Ctrl Pts',(-64.3502336696277,60.8742862973476,-3.46766655156516));
#36401=CARTESIAN_POINT('Ctrl Pts',(-64.2501039152442,58.7251810154005,-3.35074991367387));
#36402=CARTESIAN_POINT('Ctrl Pts',(-63.150956461479,56.8758306282097,-3.23383327578258));
#36403=CARTESIAN_POINT('Ctrl Pts',(-61.3107784496616,55.7608762617749,-3.11691663789129));
#36404=CARTESIAN_POINT('Ctrl Pts',(-59.8790288680541,55.6822646057641,-3.03897221263043));
#36405=CARTESIAN_POINT('Ctrl Pts',(-59.1956105045055,55.8135783132205,-3.));
#36406=CARTESIAN_POINT('Ctrl Pts',(-55.7373303217998,60.0000007547395,-8.67031832941094));
#36407=CARTESIAN_POINT('Ctrl Pts',(-55.7373282077215,60.3472087804744,-8.65087842586793));
#36408=CARTESIAN_POINT('Ctrl Pts',(-55.7792938624899,60.6944162976158,-8.63143852232491));
#36409=CARTESIAN_POINT('Ctrl Pts',(-55.8632333796441,61.0311610697605,-8.6119986187819));
#36410=CARTESIAN_POINT('Ctrl Pts',(-56.0315114116513,61.7062512950371,-8.57302640615147));
#36411=CARTESIAN_POINT('Ctrl Pts',(-56.3684839150172,62.3392913696759,-8.53405419352104));
#36412=CARTESIAN_POINT('Ctrl Pts',(-56.8345413249554,62.8558713723883,-8.49508198089061));
#36413=CARTESIAN_POINT('Ctrl Pts',(-57.3005987348936,63.3724513751007,-8.45610976826018));
#36414=CARTESIAN_POINT('Ctrl Pts',(-57.8957410514042,63.7725713058868,-8.41713755562975));
#36415=CARTESIAN_POINT('Ctrl Pts',(-58.5500132627586,64.0091983448765,-8.37816534299932));
#36416=CARTESIAN_POINT('Ctrl Pts',(-59.204285474113,64.2458253838663,-8.33919313036889));
#36417=CARTESIAN_POINT('Ctrl Pts',(-59.9176875803113,64.3189595310599,-8.30022091773846));
#36418=CARTESIAN_POINT('Ctrl Pts',(-60.6063616614631,64.2200062944972,-8.26124870510803));
#36419=CARTESIAN_POINT('Ctrl Pts',(-61.295035742615,64.1210530579345,-8.2222764924776));
#36420=CARTESIAN_POINT('Ctrl Pts',(-61.9589817987205,63.8500124376155,-8.18330427984717));
#36421=CARTESIAN_POINT('Ctrl Pts',(-62.5201597801729,63.4387393928337,-8.14433206721674));
#36422=CARTESIAN_POINT('Ctrl Pts',(-63.0813377616253,63.027466348052,-8.10535985458631));
#36423=CARTESIAN_POINT('Ctrl Pts',(-63.5397476684246,62.4759608788074,-8.06638764195588));
#36424=CARTESIAN_POINT('Ctrl Pts',(-63.8414991887032,61.8490588234943,-8.02741542932545));
#36425=CARTESIAN_POINT('Ctrl Pts',(-64.1432507089817,61.2221567681814,-7.98844321669502));
#36426=CARTESIAN_POINT('Ctrl Pts',(-64.2883438427395,60.5198581268,-7.94947100406459));
#36427=CARTESIAN_POINT('Ctrl Pts',(-64.2597382993634,59.8246938731012,-7.91049879143416));
#36428=CARTESIAN_POINT('Ctrl Pts',(-64.2311327559874,59.1295296194024,-7.87152657880373));
#36429=CARTESIAN_POINT('Ctrl Pts',(-64.0288285354774,58.4414997533863,-7.8325543661733));
#36430=CARTESIAN_POINT('Ctrl Pts',(-63.6765738476529,57.8415222983748,-7.79358215354287));
#36431=CARTESIAN_POINT('Ctrl Pts',(-63.3243191598284,57.2415448433634,-7.75460994091244));
#36432=CARTESIAN_POINT('Ctrl Pts',(-62.8221140046893,56.7296197993566,-7.71563772828201));
#36433=CARTESIAN_POINT('Ctrl Pts',(-62.229057874741,56.3658263127756,-7.67666551565158));
#36434=CARTESIAN_POINT('Ctrl Pts',(-61.6360017447926,56.0020328261945,-7.63769330302115));
#36435=CARTESIAN_POINT('Ctrl Pts',(-60.9520946400349,55.7863708970392,-7.59872109039072));
#36436=CARTESIAN_POINT('Ctrl Pts',(-60.2575790651483,55.7443951204284,-7.55974887776029));
#36437=CARTESIAN_POINT('Ctrl Pts',(-59.5630634902618,55.7024193438176,-7.52077666512986));
#36438=CARTESIAN_POINT('Ctrl Pts',(-58.8579394452463,55.8341297197513,-7.48180445249943));
#36439=CARTESIAN_POINT('Ctrl Pts',(-58.2254074012247,56.1236026667652,-7.442832239869));
#36440=CARTESIAN_POINT('Ctrl Pts',(-57.5928753572031,56.4130756137791,-7.40386002723857));
#36441=CARTESIAN_POINT('Ctrl Pts',(-57.0329353141753,56.8603111318731,-7.36488781460814));
#36442=CARTESIAN_POINT('Ctrl Pts',(-56.6107195105442,57.4136938168374,-7.32591560197771));
#36443=CARTESIAN_POINT('Ctrl Pts',(-56.1885037069131,57.9670765018017,-7.28694338934728));
#36444=CARTESIAN_POINT('Ctrl Pts',(-55.9040121426786,58.6266063536363,-7.24797117671685));
#36445=CARTESIAN_POINT('Ctrl Pts',(-55.792158423285,59.3127028731196,-7.20899896408642));
#36446=CARTESIAN_POINT('Ctrl Pts',(-55.7551528017157,59.5396906594681,-7.1961054191946));
#36447=CARTESIAN_POINT('Ctrl Pts',(-55.7370432093912,59.7695862933357,-7.18321187430277));
#36448=CARTESIAN_POINT('Ctrl Pts',(-55.7374561790016,59.9995175300878,-7.17031832941094));
#36449=CARTESIAN_POINT('Ctrl Pts',(-58.677115034431,55.0755938055567,-10.));
#36450=CARTESIAN_POINT('Ctrl Pts',(-58.5386376224601,55.1251023467987,-10.));
#36451=CARTESIAN_POINT('Ctrl Pts',(-58.4026668815791,55.1806178076285,-10.));
#36452=CARTESIAN_POINT('Ctrl Pts',(-58.2695272544167,55.2418650197503,-10.));
#36453=CARTESIAN_POINT('Ctrl Pts',(-58.135336471899,55.3035957868918,-10.));
#36454=CARTESIAN_POINT('Ctrl Pts',(-58.0040210293143,55.371149627725,-10.));
#36455=CARTESIAN_POINT('Ctrl Pts',(-57.8759387502434,55.4442909167463,-10.));
#36456=CARTESIAN_POINT('Ctrl Pts',(-57.7488534505964,55.5168628814183,-10.));
#36457=CARTESIAN_POINT('Ctrl Pts',(-57.6249506202847,55.5949361888115,-10.));
#36458=CARTESIAN_POINT('Ctrl Pts',(-57.5046138796569,55.6783182407818,-10.));
#36459=CARTESIAN_POINT('Ctrl Pts',(-57.3858527971248,55.7606085097726,-10.));
#36460=CARTESIAN_POINT('Ctrl Pts',(-57.2705645546623,55.8480699257949,-10.));
#36461=CARTESIAN_POINT('Ctrl Pts',(-57.1591587964671,55.9405462498422,-10.));
#36462=CARTESIAN_POINT('Ctrl Pts',(-57.1274511406442,55.9668663207448,-10.));
#36463=CARTESIAN_POINT('Ctrl Pts',(-57.0960582671108,55.9935927805097,-10.));
#36464=CARTESIAN_POINT('Ctrl Pts',(-57.0649903190273,56.020722374975,-10.));
#36465=CARTESIAN_POINT('Ctrl Pts',(-57.0492520137067,56.0344656012663,-10.));
#36466=CARTESIAN_POINT('Ctrl Pts',(-57.0335970960159,56.048312282282,-10.));
#36467=CARTESIAN_POINT('Ctrl Pts',(-57.018026917309,56.0622620081661,-10.));
#36468=CARTESIAN_POINT('Ctrl Pts',(-57.0026738875857,56.0760171846584,-10.));
#36469=CARTESIAN_POINT('Ctrl Pts',(-56.9874092917288,56.0898671766707,-10.));
#36470=CARTESIAN_POINT('Ctrl Pts',(-56.9722391118383,56.1038067825593,-10.));
#36471=CARTESIAN_POINT('Ctrl Pts',(-56.8611663613498,56.2058695384362,-10.));
#36472=CARTESIAN_POINT('Ctrl Pts',(-56.7550660406813,56.3128091758504,-10.));
#36473=CARTESIAN_POINT('Ctrl Pts',(-56.6543282067119,56.4243834820602,-10.));
#36474=CARTESIAN_POINT('Ctrl Pts',(-56.5578656854931,56.5312225757368,-10.));
#36475=CARTESIAN_POINT('Ctrl Pts',(-56.4663200079077,56.6423122346398,-10.));
#36476=CARTESIAN_POINT('Ctrl Pts',(-56.3798948625733,56.757269687502,-10.));
#36477=CARTESIAN_POINT('Ctrl Pts',(-56.2936201130584,56.8720270930254,-10.));
#36478=CARTESIAN_POINT('Ctrl Pts',(-56.2124477882373,56.9906396027887,-10.));
#36479=CARTESIAN_POINT('Ctrl Pts',(-56.1366282844148,57.1127461598228,-10.));
#36480=CARTESIAN_POINT('Ctrl Pts',(-56.0709511389806,57.2185185495178,-10.));
#36481=CARTESIAN_POINT('Ctrl Pts',(-56.0092911309896,57.3269133050067,-10.));
#36482=CARTESIAN_POINT('Ctrl Pts',(-55.9518427208356,57.4377011839666,-10.));
#36483=CARTESIAN_POINT('Ctrl Pts',(-55.9367455036519,57.4668158046411,-10.));
#36484=CARTESIAN_POINT('Ctrl Pts',(-55.9219393122137,57.4960957081207,-10.));
#36485=CARTESIAN_POINT('Ctrl Pts',(-55.9074280351729,57.525536740701,-10.));
#36486=CARTESIAN_POINT('Ctrl Pts',(-55.8951622011407,57.5504221328239,-10.));
#36487=CARTESIAN_POINT('Ctrl Pts',(-55.8831044077694,57.5754285256612,-10.));
#36488=CARTESIAN_POINT('Ctrl Pts',(-55.8712719981158,57.6005211318673,-10.));
#36489=CARTESIAN_POINT('Ctrl Pts',(-55.8112491801806,57.727809569127,-10.));
#36490=CARTESIAN_POINT('Ctrl Pts',(-55.7569584161731,57.8574378456489,-10.));
#36491=CARTESIAN_POINT('Ctrl Pts',(-55.708587679128,57.9890469247172,-10.));
#36492=CARTESIAN_POINT('Ctrl Pts',(-55.660604700135,58.1196009758233,-10.));
#36493=CARTESIAN_POINT('Ctrl Pts',(-55.6184470131256,58.2521049312923,-10.));
#36494=CARTESIAN_POINT('Ctrl Pts',(-55.5823476675558,58.3862204353038,-10.));
#36495=CARTESIAN_POINT('Ctrl Pts',(-55.5736126976742,58.4186724055459,-10.));
#36496=CARTESIAN_POINT('Ctrl Pts',(-55.5652326786128,58.451218759105,-10.));
#36497=CARTESIAN_POINT('Ctrl Pts',(-55.5572113733907,58.4838547369515,-10.));
#36498=CARTESIAN_POINT('Ctrl Pts',(-55.5237968418714,58.6198071636733,-10.));
#36499=CARTESIAN_POINT('Ctrl Pts',(-55.4966031500819,58.7573154760479,-10.));
#36500=CARTESIAN_POINT('Ctrl Pts',(-55.4756766726658,58.8959462545501,-10.));
#36501=CARTESIAN_POINT('Ctrl Pts',(-55.4642433082102,58.9716883961376,-10.));
#36502=CARTESIAN_POINT('Ctrl Pts',(-55.4546816532845,59.0477654877749,-10.));
#36503=CARTESIAN_POINT('Ctrl Pts',(-55.4470056777547,59.124105191105,-10.));
#36504=CARTESIAN_POINT('Ctrl Pts',(-55.4421350689108,59.1725447454963,-10.));
#36505=CARTESIAN_POINT('Ctrl Pts',(-55.4380237695898,59.2210900052751,-10.));
#36506=CARTESIAN_POINT('Ctrl Pts',(-55.4346762817703,59.269722103547,-10.));
#36507=CARTESIAN_POINT('Ctrl Pts',(-55.4333863538523,59.2884620974328,-10.));
#36508=CARTESIAN_POINT('Ctrl Pts',(-55.4322097104365,59.3072175092192,-10.));
#36509=CARTESIAN_POINT('Ctrl Pts',(-55.4311470975273,59.3259789773854,-10.));
#36510=CARTESIAN_POINT('Ctrl Pts',(-55.4233879220381,59.4629747946461,-10.));
#36511=CARTESIAN_POINT('Ctrl Pts',(-55.4217193407444,59.5999983377396,-10.));
#36512=CARTESIAN_POINT('Ctrl Pts',(-55.4261204589518,59.7366439247398,-10.));
#36513=CARTESIAN_POINT('Ctrl Pts',(-55.4305091604386,59.8729039983356,-10.));
#36514=CARTESIAN_POINT('Ctrl Pts',(-55.4409334940953,60.008789039846,-10.));
#36515=CARTESIAN_POINT('Ctrl Pts',(-55.4574237999011,60.1438893245482,-10.));
#36516=CARTESIAN_POINT('Ctrl Pts',(-55.4736437641814,60.2767747796722,-10.));
#36517=CARTESIAN_POINT('Ctrl Pts',(-55.4957326625335,60.4089016790912,-10.));
#36518=CARTESIAN_POINT('Ctrl Pts',(-55.5237660357119,60.5398620252877,-10.));
#36519=CARTESIAN_POINT('Ctrl Pts',(-55.5366368863635,60.599989325932,-10.));
#36520=CARTESIAN_POINT('Ctrl Pts',(-55.5507614458456,60.6598704056294,-10.));
#36521=CARTESIAN_POINT('Ctrl Pts',(-55.5661502149289,60.7194638770806,-10.));
#36522=CARTESIAN_POINT('Ctrl Pts',(-55.5886111804506,60.8064446421006,-10.));
#36523=CARTESIAN_POINT('Ctrl Pts',(-55.6137651104405,60.8928130396799,-10.));
#36524=CARTESIAN_POINT('Ctrl Pts',(-55.6415741874814,60.9784471096742,-10.));
#36525=CARTESIAN_POINT('Ctrl Pts',(-55.6489435502234,61.0011400068149,-10.));
#36526=CARTESIAN_POINT('Ctrl Pts',(-55.6564994059424,61.023781297052,-10.));
#36527=CARTESIAN_POINT('Ctrl Pts',(-55.6642411296903,61.0463686223145,-10.));
#36528=CARTESIAN_POINT('Ctrl Pts',(-55.6712493359898,61.0668158302424,-10.));
#36529=CARTESIAN_POINT('Ctrl Pts',(-55.6784073088638,61.0872112882693,-10.));
#36530=CARTESIAN_POINT('Ctrl Pts',(-55.6857121883891,61.1075477764851,-10.));
#36531=CARTESIAN_POINT('Ctrl Pts',(-55.7311295763656,61.233987941882,-10.));
#36532=CARTESIAN_POINT('Ctrl Pts',(-55.7822461186853,61.3582207273371,-10.));
#36533=CARTESIAN_POINT('Ctrl Pts',(-55.8388703422329,61.4798690368619,-10.));
#36534=CARTESIAN_POINT('Ctrl Pts',(-55.8863606130665,61.5818944741014,-10.));
#36535=CARTESIAN_POINT('Ctrl Pts',(-55.9377259705942,61.6821017750024,-10.));
#36536=CARTESIAN_POINT('Ctrl Pts',(-55.9928752884837,61.7802503783273,-10.));
#36537=CARTESIAN_POINT('Ctrl Pts',(-56.0250178986502,61.8374542099573,-10.));
#36538=CARTESIAN_POINT('Ctrl Pts',(-56.058446233574,61.8939583886922,-10.));
#36539=CARTESIAN_POINT('Ctrl Pts',(-56.0931449406476,61.9497120817676,-10.));
#36540=CARTESIAN_POINT('Ctrl Pts',(-56.1050647419445,61.9688647534108,-10.));
#36541=CARTESIAN_POINT('Ctrl Pts',(-56.117135878067,61.9879310128291,-10.));
#36542=CARTESIAN_POINT('Ctrl Pts',(-56.1293531064626,62.0069015018125,-10.));
#36543=CARTESIAN_POINT('Ctrl Pts',(-56.2001801628626,62.1168793011676,-10.));
#36544=CARTESIAN_POINT('Ctrl Pts',(-56.2758314901157,62.2235154810087,-10.));
#36545=CARTESIAN_POINT('Ctrl Pts',(-56.3561468922528,62.3264414348563,-10.));
#36546=CARTESIAN_POINT('Ctrl Pts',(-56.4292340916213,62.420104287919,-10.));
#36547=CARTESIAN_POINT('Ctrl Pts',(-56.5061843400653,62.5106946453669,-10.));
#36548=CARTESIAN_POINT('Ctrl Pts',(-56.5869001850835,62.5979052562006,-10.));
#36549=CARTESIAN_POINT('Ctrl Pts',(-56.6479573239608,62.6638753315437,-10.));
#36550=CARTESIAN_POINT('Ctrl Pts',(-56.7111697701537,62.7279108548516,-10.));
#36551=CARTESIAN_POINT('Ctrl Pts',(-56.7764331619493,62.7899186857328,-10.));
#36552=CARTESIAN_POINT('Origin',(-60.,60.,-6.));
#36553=CARTESIAN_POINT('Origin',(60.,60.,-3.));
#36554=CARTESIAN_POINT('Ctrl Pts',(60.8043894954945,55.8135783132204,-3.));
#36555=CARTESIAN_POINT('Ctrl Pts',(60.6804230981971,55.7770540680639,-3.));
#36556=CARTESIAN_POINT('Ctrl Pts',(60.5549403090678,55.7463481935189,-3.));
#36557=CARTESIAN_POINT('Ctrl Pts',(60.4283617848279,55.7213771687008,-3.));
#36558=CARTESIAN_POINT('Ctrl Pts',(60.2999056253408,55.6960357297336,-3.));
#36559=CARTESIAN_POINT('Ctrl Pts',(60.1703203025177,55.6766003018695,-3.));
#36560=CARTESIAN_POINT('Ctrl Pts',(60.040018990912,55.6630301707006,-3.));
#36561=CARTESIAN_POINT('Ctrl Pts',(59.9818442061206,55.6569716019064,-3.));
#36562=CARTESIAN_POINT('Ctrl Pts',(59.9235264171928,55.652082796517,-2.99999999999999));
#36563=CARTESIAN_POINT('Ctrl Pts',(59.8651012902447,55.6483632564226,-2.99999999999999));
#36564=CARTESIAN_POINT('Ctrl Pts',(59.8415724912611,55.6468653339403,-2.99999999999999));
#36565=CARTESIAN_POINT('Ctrl Pts',(59.818026278381,55.6455570663652,-3.));
#36566=CARTESIAN_POINT('Ctrl Pts',(59.7944649611546,55.6444385115308,-3.));
#36567=CARTESIAN_POINT('Ctrl Pts',(59.771035780955,55.6433262297969,-3.));
#36568=CARTESIAN_POINT('Ctrl Pts',(59.7476011418858,55.6424020040368,-3.));
#36569=CARTESIAN_POINT('Ctrl Pts',(59.724166197105,55.6416655312924,-3.));
#36570=CARTESIAN_POINT('Ctrl Pts',(59.5904471279288,55.6374632406199,-3.));
#36571=CARTESIAN_POINT('Ctrl Pts',(59.4566904103623,55.6393684815201,-3.));
#36572=CARTESIAN_POINT('Ctrl Pts',(59.3233274428939,55.647328960846,-3.));
#36573=CARTESIAN_POINT('Ctrl Pts',(59.2153950098277,55.6537714832218,-3.));
#36574=CARTESIAN_POINT('Ctrl Pts',(59.1077198305457,55.6641809940724,-3.));
#36575=CARTESIAN_POINT('Ctrl Pts',(59.0005240806928,55.6785536426348,-3.));
#36576=CARTESIAN_POINT('Ctrl Pts',(58.9469262057664,55.685739966916,-3.));
#36577=CARTESIAN_POINT('Ctrl Pts',(58.8934481282158,55.6939174138492,-3.));
#36578=CARTESIAN_POINT('Ctrl Pts',(58.8401174407215,55.7030875592919,-3.));
#36579=CARTESIAN_POINT('Ctrl Pts',(58.8127285511832,55.7077970448129,-3.));
#36580=CARTESIAN_POINT('Ctrl Pts',(58.7853785354981,55.712768378203,-2.99999999999999));
#36581=CARTESIAN_POINT('Ctrl Pts',(58.7580711348704,55.7180019159915,-2.99999999999999));
#36582=CARTESIAN_POINT('Ctrl Pts',(58.7384796892885,55.7217566699567,-2.99999999999999));
#36583=CARTESIAN_POINT('Ctrl Pts',(58.7189124095391,55.7256460128853,-3.));
#36584=CARTESIAN_POINT('Ctrl Pts',(58.6993816125308,55.7296676040812,-3.));
#36585=CARTESIAN_POINT('Ctrl Pts',(58.693127863238,55.7309553151298,-3.));
#36586=CARTESIAN_POINT('Ctrl Pts',(58.6868775384995,55.7322566451671,-3.));
#36587=CARTESIAN_POINT('Ctrl Pts',(58.6806306833416,55.7335715858747,-3.));
#36588=CARTESIAN_POINT('Ctrl Pts',(58.5505754691102,55.7609477441344,-3.));
#36589=CARTESIAN_POINT('Ctrl Pts',(58.4220249805927,55.794218981014,-3.));
#36590=CARTESIAN_POINT('Ctrl Pts',(58.2953077479336,55.8330910870826,-3.));
#36591=CARTESIAN_POINT('Ctrl Pts',(58.1663246104551,55.8726582879748,-3.));
#36592=CARTESIAN_POINT('Ctrl Pts',(58.0392402106457,55.9180285436651,-3.));
#36593=CARTESIAN_POINT('Ctrl Pts',(57.9143961990582,55.9689453660749,-3.));
#36594=CARTESIAN_POINT('Ctrl Pts',(57.7879490069731,56.0205160352784,-3.));
#36595=CARTESIAN_POINT('Ctrl Pts',(57.6637993564696,56.077776790127,-3.));
#36596=CARTESIAN_POINT('Ctrl Pts',(57.5423081830428,56.1405139151216,-3.));
#36597=CARTESIAN_POINT('Ctrl Pts',(57.465938340702,56.1799507252997,-3.));
#36598=CARTESIAN_POINT('Ctrl Pts',(57.3906191333291,56.2215525292356,-3.));
#36599=CARTESIAN_POINT('Ctrl Pts',(57.3164434804249,56.2652762658272,-3.));
#36600=CARTESIAN_POINT('Ctrl Pts',(57.2554403025305,56.3012353275553,-3.));
#36601=CARTESIAN_POINT('Ctrl Pts',(57.1952106164062,56.3386297402385,-3.));
#36602=CARTESIAN_POINT('Ctrl Pts',(57.1358080455961,56.377439247764,-3.));
#36603=CARTESIAN_POINT('Ctrl Pts',(57.1208016710562,56.3872433689947,-3.));
#36604=CARTESIAN_POINT('Ctrl Pts',(57.1058499054844,56.3971366819327,-3.));
#36605=CARTESIAN_POINT('Ctrl Pts',(57.0909629618782,56.4071123926641,-3.));
#36606=CARTESIAN_POINT('Ctrl Pts',(56.9746406743767,56.4850597217074,-3.));
#36607=CARTESIAN_POINT('Ctrl Pts',(56.8621134355589,56.5681388647664,-3.));
#36608=CARTESIAN_POINT('Ctrl Pts',(56.7537376927601,56.6560786480786,-3.));
#36609=CARTESIAN_POINT('Ctrl Pts',(56.7306089015666,56.6748461400773,-3.));
#36610=CARTESIAN_POINT('Ctrl Pts',(56.7076692206168,56.6938351971782,-3.));
#36611=CARTESIAN_POINT('Ctrl Pts',(56.6849221758314,56.7130434825668,-3.));
#36612=CARTESIAN_POINT('Ctrl Pts',(56.5793101632974,56.8022254266987,-3.));
#36613=CARTESIAN_POINT('Ctrl Pts',(56.47784887195,56.896129304385,-3.));
#36614=CARTESIAN_POINT('Ctrl Pts',(56.380714466223,56.9943655777065,-3.));
#36615=CARTESIAN_POINT('Ctrl Pts',(56.2824676905965,57.093726839364,-3.));
#36616=CARTESIAN_POINT('Ctrl Pts',(56.188646908236,57.1975207658422,-3.));
#36617=CARTESIAN_POINT('Ctrl Pts',(56.0994624522646,57.3053895227055,-3.));
#36618=CARTESIAN_POINT('Ctrl Pts',(56.0193271754091,57.4023132814607,-3.));
#36619=CARTESIAN_POINT('Ctrl Pts',(55.9429351942092,57.5025277899424,-3.));
#36620=CARTESIAN_POINT('Ctrl Pts',(55.8704637655828,57.6057990864436,-3.));
#36621=CARTESIAN_POINT('Ctrl Pts',(55.8587177026021,57.6225371468875,-3.));
#36622=CARTESIAN_POINT('Ctrl Pts',(55.847074686451,57.6393555524523,-3.));
#36623=CARTESIAN_POINT('Ctrl Pts',(55.8355355388399,57.656253357144,-3.));
#36624=CARTESIAN_POINT('Ctrl Pts',(55.8253671008489,57.6711439092871,-3.));
#36625=CARTESIAN_POINT('Ctrl Pts',(55.8152846650618,57.6860882977166,-3.));
#36626=CARTESIAN_POINT('Ctrl Pts',(55.8052890498414,57.7010849236945,-3.));
#36627=CARTESIAN_POINT('Ctrl Pts',(55.7260105077896,57.8200281419958,-3.));
#36628=CARTESIAN_POINT('Ctrl Pts',(55.6521810643325,57.9422686678001,-3.));
#36629=CARTESIAN_POINT('Ctrl Pts',(55.5839783927012,58.0673941439682,-3.));
#36630=CARTESIAN_POINT('Ctrl Pts',(55.515043000026,58.1938638793468,-3.));
#36631=CARTESIAN_POINT('Ctrl Pts',(55.4518553517568,58.323281427723,-3.));
#36632=CARTESIAN_POINT('Ctrl Pts',(55.3946315085702,58.4552626427157,-3.));
#36633=CARTESIAN_POINT('Ctrl Pts',(55.3737738613536,58.5033687724028,-3.));
#36634=CARTESIAN_POINT('Ctrl Pts',(55.3537088867656,58.5518158526946,-3.));
#36635=CARTESIAN_POINT('Ctrl Pts',(55.3344483425769,58.6005864144814,-3.));
#36636=CARTESIAN_POINT('Ctrl Pts',(55.2818816840914,58.7336930100419,-3.));
#36637=CARTESIAN_POINT('Ctrl Pts',(55.235303613332,58.8692073967039,-3.));
#36638=CARTESIAN_POINT('Ctrl Pts',(55.1947264750797,59.0067151509791,-3.));
#36639=CARTESIAN_POINT('Ctrl Pts',(55.1709933297947,59.0871420034035,-3.));
#36640=CARTESIAN_POINT('Ctrl Pts',(55.1493139447911,59.1682512730649,-3.));
#36641=CARTESIAN_POINT('Ctrl Pts',(55.1296983939106,59.2499631634561,-3.));
#36642=CARTESIAN_POINT('Ctrl Pts',(55.1222104222649,59.2811555741154,-3.));
#36643=CARTESIAN_POINT('Ctrl Pts',(55.1150232579274,59.3124358186197,-3.));
#36644=CARTESIAN_POINT('Ctrl Pts',(55.1081376850014,59.3437995167499,-3.));
#36645=CARTESIAN_POINT('Ctrl Pts',(55.1026350847819,59.3688637915852,-3.));
#36646=CARTESIAN_POINT('Ctrl Pts',(55.0973242344235,59.3939859998928,-3.));
#36647=CARTESIAN_POINT('Ctrl Pts',(55.0922112631199,59.4191348146936,-3.));
#36648=CARTESIAN_POINT('Ctrl Pts',(55.0630684411167,59.5624775776013,-3.));
#36649=CARTESIAN_POINT('Ctrl Pts',(55.0403126175449,59.7068444399294,-3.));
#36650=CARTESIAN_POINT('Ctrl Pts',(55.0238938659507,59.851778335995,-3.));
#36651=CARTESIAN_POINT('Ctrl Pts',(55.0073130217029,59.9981430789608,-3.));
#36652=CARTESIAN_POINT('Ctrl Pts',(54.9971947543477,60.1450868240802,-3.));
#36653=CARTESIAN_POINT('Ctrl Pts',(54.9935344151175,60.2921650366492,-3.));
#36654=CARTESIAN_POINT('Ctrl Pts',(54.9898705323877,60.4393856326285,-3.));
#36655=CARTESIAN_POINT('Ctrl Pts',(54.9926769058727,60.5867417347185,-3.));
#36656=CARTESIAN_POINT('Ctrl Pts',(55.0019985535712,60.7338023176659,-3.));
#36657=CARTESIAN_POINT('Ctrl Pts',(55.007624235958,60.8225544522708,-3.));
#36658=CARTESIAN_POINT('Ctrl Pts',(55.0156238884368,60.9111991867765,-3.));
#36659=CARTESIAN_POINT('Ctrl Pts',(55.0260165827179,60.9996425537523,-3.));
#36660=CARTESIAN_POINT('Ctrl Pts',(55.0384683227897,61.1056087052492,-3.));
#36661=CARTESIAN_POINT('Ctrl Pts',(55.054354939434,61.2112859368579,-3.));
#36662=CARTESIAN_POINT('Ctrl Pts',(55.0736213347631,61.3165318688511,-3.));
#36663=CARTESIAN_POINT('Ctrl Pts',(56.3967816198432,63.6078550836889,-3.));
#36664=CARTESIAN_POINT('Ctrl Pts',(56.5101573278891,63.7040964917567,-3.));
#36665=CARTESIAN_POINT('Ctrl Pts',(56.6276776524244,63.7951366320638,-3.));
#36666=CARTESIAN_POINT('Ctrl Pts',(56.7489442704341,63.8807936755053,-3.));
#36667=CARTESIAN_POINT('Ctrl Pts',(56.8703218606103,63.9665291044734,-3.));
#36668=CARTESIAN_POINT('Ctrl Pts',(56.995453355925,64.0468718760484,-3.));
#36669=CARTESIAN_POINT('Ctrl Pts',(57.1239602399913,64.1215920780355,-3.));
#36670=CARTESIAN_POINT('Ctrl Pts',(57.1803120064737,64.1543577575125,-3.));
#36671=CARTESIAN_POINT('Ctrl Pts',(57.2373130376274,64.1860416170387,-3.));
#36672=CARTESIAN_POINT('Ctrl Pts',(57.2949321173609,64.2166211629568,-3.));
#36673=CARTESIAN_POINT('Ctrl Pts',(57.3242693742672,64.2321910054261,-3.));
#36674=CARTESIAN_POINT('Ctrl Pts',(57.3537668603064,64.2474745315704,-3.));
#36675=CARTESIAN_POINT('Ctrl Pts',(57.3834204755002,64.2624685748845,-3.));
#36676=CARTESIAN_POINT('Ctrl Pts',(57.4050341385029,64.2733972996662,-3.));
#36677=CARTESIAN_POINT('Ctrl Pts',(57.4267301365591,64.2841718530121,-3.));
#36678=CARTESIAN_POINT('Ctrl Pts',(57.4484948027175,64.294785320416,-3.));
#36679=CARTESIAN_POINT('Ctrl Pts',(57.5800080989128,64.3589173439526,-3.));
#36680=CARTESIAN_POINT('Ctrl Pts',(57.7141414686933,64.4172300576872,-3.));
#36681=CARTESIAN_POINT('Ctrl Pts',(57.8505256425866,64.4695128536294,-3.));
#36682=CARTESIAN_POINT('Ctrl Pts',(57.968432834675,64.5147125090446,-3.));
#36683=CARTESIAN_POINT('Ctrl Pts',(58.0880228412298,64.5554047505907,-3.));
#36684=CARTESIAN_POINT('Ctrl Pts',(58.2090619180921,64.5914221480058,-3.));
#36685=CARTESIAN_POINT('Ctrl Pts',(58.2695814565233,64.6094308467133,-3.00000000000001));
#36686=CARTESIAN_POINT('Ctrl Pts',(58.3304632962727,64.6262703667664,-3.00000000000001));
#36687=CARTESIAN_POINT('Ctrl Pts',(58.3916782037017,64.6419168917389,-3.00000000000001));
#36688=CARTESIAN_POINT('Ctrl Pts',(58.4205105124408,64.649286427325,-3.00000000000001));
#36689=CARTESIAN_POINT('Ctrl Pts',(58.4494167078449,64.6563912777525,-3.));
#36690=CARTESIAN_POINT('Ctrl Pts',(58.4783937204173,64.6632288012031,-3.));
#36691=CARTESIAN_POINT('Ctrl Pts',(58.5046585351189,64.6694263443763,-3.));
#36692=CARTESIAN_POINT('Ctrl Pts',(58.5309854155718,64.6754050197627,-3.));
#36693=CARTESIAN_POINT('Ctrl Pts',(58.5573454950175,64.6811572553105,-3.));
#36694=CARTESIAN_POINT('Ctrl Pts',(58.5636485802747,64.682532699992,-3.));
#36695=CARTESIAN_POINT('Ctrl Pts',(58.5699538441721,64.6838952676503,-3.00000000000001));
#36696=CARTESIAN_POINT('Ctrl Pts',(58.5762612548222,64.6852449426606,-3.00000000000001));
#36697=CARTESIAN_POINT('Ctrl Pts',(58.7158131526305,64.7151065958105,-3.00000000000001));
#36698=CARTESIAN_POINT('Ctrl Pts',(58.8564152550715,64.7386614193891,-3.));
#36699=CARTESIAN_POINT('Ctrl Pts',(58.9976457358102,64.7559650852701,-3.));
#36700=CARTESIAN_POINT('Ctrl Pts',(59.139815066942,64.7733837798151,-3.));
#36701=CARTESIAN_POINT('Ctrl Pts',(59.2826219755861,64.7844678684638,-3.));
#36702=CARTESIAN_POINT('Ctrl Pts',(59.4256369954039,64.7892215558739,-3.));
#36703=CARTESIAN_POINT('Ctrl Pts',(59.5672051822675,64.7939271518904,-3.));
#36704=CARTESIAN_POINT('Ctrl Pts',(59.7089780507634,64.792429595255,-3.));
#36705=CARTESIAN_POINT('Ctrl Pts',(59.8505280903461,64.784683690889,-3.));
#36706=CARTESIAN_POINT('Ctrl Pts',(59.9398961209693,64.77979329156,-3.));
#36707=CARTESIAN_POINT('Ctrl Pts',(60.0291750731265,64.7724112867483,-3.));
#36708=CARTESIAN_POINT('Ctrl Pts',(60.1182530286222,64.7625165118624,-3.));
#36709=CARTESIAN_POINT('Ctrl Pts',(60.1850614952439,64.7550954306981,-3.));
#36710=CARTESIAN_POINT('Ctrl Pts',(60.2517568353818,64.746260760684,-3.));
#36711=CARTESIAN_POINT('Ctrl Pts',(60.3182901338221,64.7360008324502,-3.));
#36712=CARTESIAN_POINT('Ctrl Pts',(60.335922917866,64.733281726332,-3.));
#36713=CARTESIAN_POINT('Ctrl Pts',(60.3535443117469,64.7304625022116,-3.));
#36714=CARTESIAN_POINT('Ctrl Pts',(60.3711533849972,64.7275429155473,-3.));
#36715=CARTESIAN_POINT('Ctrl Pts',(60.3893511940337,64.7245257164122,-3.));
#36716=CARTESIAN_POINT('Ctrl Pts',(60.4075271680476,64.7214027597405,-3.));
#36717=CARTESIAN_POINT('Ctrl Pts',(60.4256777486191,64.718174556807,-3.));
#36718=CARTESIAN_POINT('Ctrl Pts',(60.5629885227604,64.693752911332,-3.));
#36719=CARTESIAN_POINT('Ctrl Pts',(60.6988965337467,64.6633038922754,-3.));
#36720=CARTESIAN_POINT('Ctrl Pts',(60.8330040002292,64.6268299926211,-3.));
#36721=CARTESIAN_POINT('Ctrl Pts',(60.8581918055621,64.6199795352355,-3.));
#36722=CARTESIAN_POINT('Ctrl Pts',(60.8833160533696,64.6129164047735,-3.));
#36723=CARTESIAN_POINT('Ctrl Pts',(60.9083740419004,64.6056404226031,-3.));
#36724=CARTESIAN_POINT('Ctrl Pts',(61.0423381249251,64.566741838291,-3.00000000000001));
#36725=CARTESIAN_POINT('Ctrl Pts',(61.1744105226846,64.5217632900704,-3.));
#36726=CARTESIAN_POINT('Ctrl Pts',(61.3042176288045,64.4709134975508,-3.));
#36727=CARTESIAN_POINT('Ctrl Pts',(61.4335909730649,64.4202336240844,-3.));
#36728=CARTESIAN_POINT('Ctrl Pts',(61.5607147887615,64.3637211759828,-3.));
#36729=CARTESIAN_POINT('Ctrl Pts',(61.6851875383315,64.3015421572917,-3.));
#36730=CARTESIAN_POINT('Ctrl Pts',(61.7912746295725,64.2485474957939,-3.));
#36731=CARTESIAN_POINT('Ctrl Pts',(61.895435682969,64.1914358019316,-3.));
#36732=CARTESIAN_POINT('Ctrl Pts',(61.9973985420836,64.1302904783211,-3.00000000000001));
#36733=CARTESIAN_POINT('Ctrl Pts',(62.0157427331232,64.1192897913335,-3.00000000000001));
#36734=CARTESIAN_POINT('Ctrl Pts',(62.0340157094886,64.1081585033305,-3.));
#36735=CARTESIAN_POINT('Ctrl Pts',(62.052215799533,64.0968970474319,-3.));
#36736=CARTESIAN_POINT('Ctrl Pts',(62.0686109323645,64.086752423703,-3.));
#36737=CARTESIAN_POINT('Ctrl Pts',(62.0849390653794,64.0765070092133,-3.));
#36738=CARTESIAN_POINT('Ctrl Pts',(62.1011957941185,64.0661635944481,-3.));
#36739=CARTESIAN_POINT('Ctrl Pts',(62.2160942895865,63.9930589241547,-3.));
#36740=CARTESIAN_POINT('Ctrl Pts',(62.3274845529479,63.9150275718819,-3.));
#36741=CARTESIAN_POINT('Ctrl Pts',(62.4350222646538,63.8322713282373,-3.));
#36742=CARTESIAN_POINT('Ctrl Pts',(62.5416034782076,63.7502511630611,-3.));
#36743=CARTESIAN_POINT('Ctrl Pts',(62.6444009200186,63.6635892555824,-3.));
#36744=CARTESIAN_POINT('Ctrl Pts',(62.7430433478219,63.5724461389909,-3.));
#36745=CARTESIAN_POINT('Ctrl Pts',(62.7758260127342,63.5421557830373,-3.));
#36746=CARTESIAN_POINT('Ctrl Pts',(62.808149428445,63.5113702208032,-3.));
#36747=CARTESIAN_POINT('Ctrl Pts',(62.8399989163846,63.4800946064471,-3.));
#36748=CARTESIAN_POINT('Ctrl Pts',(62.9365720682666,63.3852615384508,-3.));
#36749=CARTESIAN_POINT('Ctrl Pts',(63.0287914724018,63.2859242142018,-3.));
#36750=CARTESIAN_POINT('Ctrl Pts',(63.116384688617,63.1824188586198,-3.));
#36751=CARTESIAN_POINT('Ctrl Pts',(63.1636033936845,63.1266224274654,-3.));
#36752=CARTESIAN_POINT('Ctrl Pts',(63.2094769322843,63.0696144553279,-3.));
#36753=CARTESIAN_POINT('Ctrl Pts',(63.2539565107167,63.0114459571216,-3.));
#36754=CARTESIAN_POINT('Ctrl Pts',(63.2715142364304,62.9884847112493,-3.));
#36755=CARTESIAN_POINT('Ctrl Pts',(63.2888547102122,62.9653426270302,-3.));
#36756=CARTESIAN_POINT('Ctrl Pts',(63.3059747354259,62.942022815916,-3.));
#36757=CARTESIAN_POINT('Ctrl Pts',(63.3199565107891,62.9229777294489,-3.));
#36758=CARTESIAN_POINT('Ctrl Pts',(63.3337935971807,62.9038106514913,-3.));
#36759=CARTESIAN_POINT('Ctrl Pts',(63.3474682801689,62.8845461191246,-3.));
#36760=CARTESIAN_POINT('Ctrl Pts',(63.4242351022266,62.7763990469401,-3.));
#36761=CARTESIAN_POINT('Ctrl Pts',(63.4959842559734,62.6650546750512,-3.));
#36762=CARTESIAN_POINT('Ctrl Pts',(63.5625180995312,62.5508627289101,-3.));
#36763=CARTESIAN_POINT('Ctrl Pts',(63.6288088601457,62.4370879856974,-3.));
#36764=CARTESIAN_POINT('Ctrl Pts',(63.6899226483436,62.3204856807288,-3.));
#36765=CARTESIAN_POINT('Ctrl Pts',(63.7456163613347,62.2013821649674,-3.));
#36766=CARTESIAN_POINT('Ctrl Pts',(63.8003210691109,62.0843936814399,-3.));
#36767=CARTESIAN_POINT('Ctrl Pts',(63.8497966468504,61.9649913311224,-3.));
#36768=CARTESIAN_POINT('Ctrl Pts',(63.8937635139461,61.8434762846442,-3.));
#36769=CARTESIAN_POINT('Ctrl Pts',(63.9160764497028,61.7818080875531,-3.));
#36770=CARTESIAN_POINT('Ctrl Pts',(63.9369698093169,61.7195956989266,-3.));
#36771=CARTESIAN_POINT('Ctrl Pts',(63.9564018718053,61.6568785193336,-3.));
#36772=CARTESIAN_POINT('Ctrl Pts',(63.9829907032676,61.5710627949871,-3.));
#36773=CARTESIAN_POINT('Ctrl Pts',(64.0068439948043,61.4843017745449,-3.));
#36774=CARTESIAN_POINT('Ctrl Pts',(64.0279238903325,61.3967314318667,-3.));
#36775=CARTESIAN_POINT('Origin',(60.,60.,-13.3123464956316));
#36776=CARTESIAN_POINT('Ctrl Pts',(65.0992547463301,60.0000912484111,-9.56234649563159));
#36777=CARTESIAN_POINT('Ctrl Pts',(65.0993446065218,60.1069729367835,-9.55734157105847));
#36778=CARTESIAN_POINT('Ctrl Pts',(65.0703981457348,61.0460695286254,-9.51336443385491));
#36779=CARTESIAN_POINT('Ctrl Pts',(64.5173398680237,62.7859966304905,-9.43041508402093));
#36780=CARTESIAN_POINT('Ctrl Pts',(62.6758304956081,64.5834554024384,-9.31349844612963));
#36781=CARTESIAN_POINT('Ctrl Pts',(60.205263132424,65.3033953276082,-9.19658180823835));
#36782=CARTESIAN_POINT('Ctrl Pts',(57.6864406181491,64.7765653538453,-9.07966517034705));
#36783=CARTESIAN_POINT('Ctrl Pts',(55.7115103282802,63.1268179703927,-8.96274853245576));
#36784=CARTESIAN_POINT('Ctrl Pts',(54.7447564613263,60.7419901067622,-8.84583189456447));
#36785=CARTESIAN_POINT('Ctrl Pts',(55.0134521769933,58.1827288792718,-8.72891525667318));
#36786=CARTESIAN_POINT('Ctrl Pts',(56.4544300560118,56.0506873938616,-8.6119986187819));
#36787=CARTESIAN_POINT('Ctrl Pts',(58.7289322067895,54.8470867941934,-8.49508198089061));
#36788=CARTESIAN_POINT('Ctrl Pts',(61.3022482494153,54.8548764161609,-8.37816534299932));
#36789=CARTESIAN_POINT('Ctrl Pts',(63.5694203037008,56.0722332749569,-8.26124870510803));
#36790=CARTESIAN_POINT('Ctrl Pts',(64.8552427510861,57.9997589069056,-8.15597575598545));
#36791=CARTESIAN_POINT('Ctrl Pts',(65.0983472268173,59.4163728002799,-8.08967501949331));
#36792=CARTESIAN_POINT('Ctrl Pts',(65.098848108647,60.0001169986396,-8.06234649563159));
#36793=CARTESIAN_POINT('Ctrl Pts',(65.0987893697715,60.0001196244759,-9.68765350436842));
#36794=CARTESIAN_POINT('Ctrl Pts',(65.0989958456617,60.2735580353962,-9.67485236502099));
#36795=CARTESIAN_POINT('Ctrl Pts',(65.0114730664976,61.3793292170961,-9.62307901304313));
#36796=CARTESIAN_POINT('Ctrl Pts',(64.2231822164303,63.2145072853594,-9.53233344843484));
#36797=CARTESIAN_POINT('Ctrl Pts',(62.2146698080337,64.8232034325914,-9.41541681054355));
#36798=CARTESIAN_POINT('Ctrl Pts',(59.6855379323249,65.2980445186201,-9.29850017265226));
#36799=CARTESIAN_POINT('Ctrl Pts',(57.2303209838473,64.5273621068898,-9.18158353476097));
#36800=CARTESIAN_POINT('Ctrl Pts',(55.4262302676069,62.6923526051193,-9.06466689686969));
#36801=CARTESIAN_POINT('Ctrl Pts',(54.6973796845391,60.2243982381535,-8.94775025897839));
#36802=CARTESIAN_POINT('Ctrl Pts',(55.2151175810578,57.7036915329656,-8.8308336210871));
#36803=CARTESIAN_POINT('Ctrl Pts',(56.8577278151099,55.7228209598733,-8.71391698319582));
#36804=CARTESIAN_POINT('Ctrl Pts',(59.2390517104132,54.7474680995942,-8.59700034530453));
#36805=CARTESIAN_POINT('Ctrl Pts',(61.799265976347,55.0069271683894,-8.48008370741324));
#36806=CARTESIAN_POINT('Ctrl Pts',(63.9364928560947,56.4402025290253,-8.36316706952195));
#36807=CARTESIAN_POINT('Ctrl Pts',(64.9468057472684,58.3328863836753,-8.26569033517367));
#36808=CARTESIAN_POINT('Ctrl Pts',(65.0986023825915,59.5827292143741,-8.20718581345583));
#36809=CARTESIAN_POINT('Ctrl Pts',(65.0986049232486,60.0000009026908,-8.18765350436841));
#36810=CARTESIAN_POINT('Ctrl Pts',(56.7766472160421,62.7898325810254,-10.));
#36811=CARTESIAN_POINT('Ctrl Pts',(56.3212170277455,62.2636317705077,-9.96102778736957));
#36812=CARTESIAN_POINT('Ctrl Pts',(55.6734220606415,60.9843943012708,-9.88308336210871));
#36813=CARTESIAN_POINT('Ctrl Pts',(55.7189117270138,58.8332763305925,-9.76616672421742));
#36814=CARTESIAN_POINT('Ctrl Pts',(56.7709224287295,56.9567114979888,-9.64925008632613));
#36815=CARTESIAN_POINT('Ctrl Pts',(58.582037303137,55.7954439707652,-9.53233344843484));
#36816=CARTESIAN_POINT('Ctrl Pts',(60.7265123733809,55.6226835105978,-9.41541681054355));
#36817=CARTESIAN_POINT('Ctrl Pts',(62.7001876951902,56.4789515650734,-9.29850017265227));
#36818=CARTESIAN_POINT('Ctrl Pts',(64.0390812605523,58.1629928045498,-9.18158353476097));
#36819=CARTESIAN_POINT('Ctrl Pts',(64.4284304613218,60.2788876953404,-9.06466689686969));
#36820=CARTESIAN_POINT('Ctrl Pts',(63.7767052083516,62.329222129002,-8.94775025897839));
#36821=CARTESIAN_POINT('Ctrl Pts',(62.2371181413566,63.8319808551863,-8.8308336210871));
#36822=CARTESIAN_POINT('Ctrl Pts',(60.1716094790201,64.433883954029,-8.71391698319582));
#36823=CARTESIAN_POINT('Ctrl Pts',(58.0657572769503,63.9934297123833,-8.59700034530453));
#36824=CARTESIAN_POINT('Ctrl Pts',(56.414624147766,62.6141645435937,-8.48008370741324));
#36825=CARTESIAN_POINT('Ctrl Pts',(55.6063731701577,60.6203380712154,-8.36316706952195));
#36826=CARTESIAN_POINT('Ctrl Pts',(55.8310152246563,58.4806772332488,-8.24625043163065));
#36827=CARTESIAN_POINT('Ctrl Pts',(57.0357394251379,56.6981918729225,-8.12933379373937));
#36828=CARTESIAN_POINT('Ctrl Pts',(58.9373284953018,55.6919260646492,-8.01241715584808));
#36829=CARTESIAN_POINT('Ctrl Pts',(61.0887398092287,55.6984385491457,-7.89550051795679));
#36830=CARTESIAN_POINT('Ctrl Pts',(62.984200579462,56.7162052267388,-7.7785838800655));
#36831=CARTESIAN_POINT('Ctrl Pts',(64.1781085527216,58.5059455017865,-7.66166724217421));
#36832=CARTESIAN_POINT('Ctrl Pts',(64.3897900743559,60.6469434568749,-7.54475060428292));
#36833=CARTESIAN_POINT('Ctrl Pts',(63.5694792390211,62.6358046484627,-7.42783396639163));
#36834=CARTESIAN_POINT('Ctrl Pts',(61.9100261920983,64.0051199372434,-7.31091732850034));
#36835=CARTESIAN_POINT('Ctrl Pts',(59.8015410025307,64.4326543606342,-7.19400069060905));
#36836=CARTESIAN_POINT('Ctrl Pts',(57.7397245218596,63.8185989207299,-7.07708405271776));
#36837=CARTESIAN_POINT('Ctrl Pts',(56.2092450962316,62.3058003341377,-6.96016741482647));
#36838=CARTESIAN_POINT('Ctrl Pts',(55.5699912429921,60.2531607317565,-6.84325077693518));
#36839=CARTESIAN_POINT('Ctrl Pts',(55.9720481528381,58.1361860697788,-6.72633413904389));
#36840=CARTESIAN_POINT('Ctrl Pts',(57.3213012555681,56.4677215227762,-6.60941750115261));
#36841=CARTESIAN_POINT('Ctrl Pts',(59.9592774377706,55.3204052536368,-6.45352865063088));
#36842=CARTESIAN_POINT('Ctrl Pts',(63.6618728268516,56.5785257712713,-6.25866758747874));
#36843=CARTESIAN_POINT('Ctrl Pts',(64.8778949937948,61.1497560295123,-6.02483431169615));
#36844=CARTESIAN_POINT('Ctrl Pts',(62.2898185828427,64.0812983442691,-5.82997324854401));
#36845=CARTESIAN_POINT('Ctrl Pts',(59.4304505580215,64.3963657306031,-5.67408439802229));
#36846=CARTESIAN_POINT('Ctrl Pts',(57.430523426142,63.6188380159844,-5.557167760131));
#36847=CARTESIAN_POINT('Ctrl Pts',(56.0297438251523,61.9814474127173,-5.44025112223971));
#36848=CARTESIAN_POINT('Ctrl Pts',(55.5646049319228,59.8824903773911,-5.32333448434842));
#36849=CARTESIAN_POINT('Ctrl Pts',(56.1411247152275,57.8091954694446,-5.20641784645712));
#36850=CARTESIAN_POINT('Ctrl Pts',(57.6253116388877,56.2518450082663,-5.08950120856584));
#36851=CARTESIAN_POINT('Ctrl Pts',(59.6675354017074,55.5752228240151,-4.97258457067455));
#36852=CARTESIAN_POINT('Ctrl Pts',(61.7880226520381,55.9390120440154,-4.85566793278326));
#36853=CARTESIAN_POINT('Ctrl Pts',(63.4881170626526,57.2574041330032,-4.73875129489197));
#36854=CARTESIAN_POINT('Ctrl Pts',(64.3682162435255,59.2205920361106,-4.62183465700068));
#36855=CARTESIAN_POINT('Ctrl Pts',(64.2213857418157,61.3669907186962,-4.50491801910939));
#36856=CARTESIAN_POINT('Ctrl Pts',(63.082159015354,63.1920340067288,-4.3880013812181));
#36857=CARTESIAN_POINT('Ctrl Pts',(61.2183485912993,64.2666612780442,-4.27108474332681));
#36858=CARTESIAN_POINT('Ctrl Pts',(59.0681189506421,64.3382456551615,-4.15416810543553));
#36859=CARTESIAN_POINT('Ctrl Pts',(57.1369637190351,63.3899556120333,-4.03725146754423));
#36860=CARTESIAN_POINT('Ctrl Pts',(55.8788769012213,61.6447249674203,-3.92033482965294));
#36861=CARTESIAN_POINT('Ctrl Pts',(55.5896202577371,59.5128374687636,-3.80341819176165));
#36862=CARTESIAN_POINT('Ctrl Pts',(56.3371953964416,57.4954766475313,-3.68650155387037));
#36863=CARTESIAN_POINT('Ctrl Pts',(57.945854696259,56.0669013403294,-3.56958491597907));
#36864=CARTESIAN_POINT('Ctrl Pts',(60.0374221729278,55.5629543318799,-3.45266827808779));
#36865=CARTESIAN_POINT('Ctrl Pts',(62.1201892005749,56.1021068992122,-3.3357516401965));
#36866=CARTESIAN_POINT('Ctrl Pts',(63.7045295307839,57.5576125154289,-3.21883500230521));
#36867=CARTESIAN_POINT('Ctrl Pts',(64.417962512424,59.5872929422394,-3.10191836441392));
#36868=CARTESIAN_POINT('Ctrl Pts',(64.0928111357616,61.7140030980687,-2.98500172652263));
#36869=CARTESIAN_POINT('Ctrl Pts',(62.805423754937,63.4377528158129,-2.86808508863134));
#36870=CARTESIAN_POINT('Ctrl Pts',(60.858656910251,64.3533514942534,-2.75116845074005));
#36871=CARTESIAN_POINT('Ctrl Pts',(58.7097667243778,64.2454218753984,-2.63425181284876));
#36872=CARTESIAN_POINT('Ctrl Pts',(57.4799483719373,63.5081067174902,-2.5563073875879));
#36873=CARTESIAN_POINT('Ctrl Pts',(56.9875426643247,63.0163338344315,-2.51733517495747));
#36874=CARTESIAN_POINT('Ctrl Pts',(56.5659409116095,62.9722002436837,-10.1608882750142));
#36875=CARTESIAN_POINT('Ctrl Pts',(56.0807398547996,62.4116023827639,-10.1219160623837));
#36876=CARTESIAN_POINT('Ctrl Pts',(55.390599388243,61.0487428536097,-10.0439716371229));
#36877=CARTESIAN_POINT('Ctrl Pts',(55.4390626538871,58.7570091488251,-9.9270549992316));
#36878=CARTESIAN_POINT('Ctrl Pts',(56.5598419025287,56.757775757299,-9.8101383613403));
#36879=CARTESIAN_POINT('Ctrl Pts',(58.4893469587335,55.5205977090997,-9.69322172344902));
#36880=CARTESIAN_POINT('Ctrl Pts',(60.7740035254761,55.3365441263504,-9.57630508555772));
#36881=CARTESIAN_POINT('Ctrl Pts',(62.8766953903328,56.2487852900246,-9.45938844766644));
#36882=CARTESIAN_POINT('Ctrl Pts',(64.3031106556436,58.0429100760021,-9.34247180977514));
#36883=CARTESIAN_POINT('Ctrl Pts',(64.7179110982492,60.297118214795,-9.22555517188386));
#36884=CARTESIAN_POINT('Ctrl Pts',(64.0235834282423,62.4814802961648,-9.10863853399257));
#36885=CARTESIAN_POINT('Ctrl Pts',(62.3833555927738,64.0824723709371,-8.99172189610128));
#36886=CARTESIAN_POINT('Ctrl Pts',(60.1828273634881,64.7237210785554,-8.87480525820999));
#36887=CARTESIAN_POINT('Ctrl Pts',(57.9393183906832,64.254474926204,-8.7578886203187));
#36888=CARTESIAN_POINT('Ctrl Pts',(56.1802528746041,62.7850490191933,-8.64097198242741));
#36889=CARTESIAN_POINT('Ctrl Pts',(55.3191676005472,60.660888749731,-8.52405534453612));
#36890=CARTESIAN_POINT('Ctrl Pts',(55.5584942087686,58.3813611152564,-8.40713870664483));
#36891=CARTESIAN_POINT('Ctrl Pts',(56.8419696354292,56.4823570465689,-8.29022206875355));
#36892=CARTESIAN_POINT('Ctrl Pts',(58.8678630657977,55.4103129744973,-8.17330543086225));
#36893=CARTESIAN_POINT('Ctrl Pts',(61.1599092892909,55.4172511714842,-8.05638879297097));
#36894=CARTESIAN_POINT('Ctrl Pts',(63.1792738208749,56.5015479094781,-7.93947215507968));
#36895=CARTESIAN_POINT('Ctrl Pts',(64.4512259778585,58.4082811370585,-7.82255551718838));
#36896=CARTESIAN_POINT('Ctrl Pts',(64.6767448403393,60.6892332942311,-7.7056388792971));
#36897=CARTESIAN_POINT('Ctrl Pts',(63.8028113716211,62.8081037090707,-7.58872224140581));
#36898=CARTESIAN_POINT('Ctrl Pts',(62.0348820757948,64.2669293255877,-7.47180560351452));
#36899=CARTESIAN_POINT('Ctrl Pts',(59.788568000585,64.7224111082681,-7.35488896562323));
#36900=CARTESIAN_POINT('Ctrl Pts',(57.5919733059925,64.0682156771401,-7.23797232773193));
#36901=CARTESIAN_POINT('Ctrl Pts',(55.9614484663504,62.4565274495758,-7.12105568984065));
#36902=CARTESIAN_POINT('Ctrl Pts',(55.280407434965,60.2697095136588,-7.00413905194936));
#36903=CARTESIAN_POINT('Ctrl Pts',(55.7087462727672,58.0143510204657,-6.88722241405807));
#36904=CARTESIAN_POINT('Ctrl Pts',(57.1461982646896,56.2368211547287,-6.77030577616678));
#36905=CARTESIAN_POINT('Ctrl Pts',(59.956615457786,55.014506339886,-6.61441692564507));
#36906=CARTESIAN_POINT('Ctrl Pts',(63.901244605978,56.354868530266,-6.41955586249291));
#36907=CARTESIAN_POINT('Ctrl Pts',(65.1967565322115,61.2249140591216,-6.18572258671033));
#36908=CARTESIAN_POINT('Ctrl Pts',(62.4395009923554,64.3480874142361,-5.99086152355818));
#36909=CARTESIAN_POINT('Ctrl Pts',(59.3932198649654,64.6837503385306,-5.83497267303646));
#36910=CARTESIAN_POINT('Ctrl Pts',(57.2625601439663,63.8553966664936,-5.71805603514517));
#36911=CARTESIAN_POINT('Ctrl Pts',(55.7702134348034,62.1109720070587,-5.60113939725388));
#36912=CARTESIAN_POINT('Ctrl Pts',(55.2746690278715,59.8748089289196,-5.48422275936259));
#36913=CARTESIAN_POINT('Ctrl Pts',(55.8888751462175,57.6659854774559,-5.3673061214713));
#36914=CARTESIAN_POINT('Ctrl Pts',(57.4700814043196,56.0068330782413,-5.25038948358001));
#36915=CARTESIAN_POINT('Ctrl Pts',(59.6458026310317,55.2859809975139,-5.13347284568873));
#36916=CARTESIAN_POINT('Ctrl Pts',(61.9049033258284,55.6735506372437,-5.01655620779744));
#36917=CARTESIAN_POINT('Ctrl Pts',(63.7161306574902,57.0781242718092,-4.89963956990615));
#36918=CARTESIAN_POINT('Ctrl Pts',(64.6537607567468,59.1696431692867,-4.78272293201486));
#36919=CARTESIAN_POINT('Ctrl Pts',(64.4973321395136,61.4563490923634,-4.66580629412357));
#36920=CARTESIAN_POINT('Ctrl Pts',(63.2836356700444,63.4006930441535,-4.54888965623228));
#36921=CARTESIAN_POINT('Ctrl Pts',(61.29799042587,64.5455672776098,-4.43197301834099));
#36922=CARTESIAN_POINT('Ctrl Pts',(59.007203120064,64.6218310306964,-4.3150563804497));
#36923=CARTESIAN_POINT('Ctrl Pts',(56.9498108274184,63.6115525227894,-4.19813974255841));
#36924=CARTESIAN_POINT('Ctrl Pts',(55.6094845397717,61.7522384612638,-4.08122310466712));
#36925=CARTESIAN_POINT('Ctrl Pts',(55.3013195724191,59.4809922989995,-3.96430646677583));
#36926=CARTESIAN_POINT('Ctrl Pts',(56.0977627083054,57.3317592714531,-3.84738982888454));
#36927=CARTESIAN_POINT('Ctrl Pts',(57.8115779370184,55.8097998875587,-3.73047319099325));
#36928=CARTESIAN_POINT('Ctrl Pts',(60.0398684108329,55.2729105302888,-3.61355655310196));
#36929=CARTESIAN_POINT('Ctrl Pts',(62.2587831619229,55.8473067872207,-3.49663991521067));
#36930=CARTESIAN_POINT('Ctrl Pts',(63.9466897221777,57.3979568787802,-3.37972327731938));
#36931=CARTESIAN_POINT('Ctrl Pts',(64.7067588733894,59.5603148282126,-3.26280663942809));
#36932=CARTESIAN_POINT('Ctrl Pts',(64.360352781668,61.8260452116026,-3.14589000153681));
#36933=CARTESIAN_POINT('Ctrl Pts',(62.9888105919944,63.6624741665064,-3.02897336364551));
#36934=CARTESIAN_POINT('Ctrl Pts',(60.9147861757894,64.6379243184927,-2.91205672575423));
#36935=CARTESIAN_POINT('Ctrl Pts',(58.6254258831533,64.5229394833297,-2.79514008786294));
#36936=CARTESIAN_POINT('Ctrl Pts',(57.3152159330398,63.7374270096024,-2.71719566260208));
#36937=CARTESIAN_POINT('Ctrl Pts',(56.7906223161642,63.213507584184,-2.67822344997165));
#36938=CARTESIAN_POINT('Ctrl Pts',(56.3552346071769,63.1545679063421,-10.3217765500284));
#36939=CARTESIAN_POINT('Ctrl Pts',(55.8402626818537,62.55957299502,-10.2828043373979));
#36940=CARTESIAN_POINT('Ctrl Pts',(55.1077767158446,61.1130914059486,-10.2048599121371));
#36941=CARTESIAN_POINT('Ctrl Pts',(55.1592135807605,58.6807419670576,-10.0879432742458));
#36942=CARTESIAN_POINT('Ctrl Pts',(56.3487613763279,56.5588400166092,-9.97102663635448));
#36943=CARTESIAN_POINT('Ctrl Pts',(58.3966566143299,55.2457514474342,-9.8541099984632));
#36944=CARTESIAN_POINT('Ctrl Pts',(60.8214946775714,55.0504047421029,-9.7371933605719));
#36945=CARTESIAN_POINT('Ctrl Pts',(63.0532030854754,56.0186190149759,-9.62027672268062));
#36946=CARTESIAN_POINT('Ctrl Pts',(64.5671400507348,57.9228273474544,-9.50336008478932));
#36947=CARTESIAN_POINT('Ctrl Pts',(65.0073917351767,60.3153487342495,-9.38644344689804));
#36948=CARTESIAN_POINT('Ctrl Pts',(64.270461648133,62.6337384633277,-9.26952680900675));
#36949=CARTESIAN_POINT('Ctrl Pts',(62.529593044191,64.3329638866877,-9.15261017111546));
#36950=CARTESIAN_POINT('Ctrl Pts',(60.194045247956,65.0135582030818,-9.03569353322417));
#36951=CARTESIAN_POINT('Ctrl Pts',(57.8128795044162,64.5155201400246,-8.91877689533288));
#36952=CARTESIAN_POINT('Ctrl Pts',(55.9458816014421,62.9559334947931,-8.80186025744159));
#36953=CARTESIAN_POINT('Ctrl Pts',(55.0319620309368,60.7014394282466,-8.6849436195503));
#36954=CARTESIAN_POINT('Ctrl Pts',(55.285973192881,58.2820449972641,-8.56802698165901));
#36955=CARTESIAN_POINT('Ctrl Pts',(56.6481998457205,56.2665222202153,-8.45111034376772));
#36956=CARTESIAN_POINT('Ctrl Pts',(58.7983976362936,55.1286998843454,-8.33419370587643));
#36957=CARTESIAN_POINT('Ctrl Pts',(61.2310787693531,55.1360637938226,-8.21727706798514));
#36958=CARTESIAN_POINT('Ctrl Pts',(63.3743470622879,56.2868905922175,-8.10036043009385));
#36959=CARTESIAN_POINT('Ctrl Pts',(64.7243434029953,58.3106167723305,-7.98344379220256));
#36960=CARTESIAN_POINT('Ctrl Pts',(64.9636996063227,60.7315231315872,-7.86652715431127));
#36961=CARTESIAN_POINT('Ctrl Pts',(64.0361435042211,62.9804027696786,-7.74961051641998));
#36962=CARTESIAN_POINT('Ctrl Pts',(62.1597379594913,64.528738713932,-7.63269387852869));
#36963=CARTESIAN_POINT('Ctrl Pts',(59.7755949986392,65.0121678559021,-7.5157772406374));
#36964=CARTESIAN_POINT('Ctrl Pts',(57.4442220901253,64.3178324335504,-7.39886060274612));
#36965=CARTESIAN_POINT('Ctrl Pts',(55.7136518364692,62.6072545650141,-7.28194396485483));
#36966=CARTESIAN_POINT('Ctrl Pts',(54.9908236269379,60.2862582955611,-7.16502732696353));
#36967=CARTESIAN_POINT('Ctrl Pts',(55.4454443926962,57.8925159711526,-7.04811068907225));
#36968=CARTESIAN_POINT('Ctrl Pts',(56.9710952738111,56.0059207866812,-6.93119405118096));
#36969=CARTESIAN_POINT('Ctrl Pts',(59.9539534778013,54.7086074261351,-6.77530520065924));
#36970=CARTESIAN_POINT('Ctrl Pts',(64.1406163851045,56.1312112892607,-6.58044413750709));
#36971=CARTESIAN_POINT('Ctrl Pts',(65.5156180706283,61.3000720887308,-6.34661086172451));
#36972=CARTESIAN_POINT('Ctrl Pts',(62.5891834018679,64.6148764842033,-6.15174979857236));
#36973=CARTESIAN_POINT('Ctrl Pts',(59.3559891719093,64.9711349464581,-5.99586094805064));
#36974=CARTESIAN_POINT('Ctrl Pts',(57.0945968617905,64.0919553170029,-5.87894431015935));
#36975=CARTESIAN_POINT('Ctrl Pts',(55.5106830444545,62.2404966014001,-5.76202767226806));
#36976=CARTESIAN_POINT('Ctrl Pts',(54.9847331238201,59.8671274804482,-5.64511103437677));
#36977=CARTESIAN_POINT('Ctrl Pts',(55.6366255772074,57.5227754854671,-5.52819439648548));
#36978=CARTESIAN_POINT('Ctrl Pts',(57.3148511697517,55.7618211482163,-5.41127775859419));
#36979=CARTESIAN_POINT('Ctrl Pts',(59.6240698603559,54.9967391710128,-5.2943611207029));
#36980=CARTESIAN_POINT('Ctrl Pts',(62.0217839996187,55.408089230472,-5.17744448281161));
#36981=CARTESIAN_POINT('Ctrl Pts',(63.9441442523277,56.8988444106153,-5.06052784492032));
#36982=CARTESIAN_POINT('Ctrl Pts',(64.9393052699681,59.1186943024627,-4.94361120702903));
#36983=CARTESIAN_POINT('Ctrl Pts',(64.7732785372114,61.5457074660306,-4.82669456913774));
#36984=CARTESIAN_POINT('Ctrl Pts',(63.4851123247348,63.6093520815783,-4.70977793124645));
#36985=CARTESIAN_POINT('Ctrl Pts',(61.3776322604409,64.8244732771755,-4.59286129335517));
#36986=CARTESIAN_POINT('Ctrl Pts',(58.9462872894859,64.9054164062312,-4.47594465546388));
#36987=CARTESIAN_POINT('Ctrl Pts',(56.7626579358016,63.8331494335455,-4.35902801757259));
#36988=CARTESIAN_POINT('Ctrl Pts',(55.3400921783221,61.8597519551072,-4.2421113796813));
#36989=CARTESIAN_POINT('Ctrl Pts',(55.0130188871011,59.4491471292353,-4.12519474179001));
#36990=CARTESIAN_POINT('Ctrl Pts',(55.8583300201691,57.168041895375,-4.00827810389872));
#36991=CARTESIAN_POINT('Ctrl Pts',(57.6773011777778,55.552698434788,-3.89136146600743));
#36992=CARTESIAN_POINT('Ctrl Pts',(60.0423146487379,54.9828667286977,-3.77444482811614));
#36993=CARTESIAN_POINT('Ctrl Pts',(62.3973771232709,55.5925066752293,-3.65752819022485));
#36994=CARTESIAN_POINT('Ctrl Pts',(64.1888499135715,57.2383012421313,-3.54061155233356));
#36995=CARTESIAN_POINT('Ctrl Pts',(64.9955552343548,59.5333367141859,-3.42369491444227));
#36996=CARTESIAN_POINT('Ctrl Pts',(64.6278944275743,61.9380873251365,-3.30677827655098));
#36997=CARTESIAN_POINT('Ctrl Pts',(63.1721974290518,63.8871955171999,-3.18986163865969));
#36998=CARTESIAN_POINT('Ctrl Pts',(60.9709154413277,64.9224971427319,-3.0729450007684));
#36999=CARTESIAN_POINT('Ctrl Pts',(58.5410850419288,64.800457091261,-2.95602836287711));
#37000=CARTESIAN_POINT('Ctrl Pts',(57.1504834941423,63.9667473017145,-2.87808393761625));
#37001=CARTESIAN_POINT('Ctrl Pts',(56.5937019680037,63.4106813339364,-2.83911172498582));
#37002=CARTESIAN_POINT('Ctrl Pts',(56.1445283027442,63.3369355690004,-10.4826648250425));
#37003=CARTESIAN_POINT('Ctrl Pts',(55.5997855089079,62.7075436072762,-10.4436926124121));
#37004=CARTESIAN_POINT('Ctrl Pts',(54.8249540434462,61.1774399582876,-10.3657481871512));
#37005=CARTESIAN_POINT('Ctrl Pts',(54.8793645076338,58.60447478529,-10.24883154926));
#37006=CARTESIAN_POINT('Ctrl Pts',(56.1376808501272,56.3599042759194,-10.1319149113687));
#37007=CARTESIAN_POINT('Ctrl Pts',(58.3039662699263,54.9709051857687,-10.0149982734774));
#37008=CARTESIAN_POINT('Ctrl Pts',(60.8689858296667,54.7642653578555,-9.89808163558608));
#37009=CARTESIAN_POINT('Ctrl Pts',(63.2297107806181,55.7884527399271,-9.78116499769479));
#37010=CARTESIAN_POINT('Ctrl Pts',(64.831169445826,57.8027446189067,-9.6642483598035));
#37011=CARTESIAN_POINT('Ctrl Pts',(65.2968723721041,60.3335792537041,-9.54733172191222));
#37012=CARTESIAN_POINT('Ctrl Pts',(64.5173398680237,62.7859966304905,-9.43041508402093));
#37013=CARTESIAN_POINT('Ctrl Pts',(62.6758304956081,64.5834554024384,-9.31349844612963));
#37014=CARTESIAN_POINT('Ctrl Pts',(60.205263132424,65.3033953276082,-9.19658180823835));
#37015=CARTESIAN_POINT('Ctrl Pts',(57.6864406181491,64.7765653538453,-9.07966517034705));
#37016=CARTESIAN_POINT('Ctrl Pts',(55.7115103282802,63.1268179703927,-8.96274853245576));
#37017=CARTESIAN_POINT('Ctrl Pts',(54.7447564613263,60.7419901067622,-8.84583189456447));
#37018=CARTESIAN_POINT('Ctrl Pts',(55.0134521769933,58.1827288792718,-8.72891525667318));
#37019=CARTESIAN_POINT('Ctrl Pts',(56.4544300560118,56.0506873938616,-8.6119986187819));
#37020=CARTESIAN_POINT('Ctrl Pts',(58.7289322067895,54.8470867941934,-8.49508198089061));
#37021=CARTESIAN_POINT('Ctrl Pts',(61.3022482494153,54.8548764161609,-8.37816534299932));
#37022=CARTESIAN_POINT('Ctrl Pts',(63.5694203037008,56.0722332749569,-8.26124870510803));
#37023=CARTESIAN_POINT('Ctrl Pts',(64.9974608281321,58.2129524076025,-8.14433206721674));
#37024=CARTESIAN_POINT('Ctrl Pts',(65.250654372306,60.7738129689434,-8.02741542932545));
#37025=CARTESIAN_POINT('Ctrl Pts',(64.2694756368211,63.1527018302866,-7.91049879143416));
#37026=CARTESIAN_POINT('Ctrl Pts',(62.2845938431877,64.7905481022763,-7.79358215354287));
#37027=CARTESIAN_POINT('Ctrl Pts',(59.7626219966935,65.301924603536,-7.67666551565158));
#37028=CARTESIAN_POINT('Ctrl Pts',(57.2964708742581,64.5674491899606,-7.55974887776029));
#37029=CARTESIAN_POINT('Ctrl Pts',(55.4658552065881,62.7579816804522,-7.442832239869));
#37030=CARTESIAN_POINT('Ctrl Pts',(54.7012398189108,60.3028070774634,-7.32591560197771));
#37031=CARTESIAN_POINT('Ctrl Pts',(55.1821425126253,57.7706809218396,-7.20899896408643));
#37032=CARTESIAN_POINT('Ctrl Pts',(56.7959922829326,55.7750204186338,-7.09208232619513));
#37033=CARTESIAN_POINT('Ctrl Pts',(59.9512914978166,54.4027085123842,-6.93619347567342));
#37034=CARTESIAN_POINT('Ctrl Pts',(64.3799881642309,55.9075540482554,-6.74133241252127));
#37035=CARTESIAN_POINT('Ctrl Pts',(65.834479609045,61.37523011834,-6.50749913673868));
#37036=CARTESIAN_POINT('Ctrl Pts',(62.7388658113806,64.8816655541704,-6.31263807358654));
#37037=CARTESIAN_POINT('Ctrl Pts',(59.3187584788532,65.2585195543855,-6.15674922306482));
#37038=CARTESIAN_POINT('Ctrl Pts',(56.9266335796149,64.3285139675122,-6.03983258517353));
#37039=CARTESIAN_POINT('Ctrl Pts',(55.2511526541055,62.3700211957414,-5.92291594728224));
#37040=CARTESIAN_POINT('Ctrl Pts',(54.6947972197688,59.8594460319768,-5.80599930939095));
#37041=CARTESIAN_POINT('Ctrl Pts',(55.3843760081973,57.3795654934784,-5.68908267149966));
#37042=CARTESIAN_POINT('Ctrl Pts',(57.1596209351837,55.5168092181914,-5.57216603360837));
#37043=CARTESIAN_POINT('Ctrl Pts',(59.6023370896801,54.7074973445116,-5.45524939571708));
#37044=CARTESIAN_POINT('Ctrl Pts',(62.138664673409,55.1426278237003,-5.33833275782579));
#37045=CARTESIAN_POINT('Ctrl Pts',(64.1721578471653,56.7195645494213,-5.2214161199345));
#37046=CARTESIAN_POINT('Ctrl Pts',(65.2248497831894,59.0677454356388,-5.10449948204321));
#37047=CARTESIAN_POINT('Ctrl Pts',(65.0492249349093,61.6350658396978,-4.98758284415192));
#37048=CARTESIAN_POINT('Ctrl Pts',(63.6865889794253,63.8180111190031,-4.87066620626063));
#37049=CARTESIAN_POINT('Ctrl Pts',(61.4572740950116,65.1033792767411,-4.75374956836934));
#37050=CARTESIAN_POINT('Ctrl Pts',(58.8853714589078,65.189001781766,-4.63683293047805));
#37051=CARTESIAN_POINT('Ctrl Pts',(56.5755050441849,64.0547463443016,-4.51991629258676));
#37052=CARTESIAN_POINT('Ctrl Pts',(55.0706998168725,61.9672654489506,-4.40299965469547));
#37053=CARTESIAN_POINT('Ctrl Pts',(54.7247182017831,59.4173019594712,-4.28608301680418));
#37054=CARTESIAN_POINT('Ctrl Pts',(55.6188973320329,57.0043245192968,-4.16916637891289));
#37055=CARTESIAN_POINT('Ctrl Pts',(57.5430244185373,55.2955969820173,-4.0522497410216));
#37056=CARTESIAN_POINT('Ctrl Pts',(60.0447608866429,54.6928229271066,-3.93533310313032));
#37057=CARTESIAN_POINT('Ctrl Pts',(62.5359710846191,55.3377065632379,-3.81841646523902));
#37058=CARTESIAN_POINT('Ctrl Pts',(64.4310101049653,57.0786456054826,-3.70149982734774));
#37059=CARTESIAN_POINT('Ctrl Pts',(65.2843515953202,59.5063586001592,-3.58458318945645));
#37060=CARTESIAN_POINT('Ctrl Pts',(64.8954360734807,62.0501294386705,-3.46766655156516));
#37061=CARTESIAN_POINT('Ctrl Pts',(63.3555842661093,64.1119168678935,-3.35074991367387));
#37062=CARTESIAN_POINT('Ctrl Pts',(61.027044706866,65.2070699669712,-3.23383327578258));
#37063=CARTESIAN_POINT('Ctrl Pts',(58.4567442007043,65.0779746991923,-3.11691663789129));
#37064=CARTESIAN_POINT('Ctrl Pts',(56.9857510552448,64.1960675938266,-3.03897221263043));
#37065=CARTESIAN_POINT('Ctrl Pts',(56.3967816198432,63.6078550836889,-3.));
#37066=CARTESIAN_POINT('Ctrl Pts',(56.7766472160421,62.7898325810254,-10.));
#37067=CARTESIAN_POINT('Ctrl Pts',(56.6836916815798,62.7013634565378,-10.));
#37068=CARTESIAN_POINT('Ctrl Pts',(56.5950267759711,62.6087976402809,-10.));
#37069=CARTESIAN_POINT('Ctrl Pts',(56.5107708328057,62.5125537979556,-10.));
#37070=CARTESIAN_POINT('Ctrl Pts',(56.4249559337053,62.414529192119,-10.));
#37071=CARTESIAN_POINT('Ctrl Pts',(56.3437141378064,62.312688781189,-10.));
#37072=CARTESIAN_POINT('Ctrl Pts',(56.2671934014339,62.2074259581361,-10.));
#37073=CARTESIAN_POINT('Ctrl Pts',(56.1895731759036,62.1006506648932,-10.));
#37074=CARTESIAN_POINT('Ctrl Pts',(56.1168100786834,61.9903533919095,-10.));
#37075=CARTESIAN_POINT('Ctrl Pts',(56.0490902779739,61.8769019388278,-10.));
#37076=CARTESIAN_POINT('Ctrl Pts',(55.9815184148182,61.7636983265589,-10.));
#37077=CARTESIAN_POINT('Ctrl Pts',(55.9189673273988,61.6473536561778,-10.));
#37078=CARTESIAN_POINT('Ctrl Pts',(55.8616613826493,61.5281998896676,-10.));
#37079=CARTESIAN_POINT('Ctrl Pts',(55.8501068150877,61.5041749782664,-10.));
#37080=CARTESIAN_POINT('Ctrl Pts',(55.8387656287774,61.4800357739801,-10.));
#37081=CARTESIAN_POINT('Ctrl Pts',(55.8276398866233,61.4557848691785,-10.));
#37082=CARTESIAN_POINT('Ctrl Pts',(55.8174344409603,61.4335399449477,-10.));
#37083=CARTESIAN_POINT('Ctrl Pts',(55.8074083930678,61.4111965365112,-10.));
#37084=CARTESIAN_POINT('Ctrl Pts',(55.7975752706419,61.3887843305408,-10.));
#37085=CARTESIAN_POINT('Ctrl Pts',(55.7403627711479,61.2583823821857,-10.));
#37086=CARTESIAN_POINT('Ctrl Pts',(55.6896031187019,61.1254984802314,-10.));
#37087=CARTESIAN_POINT('Ctrl Pts',(55.645479920562,60.9906068936445,-10.));
#37088=CARTESIAN_POINT('Ctrl Pts',(55.6039768116069,60.863725333575,-10.));
#37089=CARTESIAN_POINT('Ctrl Pts',(55.5683448579499,60.7350665035816,-10.));
#37090=CARTESIAN_POINT('Ctrl Pts',(55.5385236905657,60.6050521672458,-10.));
#37091=CARTESIAN_POINT('Ctrl Pts',(55.5083230209178,60.4733832768034,-10.));
#37092=CARTESIAN_POINT('Ctrl Pts',(55.4840817318274,60.3403234669823,-10.));
#37093=CARTESIAN_POINT('Ctrl Pts',(55.4657841380372,60.2062855830499,-10.));
#37094=CARTESIAN_POINT('Ctrl Pts',(55.4495746406316,60.0875439191587,-10.));
#37095=CARTESIAN_POINT('Ctrl Pts',(55.4380302645887,59.9680339642758,-10.));
#37096=CARTESIAN_POINT('Ctrl Pts',(55.4311725531702,59.8480333617552,-10.));
#37097=CARTESIAN_POINT('Ctrl Pts',(55.429455905751,59.8179943717717,-10.));
#37098=CARTESIAN_POINT('Ctrl Pts',(55.4280330868615,59.7879246126589,-10.));
#37099=CARTESIAN_POINT('Ctrl Pts',(55.4269047438418,59.7578284042711,-10.));
#37100=CARTESIAN_POINT('Ctrl Pts',(55.42609738417,59.7362937605487,-10.));
#37101=CARTESIAN_POINT('Ctrl Pts',(55.4254408285579,59.7147438446829,-10.));
#37102=CARTESIAN_POINT('Ctrl Pts',(55.4249356300217,59.6932018270316,-10.));
#37103=CARTESIAN_POINT('Ctrl Pts',(55.4216903829473,59.5548222301979,-10.));
#37104=CARTESIAN_POINT('Ctrl Pts',(55.4246781614053,59.4165725060038,-10.));
#37105=CARTESIAN_POINT('Ctrl Pts',(55.4338328579124,59.2788933768414,-10.));
#37106=CARTESIAN_POINT('Ctrl Pts',(55.4430905358525,59.139665491367,-10.));
#37107=CARTESIAN_POINT('Ctrl Pts',(55.4586544403344,59.0010203364085,-10.));
#37108=CARTESIAN_POINT('Ctrl Pts',(55.4805057053574,58.8633952047768,-10.));
#37109=CARTESIAN_POINT('Ctrl Pts',(55.485322464481,58.8330579630784,-10.));
#37110=CARTESIAN_POINT('Ctrl Pts',(55.4904449293029,58.8027702410737,-10.));
#37111=CARTESIAN_POINT('Ctrl Pts',(55.4958732326893,58.7725366629253,-10.));
#37112=CARTESIAN_POINT('Ctrl Pts',(55.5203481259231,58.6362208484638,-10.));
#37113=CARTESIAN_POINT('Ctrl Pts',(55.551036175231,58.5010055472366,-10.));
#37114=CARTESIAN_POINT('Ctrl Pts',(55.5877252511952,58.3672429184636,-10.));
#37115=CARTESIAN_POINT('Ctrl Pts',(55.6089636892506,58.2898108973326,-10.));
#37116=CARTESIAN_POINT('Ctrl Pts',(55.6322140471996,58.2128656730071,-10.));
#37117=CARTESIAN_POINT('Ctrl Pts',(55.6574430346149,58.136476625185,-10.));
#37118=CARTESIAN_POINT('Ctrl Pts',(55.6711730594046,58.0949044644403,-10.));
#37119=CARTESIAN_POINT('Ctrl Pts',(55.6854891955254,58.0534970476954,-10.));
#37120=CARTESIAN_POINT('Ctrl Pts',(55.7003867655987,58.0122657515545,-10.));
#37121=CARTESIAN_POINT('Ctrl Pts',(55.7064544678847,57.9954724605263,-10.));
#37122=CARTESIAN_POINT('Ctrl Pts',(55.7126186291905,57.9787083878453,-10.));
#37123=CARTESIAN_POINT('Ctrl Pts',(55.7188789560352,57.9619743104561,-10.));
#37124=CARTESIAN_POINT('Ctrl Pts',(55.7254264843682,57.9444725332243,-10.));
#37125=CARTESIAN_POINT('Ctrl Pts',(55.7320759675732,57.9270122449326,-10.));
#37126=CARTESIAN_POINT('Ctrl Pts',(55.7388258598846,57.9095965174206,-10.));
#37127=CARTESIAN_POINT('Ctrl Pts',(55.7901008092709,57.7772995109641,-10.));
#37128=CARTESIAN_POINT('Ctrl Pts',(55.8471813531683,57.647531798479,-10.));
#37129=CARTESIAN_POINT('Ctrl Pts',(55.9097891914145,57.5206512582104,-10.));
#37130=CARTESIAN_POINT('Ctrl Pts',(55.9730108624179,57.3925267294244,-10.));
#37131=CARTESIAN_POINT('Ctrl Pts',(56.0418689194203,57.2673455178894,-10.));
#37132=CARTESIAN_POINT('Ctrl Pts',(56.1161301251681,57.1454790677295,-10.));
#37133=CARTESIAN_POINT('Ctrl Pts',(56.1904609341748,57.0234983950494,-10.));
#37134=CARTESIAN_POINT('Ctrl Pts',(56.2702052813482,56.9048379308472,-10.));
#37135=CARTESIAN_POINT('Ctrl Pts',(56.3551790628638,56.7898845039161,-10.));
#37136=CARTESIAN_POINT('Ctrl Pts',(56.3877839571239,56.7457762594309,-10.));
#37137=CARTESIAN_POINT('Ctrl Pts',(56.4211592802161,56.7022140122855,-10.));
#37138=CARTESIAN_POINT('Ctrl Pts',(56.4552964526868,56.6592205467288,-10.));
#37139=CARTESIAN_POINT('Ctrl Pts',(56.5184577159342,56.5796731970391,-10.));
#37140=CARTESIAN_POINT('Ctrl Pts',(56.5842264250915,56.502072454838,-10.));
#37141=CARTESIAN_POINT('Ctrl Pts',(56.6524865794293,56.4265028368199,-10.));
#37142=CARTESIAN_POINT('Ctrl Pts',(56.6665323443044,56.4109530172116,-10.));
#37143=CARTESIAN_POINT('Ctrl Pts',(56.6806836330993,56.3954892252364,-10.));
#37144=CARTESIAN_POINT('Ctrl Pts',(56.6949394878897,56.3801122433927,-10.));
#37145=CARTESIAN_POINT('Ctrl Pts',(56.7093516312862,56.3645666818957,-10.));
#37146=CARTESIAN_POINT('Ctrl Pts',(56.7238639781207,56.3491170502204,-10.));
#37147=CARTESIAN_POINT('Ctrl Pts',(56.7384737535074,56.3337654700224,-10.));
#37148=CARTESIAN_POINT('Ctrl Pts',(56.838104851128,56.229075647979,-10.));
#37149=CARTESIAN_POINT('Ctrl Pts',(56.9422847841482,56.1289203917598,-10.));
#37150=CARTESIAN_POINT('Ctrl Pts',(57.0506144838166,56.0334961807761,-10.));
#37151=CARTESIAN_POINT('Ctrl Pts',(57.1492676318998,55.9465957384623,-10.));
#37152=CARTESIAN_POINT('Ctrl Pts',(57.2513631973246,55.8636188452892,-10.));
#37153=CARTESIAN_POINT('Ctrl Pts',(57.3566308813066,55.7847333558599,-10.));
#37154=CARTESIAN_POINT('Ctrl Pts',(57.4121395358538,55.7431362843193,-10.));
#37155=CARTESIAN_POINT('Ctrl Pts',(57.4685306777316,55.7026771906877,-10.));
#37156=CARTESIAN_POINT('Ctrl Pts',(57.5257674930296,55.663383235408,-10.));
#37157=CARTESIAN_POINT('Ctrl Pts',(57.5474706288127,55.648483698415,-10.));
#37158=CARTESIAN_POINT('Ctrl Pts',(57.569295372594,55.6337517029334,-10.));
#37159=CARTESIAN_POINT('Ctrl Pts',(57.5912397820617,55.6191888039281,-10.));
#37160=CARTESIAN_POINT('Ctrl Pts',(57.6130039682011,55.6047455059597,-10.));
#37161=CARTESIAN_POINT('Ctrl Pts',(57.6348798477783,55.590472576591,-10.));
#37162=CARTESIAN_POINT('Ctrl Pts',(57.6568590240097,55.5763752246629,-10.));
#37163=CARTESIAN_POINT('Ctrl Pts',(57.782190594167,55.4959880785018,-10.));
#37164=CARTESIAN_POINT('Ctrl Pts',(57.910939943541,55.4212659189356,-10.));
#37165=CARTESIAN_POINT('Ctrl Pts',(58.0427132794917,55.3524362848689,-10.));
#37166=CARTESIAN_POINT('Ctrl Pts',(58.1526798140915,55.294997074717,-10.));
#37167=CARTESIAN_POINT('Ctrl Pts',(58.2647532542174,55.2416618501413,-10.));
#37168=CARTESIAN_POINT('Ctrl Pts',(58.3787241380444,55.1925827330161,-10.));
#37169=CARTESIAN_POINT('Ctrl Pts',(58.4767840492774,55.1503553350432,-10.));
#37170=CARTESIAN_POINT('Ctrl Pts',(58.5762489664664,55.1112788488363,-10.));
#37171=CARTESIAN_POINT('Ctrl Pts',(58.6769607112098,55.0753649997562,-10.));
#37172=CARTESIAN_POINT('Ctrl Pts',(64.2628730117989,60.0000978162778,-7.57968167058906));
#37173=CARTESIAN_POINT('Ctrl Pts',(64.2624542514066,59.5120606486749,-7.60701019445078));
#37174=CARTESIAN_POINT('Ctrl Pts',(64.1786779666622,59.0238810355797,-7.63433871831249));
#37175=CARTESIAN_POINT('Ctrl Pts',(64.0144041441174,58.56448844846,-7.66166724217421));
#37176=CARTESIAN_POINT('Ctrl Pts',(63.7801392283017,57.909365410104,-7.70063945480464));
#37177=CARTESIAN_POINT('Ctrl Pts',(63.3821699038818,57.3127853184214,-7.73961166743507));
#37178=CARTESIAN_POINT('Ctrl Pts',(62.8672751132997,56.8448674929813,-7.7785838800655));
#37179=CARTESIAN_POINT('Ctrl Pts',(62.3523803227176,56.3769496675411,-7.81755609269593));
#37180=CARTESIAN_POINT('Ctrl Pts',(61.7205600659731,56.0376941083434,-7.85652830532636));
#37181=CARTESIAN_POINT('Ctrl Pts',(61.0460813852798,55.8669809146618,-7.89550051795679));
#37182=CARTESIAN_POINT('Ctrl Pts',(60.3716027045864,55.6962677209802,-7.93447273058722));
#37183=CARTESIAN_POINT('Ctrl Pts',(59.6544655999441,55.6940968928147,-7.97344494321765));
#37184=CARTESIAN_POINT('Ctrl Pts',(58.9789655359289,55.8607224467775,-8.01241715584808));
#37185=CARTESIAN_POINT('Ctrl Pts',(58.3034654719138,56.0273480007403,-8.05138936847851));
#37186=CARTESIAN_POINT('Ctrl Pts',(57.6696024485259,56.3627699368315,-8.09036158110894));
#37187=CARTESIAN_POINT('Ctrl Pts',(57.1518835700849,56.8275617982647,-8.12933379373937));
#37188=CARTESIAN_POINT('Ctrl Pts',(56.634164691644,57.292353659698,-8.1683060063698));
#37189=CARTESIAN_POINT('Ctrl Pts',(56.2325899581502,57.8865154464734,-8.20727821900023));
#37190=CARTESIAN_POINT('Ctrl Pts',(55.9943622489868,58.5402064795222,-8.24625043163065));
#37191=CARTESIAN_POINT('Ctrl Pts',(55.7561345398234,59.193897512571,-8.28522264426108));
#37192=CARTESIAN_POINT('Ctrl Pts',(55.6812538549906,59.9071177918932,-8.32419485689152));
#37193=CARTESIAN_POINT('Ctrl Pts',(55.7785220088422,60.5960323436173,-8.36316706952195));
#37194=CARTESIAN_POINT('Ctrl Pts',(55.8757901626938,61.2849468953415,-8.40213928215238));
#37195=CARTESIAN_POINT('Ctrl Pts',(56.1452071552299,61.9495557194676,-8.44111149478281));
#37196=CARTESIAN_POINT('Ctrl Pts',(56.555104506362,62.5117376596622,-8.48008370741324));
#37197=CARTESIAN_POINT('Ctrl Pts',(56.9650018574941,63.0739195998569,-8.51905592004367));
#37198=CARTESIAN_POINT('Ctrl Pts',(57.5153795672222,63.5336746561201,-8.5580281326741));
#37199=CARTESIAN_POINT('Ctrl Pts',(58.1415437890979,63.836961224526,-8.59700034530453));
#37200=CARTESIAN_POINT('Ctrl Pts',(58.7677080109736,64.1402477929319,-8.63597255793496));
#37201=CARTESIAN_POINT('Ctrl Pts',(59.4696587449968,64.2870658734804,-8.67494477056539));
#37202=CARTESIAN_POINT('Ctrl Pts',(60.1648855557312,64.2601577306143,-8.71391698319582));
#37203=CARTESIAN_POINT('Ctrl Pts',(60.8601123664656,64.2332495877481,-8.75288919582625));
#37204=CARTESIAN_POINT('Ctrl Pts',(61.5486152539111,64.0326152214672,-8.79186140845667));
#37205=CARTESIAN_POINT('Ctrl Pts',(62.149464542133,63.6818382506294,-8.8308336210871));
#37206=CARTESIAN_POINT('Ctrl Pts',(62.750313830355,63.3310612797916,-8.86980583371753));
#37207=CARTESIAN_POINT('Ctrl Pts',(63.2635095193533,62.8301417043968,-8.90877804634796));
#37208=CARTESIAN_POINT('Ctrl Pts',(63.6287282393475,62.2379595110891,-8.94775025897839));
#37209=CARTESIAN_POINT('Ctrl Pts',(63.9939469593417,61.6457773177814,-8.98672247160882));
#37210=CARTESIAN_POINT('Ctrl Pts',(64.2111887103318,60.9623325065609,-9.02569468423925));
#37211=CARTESIAN_POINT('Ctrl Pts',(64.2549180523652,60.2679609524856,-9.06466689686968));
#37212=CARTESIAN_POINT('Ctrl Pts',(64.2605339012929,60.1787877436963,-9.06967182144281));
#37213=CARTESIAN_POINT('Ctrl Pts',(64.2632881070018,60.089434326242,-9.07467674601593));
#37214=CARTESIAN_POINT('Ctrl Pts',(64.2632129797225,60.0000762878951,-9.07968167058906));
#37215=CARTESIAN_POINT('Ctrl Pts',(61.322884965569,55.0755938055567,-10.));
#37216=CARTESIAN_POINT('Ctrl Pts',(62.1267766598728,55.2915500435982,-9.96102778736957));
#37217=CARTESIAN_POINT('Ctrl Pts',(63.6260271731292,56.1245140078271,-9.88308336210872));
#37218=CARTESIAN_POINT('Ctrl Pts',(65.0229772277616,58.2859118284941,-9.76616672421742));
#37219=CARTESIAN_POINT('Ctrl Pts',(65.2388166032808,60.8500628014955,-9.64925008632614));
#37220=CARTESIAN_POINT('Ctrl Pts',(64.2231822164303,63.2145072853594,-9.53233344843484));
#37221=CARTESIAN_POINT('Ctrl Pts',(62.2146698080337,64.8232034325914,-9.41541681054355));
#37222=CARTESIAN_POINT('Ctrl Pts',(59.6855379323249,65.2980445186201,-9.29850017265226));
#37223=CARTESIAN_POINT('Ctrl Pts',(57.2303209838473,64.5273621068898,-9.18158353476097));
#37224=CARTESIAN_POINT('Ctrl Pts',(55.4262302676069,62.6923526051193,-9.06466689686969));
#37225=CARTESIAN_POINT('Ctrl Pts',(54.6973796845391,60.2243982381535,-8.94775025897839));
#37226=CARTESIAN_POINT('Ctrl Pts',(55.2151175810578,57.7036915329656,-8.8308336210871));
#37227=CARTESIAN_POINT('Ctrl Pts',(56.8577278151099,55.7228209598733,-8.71391698319582));
#37228=CARTESIAN_POINT('Ctrl Pts',(59.2390517104132,54.7474680995942,-8.59700034530453));
#37229=CARTESIAN_POINT('Ctrl Pts',(61.799265976347,55.0069271683894,-8.48008370741324));
#37230=CARTESIAN_POINT('Ctrl Pts',(63.9364928560947,56.4402025290253,-8.36316706952195));
#37231=CARTESIAN_POINT('Ctrl Pts',(65.1482936744543,58.7103466239862,-8.24625043163065));
#37232=CARTESIAN_POINT('Ctrl Pts',(65.1497879909792,61.2836744162533,-8.12933379373937));
#37233=CARTESIAN_POINT('Ctrl Pts',(63.9406234579031,63.5552235763429,-8.01241715584808));
#37234=CARTESIAN_POINT('Ctrl Pts',(61.8050635087969,64.9909811652868,-7.89550051795679));
#37235=CARTESIAN_POINT('Ctrl Pts',(59.2451498198411,65.2534097530527,-7.7785838800655));
#37236=CARTESIAN_POINT('Ctrl Pts',(56.8627001620859,64.2808297817029,-7.66166724217421));
#37237=CARTESIAN_POINT('Ctrl Pts',(55.2177796069362,62.3018527370191,-7.54475060428292));
#37238=CARTESIAN_POINT('Ctrl Pts',(54.6971392652592,59.7817817811634,-7.42783396639163));
#37239=CARTESIAN_POINT('Ctrl Pts',(55.4230712085558,57.3129118130677,-7.31091732850034));
#37240=CARTESIAN_POINT('Ctrl Pts',(57.2251429658425,55.4759618040439,-7.19400069060905));
#37241=CARTESIAN_POINT('Ctrl Pts',(59.6792193933806,54.7020984074429,-7.07708405271776));
#37242=CARTESIAN_POINT('Ctrl Pts',(62.2094284211809,55.174716747074,-6.96016741482647));
#37243=CARTESIAN_POINT('Ctrl Pts',(64.2186721193591,56.7795408043723,-6.84325077693519));
#37244=CARTESIAN_POINT('Ctrl Pts',(65.2395171494002,59.1461424584795,-6.72633413904389));
#37245=CARTESIAN_POINT('Ctrl Pts',(65.0214070657763,61.7034072624198,-6.60941750115261));
#37246=CARTESIAN_POINT('Ctrl Pts',(63.1773281761085,64.6083211110609,-6.45352865063088));
#37247=CARTESIAN_POINT('Ctrl Pts',(58.6661397561353,65.8440762220129,-6.25866758747874));
#37248=CARTESIAN_POINT('Ctrl Pts',(54.3971986841152,62.1309686655549,-6.02483431169616));
#37249=CARTESIAN_POINT('Ctrl Pts',(54.9957816802558,57.4920452935348,-5.82997324854401));
#37250=CARTESIAN_POINT('Ctrl Pts',(57.6170719268681,55.2631467174745,-5.67408439802229));
#37251=CARTESIAN_POINT('Ctrl Pts',(60.1194257717932,54.6927078330755,-5.557167760131));
#37252=CARTESIAN_POINT('Ctrl Pts',(62.6046743394157,55.3756921094109,-5.44025112223971));
#37253=CARTESIAN_POINT('Ctrl Pts',(64.4724884051625,57.1431171033903,-5.32333448434842));
#37254=CARTESIAN_POINT('Ctrl Pts',(65.2912292886472,59.5834017558471,-5.20641784645713));
#37255=CARTESIAN_POINT('Ctrl Pts',(64.8649668293915,62.1210494825228,-5.08950120856584));
#37256=CARTESIAN_POINT('Ctrl Pts',(63.2955109480772,64.1603278329295,-4.97258457067455));
#37257=CARTESIAN_POINT('Ctrl Pts',(60.9510823128121,65.2214359708436,-4.85566793278326));
#37258=CARTESIAN_POINT('Ctrl Pts',(58.3831734117936,65.0550993752034,-4.73875129489197));
#37259=CARTESIAN_POINT('Ctrl Pts',(56.1953122098592,63.7003384596412,-4.62183465700068));
#37260=CARTESIAN_POINT('Ctrl Pts',(54.9019142936214,61.4756811820325,-4.50491801910939));
#37261=CARTESIAN_POINT('Ctrl Pts',(54.8070090801581,58.9041019292639,-4.3880013812181));
#37262=CARTESIAN_POINT('Ctrl Pts',(55.9329235426593,56.5901588022821,-4.27108474332681));
#37263=CARTESIAN_POINT('Ctrl Pts',(58.0149603175651,55.0778303762239,-4.15416810543552));
#37264=CARTESIAN_POINT('Ctrl Pts',(60.5636590493342,54.7226500811105,-4.03725146754424));
#37265=CARTESIAN_POINT('Ctrl Pts',(62.9798472108349,55.6081160860788,-3.92033482965294));
#37266=CARTESIAN_POINT('Ctrl Pts',(64.6955066712587,57.5260654357952,-3.80341819176166));
#37267=CARTESIAN_POINT('Ctrl Pts',(65.3073040613093,60.0256094769815,-3.68650155387036));
#37268=CARTESIAN_POINT('Ctrl Pts',(64.6714138007994,62.5191327746011,-3.56958491597908));
#37269=CARTESIAN_POINT('Ctrl Pts',(62.93732429588,64.4204364118546,-3.45266827808779));
#37270=CARTESIAN_POINT('Ctrl Pts',(60.5127057455321,65.2825431684356,-3.3357516401965));
#37271=CARTESIAN_POINT('Ctrl Pts',(57.967548471337,64.9027852181516,-3.2188350023052));
#37272=CARTESIAN_POINT('Ctrl Pts',(55.9002137011895,63.3704311318214,-3.10191836441392));
#37273=CARTESIAN_POINT('Ctrl Pts',(54.7966592622721,61.0457391111864,-2.98500172652262));
#37274=CARTESIAN_POINT('Ctrl Pts',(54.9164250447544,58.4751813736776,-2.86808508863134));
#37275=CARTESIAN_POINT('Ctrl Pts',(56.2311219607459,56.2631621903272,-2.75116845074005));
#37276=CARTESIAN_POINT('Ctrl Pts',(58.4321699151165,54.9295588396458,-2.63425181284876));
#37277=CARTESIAN_POINT('Ctrl Pts',(60.1446943002093,54.8355306649757,-2.5563073875879));
#37278=CARTESIAN_POINT('Ctrl Pts',(60.9621351249183,54.9925957821044,-2.51733517495747));
#37279=CARTESIAN_POINT('Ctrl Pts',(61.2505876634042,55.344718704462,-10.1608882750142));
#37280=CARTESIAN_POINT('Ctrl Pts',(62.0105456807492,55.5488726665669,-10.1219160623837));
#37281=CARTESIAN_POINT('Ctrl Pts',(63.4278602961771,56.3363141182708,-10.0439716371229));
#37282=CARTESIAN_POINT('Ctrl Pts',(64.7484652997752,58.3795888704878,-9.9270549992316));
#37283=CARTESIAN_POINT('Ctrl Pts',(64.9525087860393,60.8036058163318,-9.81013836134031));
#37284=CARTESIAN_POINT('Ctrl Pts',(63.9923800766032,63.0388304800668,-9.69322172344902));
#37285=CARTESIAN_POINT('Ctrl Pts',(62.0936353594806,64.5596093899918,-9.57630508555773));
#37286=CARTESIAN_POINT('Ctrl Pts',(59.7027236738805,65.0084998224335,-9.45938844766644));
#37287=CARTESIAN_POINT('Ctrl Pts',(57.3816873731722,64.2799361592295,-9.34247180977515));
#37288=CARTESIAN_POINT('Ctrl Pts',(55.6761924494909,62.5452121999497,-9.22555517188386));
#37289=CARTESIAN_POINT('Ctrl Pts',(54.9871744536915,60.2121345964527,-9.10863853399257));
#37290=CARTESIAN_POINT('Ctrl Pts',(55.4766173327892,57.8291876353675,-8.99172189610128));
#37291=CARTESIAN_POINT('Ctrl Pts',(57.0294568826766,55.9565740930069,-8.87480525820999));
#37292=CARTESIAN_POINT('Ctrl Pts',(59.2806384771057,55.0345254748142,-8.7578886203187));
#37293=CARTESIAN_POINT('Ctrl Pts',(61.7009338617999,55.2798047840805,-8.64097198242741));
#37294=CARTESIAN_POINT('Ctrl Pts',(63.7213586449621,56.634749870709,-8.52405534453613));
#37295=CARTESIAN_POINT('Ctrl Pts',(64.8669330474135,58.7808277786144,-8.40713870664483));
#37296=CARTESIAN_POINT('Ctrl Pts',(64.8683456976891,61.2135200191828,-8.29022206875355));
#37297=CARTESIAN_POINT('Ctrl Pts',(63.7252635042647,63.3609262036671,-8.17330543086225));
#37298=CARTESIAN_POINT('Ctrl Pts',(61.7064145519195,64.7182178617515,-8.05638879297097));
#37299=CARTESIAN_POINT('Ctrl Pts',(59.2864033172989,64.9663044020981,-7.93947215507967));
#37300=CARTESIAN_POINT('Ctrl Pts',(57.0341574847307,64.0468771310195,-7.82255551718839));
#37301=CARTESIAN_POINT('Ctrl Pts',(55.4791338756556,62.1760536333943,-7.7056388792971));
#37302=CARTESIAN_POINT('Ctrl Pts',(54.9869471736231,59.7937076771527,-7.58872224140581));
#37303=CARTESIAN_POINT('Ctrl Pts',(55.6732060369304,57.4597645112618,-7.47180560351452));
#37304=CARTESIAN_POINT('Ctrl Pts',(57.3767923402659,55.723206095854,-7.35488896562323));
#37305=CARTESIAN_POINT('Ctrl Pts',(59.696750450917,54.9916352925431,-7.23797232773193));
#37306=CARTESIAN_POINT('Ctrl Pts',(62.0886804209124,55.4384244544314,-7.12105568984065));
#37307=CARTESIAN_POINT('Ctrl Pts',(63.988116461924,56.9555428889342,-7.00413905194936));
#37308=CARTESIAN_POINT('Ctrl Pts',(64.9531710464455,59.1928068308866,-6.88722241405807));
#37309=CARTESIAN_POINT('Ctrl Pts',(64.7469809490875,61.6103139453392,-6.77030577616678));
#37310=CARTESIAN_POINT('Ctrl Pts',(63.0036832551942,64.3564706535303,-6.61441692564506));
#37311=CARTESIAN_POINT('Ctrl Pts',(58.7390368708552,65.5246902168091,-6.41955586249291));
#37312=CARTESIAN_POINT('Ctrl Pts',(54.7033987168066,62.0145085881277,-6.18572258671033));
#37313=CARTESIAN_POINT('Ctrl Pts',(55.2692684106804,57.6291081251099,-5.99086152355818));
#37314=CARTESIAN_POINT('Ctrl Pts',(57.747301898048,55.522021617402,-5.83497267303646));
#37315=CARTESIAN_POINT('Ctrl Pts',(60.1128990054194,54.9827579246979,-5.71805603514517));
#37316=CARTESIAN_POINT('Ctrl Pts',(62.462325660083,55.6284162642473,-5.60113939725389));
#37317=CARTESIAN_POINT('Ctrl Pts',(64.2280613732794,57.2992492928108,-5.48422275936259));
#37318=CARTESIAN_POINT('Ctrl Pts',(65.0020570532214,59.6061693659741,-5.36730612147131));
#37319=CARTESIAN_POINT('Ctrl Pts',(64.59909036542,62.0051315007363,-5.25038948358001));
#37320=CARTESIAN_POINT('Ctrl Pts',(63.1154071922693,63.9329607630251,-5.13347284568873));
#37321=CARTESIAN_POINT('Ctrl Pts',(60.8991044862114,64.9360780266961,-5.01655620779744));
#37322=CARTESIAN_POINT('Ctrl Pts',(58.4715349877719,64.7788319320662,-4.89963956990615));
#37323=CARTESIAN_POINT('Ctrl Pts',(56.4032431108567,63.498110378824,-4.78272293201486));
#37324=CARTESIAN_POINT('Ctrl Pts',(55.180530993009,61.3950333773531,-4.66580629412357));
#37325=CARTESIAN_POINT('Ctrl Pts',(55.0908124670305,58.9639941164336,-4.54888965623228));
#37326=CARTESIAN_POINT('Ctrl Pts',(56.1551943093676,56.7765108478657,-4.43197301834099));
#37327=CARTESIAN_POINT('Ctrl Pts',(58.1234451952872,55.3468330437716,-4.3150563804497));
#37328=CARTESIAN_POINT('Ctrl Pts',(60.5328543840245,55.0110637917852,-4.19813974255841));
#37329=CARTESIAN_POINT('Ctrl Pts',(62.8169948693132,55.8481379826623,-4.08122310466712));
#37330=CARTESIAN_POINT('Ctrl Pts',(64.4388914148573,57.6612690244515,-3.96430646677583));
#37331=CARTESIAN_POINT('Ctrl Pts',(65.017253319644,60.0242098873393,-3.84738982888454));
#37332=CARTESIAN_POINT('Ctrl Pts',(64.416115249615,62.3814590477548,-3.73047319099325));
#37333=CARTESIAN_POINT('Ctrl Pts',(62.7767958843382,64.178854085888,-3.61355655310196));
#37334=CARTESIAN_POINT('Ctrl Pts',(60.4846857413964,64.9938456402397,-3.49663991521067));
#37335=CARTESIAN_POINT('Ctrl Pts',(58.0786244651895,64.6348419323848,-3.37972327731938));
#37336=CARTESIAN_POINT('Ctrl Pts',(56.1242721012553,63.1862328951605,-3.26280663942809));
#37337=CARTESIAN_POINT('Ctrl Pts',(55.0810282795134,60.9885881732933,-3.1458900015368));
#37338=CARTESIAN_POINT('Ctrl Pts',(55.1942487136166,58.558514600559,-3.02897336364552));
#37339=CARTESIAN_POINT('Ctrl Pts',(56.437095814496,56.4673850058392,-2.91205672575423));
#37340=CARTESIAN_POINT('Ctrl Pts',(58.5178537714911,55.206664730347,-2.79514008786294));
#37341=CARTESIAN_POINT('Ctrl Pts',(60.1367865774548,55.1177753119051,-2.71719566260207));
#37342=CARTESIAN_POINT('Ctrl Pts',(60.9095532484437,55.2662566258098,-2.67822344997165));
#37343=CARTESIAN_POINT('Ctrl Pts',(61.1782903612393,55.6138436033673,-10.3217765500284));
#37344=CARTESIAN_POINT('Ctrl Pts',(61.8943147016256,55.8061952895356,-10.2828043373979));
#37345=CARTESIAN_POINT('Ctrl Pts',(63.229693419225,56.5481142287144,-10.2048599121371));
#37346=CARTESIAN_POINT('Ctrl Pts',(64.4739533717888,58.4732659124817,-10.0879432742458));
#37347=CARTESIAN_POINT('Ctrl Pts',(64.6662009687979,60.757148831168,-9.97102663635449));
#37348=CARTESIAN_POINT('Ctrl Pts',(63.761577936776,62.8631536747742,-9.85410999846319));
#37349=CARTESIAN_POINT('Ctrl Pts',(61.9726009109276,64.2960153473921,-9.7371933605719));
#37350=CARTESIAN_POINT('Ctrl Pts',(59.7199094154362,64.7189551262469,-9.62027672268062));
#37351=CARTESIAN_POINT('Ctrl Pts',(57.5330537624972,64.0325102115692,-9.50336008478933));
#37352=CARTESIAN_POINT('Ctrl Pts',(55.926154631375,62.3980717947801,-9.38644344689803));
#37353=CARTESIAN_POINT('Ctrl Pts',(55.276969222844,60.199870954752,-9.26952680900675));
#37354=CARTESIAN_POINT('Ctrl Pts',(55.7381170845207,57.9546837377693,-9.15261017111545));
#37355=CARTESIAN_POINT('Ctrl Pts',(57.2011859502433,56.1903272261406,-9.03569353322417));
#37356=CARTESIAN_POINT('Ctrl Pts',(59.3222252437981,55.3215828500341,-8.91877689533288));
#37357=CARTESIAN_POINT('Ctrl Pts',(61.6026017472529,55.5526823997716,-8.80186025744159));
#37358=CARTESIAN_POINT('Ctrl Pts',(63.5062244338295,56.8292972123926,-8.6849436195503));
#37359=CARTESIAN_POINT('Ctrl Pts',(64.5855724203726,58.8513089332426,-8.56802698165901));
#37360=CARTESIAN_POINT('Ctrl Pts',(64.586903404399,61.1433656221122,-8.45111034376773));
#37361=CARTESIAN_POINT('Ctrl Pts',(63.5099035506263,63.1666288309912,-8.33419370587642));
#37362=CARTESIAN_POINT('Ctrl Pts',(61.607765595042,64.4454545582162,-8.21727706798515));
#37363=CARTESIAN_POINT('Ctrl Pts',(59.3276568147568,64.6791990511435,-8.10036043009385));
#37364=CARTESIAN_POINT('Ctrl Pts',(57.2056148073754,63.8129244803361,-7.98344379220256));
#37365=CARTESIAN_POINT('Ctrl Pts',(55.740488144375,62.0502545297695,-7.86652715431127));
#37366=CARTESIAN_POINT('Ctrl Pts',(55.2767550819871,59.8056335731419,-7.74961051641998));
#37367=CARTESIAN_POINT('Ctrl Pts',(55.9233408653051,57.6066172094559,-7.63269387852869));
#37368=CARTESIAN_POINT('Ctrl Pts',(57.5284417146894,55.9704503876641,-7.51577724063741));
#37369=CARTESIAN_POINT('Ctrl Pts',(59.7142815084534,55.2811721776433,-7.39886060274611));
#37370=CARTESIAN_POINT('Ctrl Pts',(61.9679324206439,55.7021321617888,-7.28194396485482));
#37371=CARTESIAN_POINT('Ctrl Pts',(63.757560804489,57.1315449734963,-7.16502732696353));
#37372=CARTESIAN_POINT('Ctrl Pts',(64.6668249434908,59.2394712032937,-7.04811068907225));
#37373=CARTESIAN_POINT('Ctrl Pts',(64.4725548323986,61.5172206282585,-6.93119405118096));
#37374=CARTESIAN_POINT('Ctrl Pts',(62.8300383342798,64.1046201959996,-6.77530520065924));
#37375=CARTESIAN_POINT('Ctrl Pts',(58.8119339855751,65.2053042116052,-6.58044413750709));
#37376=CARTESIAN_POINT('Ctrl Pts',(55.0095987494979,61.8980485107005,-6.34661086172451));
#37377=CARTESIAN_POINT('Ctrl Pts',(55.5427551411051,57.7661709566851,-6.15174979857236));
#37378=CARTESIAN_POINT('Ctrl Pts',(57.8775318692278,55.7808965173295,-5.99586094805064));
#37379=CARTESIAN_POINT('Ctrl Pts',(60.1063722390457,55.2728080163204,-5.87894431015935));
#37380=CARTESIAN_POINT('Ctrl Pts',(62.3199769807503,55.8811404190837,-5.76202767226806));
#37381=CARTESIAN_POINT('Ctrl Pts',(63.9836343413963,57.4553814822313,-5.64511103437677));
#37382=CARTESIAN_POINT('Ctrl Pts',(64.7128848177956,59.628936976101,-5.52819439648548));
#37383=CARTESIAN_POINT('Ctrl Pts',(64.3332139014486,61.8892135189497,-5.41127775859419));
#37384=CARTESIAN_POINT('Ctrl Pts',(62.9353034364615,63.7055936931205,-5.29436112070291));
#37385=CARTESIAN_POINT('Ctrl Pts',(60.8471266596107,64.6507200825485,-5.17744448281161));
#37386=CARTESIAN_POINT('Ctrl Pts',(58.5598965637503,64.502564488929,-5.06052784492033));
#37387=CARTESIAN_POINT('Ctrl Pts',(56.6111740118541,63.2958822980069,-4.94361120702903));
#37388=CARTESIAN_POINT('Ctrl Pts',(55.4591476923966,61.3143855726739,-4.82669456913774));
#37389=CARTESIAN_POINT('Ctrl Pts',(55.374615853903,59.0238863036033,-4.70977793124645));
#37390=CARTESIAN_POINT('Ctrl Pts',(56.3774650760759,56.9628628934493,-4.59286129335516));
#37391=CARTESIAN_POINT('Ctrl Pts',(58.2319300730093,55.6158357113192,-4.47594465546387));
#37392=CARTESIAN_POINT('Ctrl Pts',(60.5020497187147,55.29947750246,-4.35902801757259));
#37393=CARTESIAN_POINT('Ctrl Pts',(62.6541425277914,56.0881598792458,-4.2421113796813));
#37394=CARTESIAN_POINT('Ctrl Pts',(64.1822761584559,57.7964726131078,-4.12519474179001));
#37395=CARTESIAN_POINT('Ctrl Pts',(64.7272025779786,60.0228102976971,-4.00827810389872));
#37396=CARTESIAN_POINT('Ctrl Pts',(64.1608166984306,62.2437853209086,-3.89136146600743));
#37397=CARTESIAN_POINT('Ctrl Pts',(62.6162674727963,63.9372717599215,-3.77444482811614));
#37398=CARTESIAN_POINT('Ctrl Pts',(60.4566657372606,64.7051481120438,-3.65752819022485));
#37399=CARTESIAN_POINT('Ctrl Pts',(58.1897004590421,64.366898646618,-3.54061155233356));
#37400=CARTESIAN_POINT('Ctrl Pts',(56.348330501321,63.0020346584995,-3.42369491444227));
#37401=CARTESIAN_POINT('Ctrl Pts',(55.3653972967547,60.9314372354001,-3.30677827655098));
#37402=CARTESIAN_POINT('Ctrl Pts',(55.4720723824788,58.6418478274405,-3.18986163865969));
#37403=CARTESIAN_POINT('Ctrl Pts',(56.6430696682462,56.6716078213511,-3.0729450007684));
#37404=CARTESIAN_POINT('Ctrl Pts',(58.6035376278658,55.4837706210482,-2.95602836287711));
#37405=CARTESIAN_POINT('Ctrl Pts',(60.1288788547003,55.4000199588346,-2.87808393761625));
#37406=CARTESIAN_POINT('Ctrl Pts',(60.8569713719691,55.5399174695151,-2.83911172498582));
#37407=CARTESIAN_POINT('Ctrl Pts',(61.1059930590745,55.8829685022727,-10.4826648250425));
#37408=CARTESIAN_POINT('Ctrl Pts',(61.778083722502,56.0635179125043,-10.4436926124121));
#37409=CARTESIAN_POINT('Ctrl Pts',(63.031526542273,56.759914339158,-10.3657481871512));
#37410=CARTESIAN_POINT('Ctrl Pts',(64.1994414438023,58.5669429544754,-10.24883154926));
#37411=CARTESIAN_POINT('Ctrl Pts',(64.3798931515564,60.7106918460042,-10.1319149113687));
#37412=CARTESIAN_POINT('Ctrl Pts',(63.5307757969489,62.6874768694816,-10.0149982734774));
#37413=CARTESIAN_POINT('Ctrl Pts',(61.8515664623745,64.0324213047925,-9.89808163558608));
#37414=CARTESIAN_POINT('Ctrl Pts',(59.7370951569918,64.4294104300603,-9.78116499769479));
#37415=CARTESIAN_POINT('Ctrl Pts',(57.6844201518221,63.7850842639089,-9.6642483598035));
#37416=CARTESIAN_POINT('Ctrl Pts',(56.176116813259,62.2509313896104,-9.54733172191221));
#37417=CARTESIAN_POINT('Ctrl Pts',(55.5667639919965,60.1876073130513,-9.43041508402093));
#37418=CARTESIAN_POINT('Ctrl Pts',(55.9996168362521,58.0801798401711,-9.31349844612963));
#37419=CARTESIAN_POINT('Ctrl Pts',(57.37291501781,56.4240803592743,-9.19658180823834));
#37420=CARTESIAN_POINT('Ctrl Pts',(59.3638120104906,55.608640225254,-9.07966517034706));
#37421=CARTESIAN_POINT('Ctrl Pts',(61.5042696327058,55.8255600154627,-8.96274853245576));
#37422=CARTESIAN_POINT('Ctrl Pts',(63.2910902226969,57.0238445540762,-8.84583189456448));
#37423=CARTESIAN_POINT('Ctrl Pts',(64.3042117933318,58.9217900878708,-8.72891525667318));
#37424=CARTESIAN_POINT('Ctrl Pts',(64.3054611111089,61.0732112250417,-8.6119986187819));
#37425=CARTESIAN_POINT('Ctrl Pts',(63.2945435969878,62.9723314583153,-8.4950819808906));
#37426=CARTESIAN_POINT('Ctrl Pts',(61.5091166381646,64.1726912546809,-8.37816534299932));
#37427=CARTESIAN_POINT('Ctrl Pts',(59.3689103122146,64.392093700189,-8.26124870510803));
#37428=CARTESIAN_POINT('Ctrl Pts',(57.3770721300201,63.5789718296528,-8.14433206721674));
#37429=CARTESIAN_POINT('Ctrl Pts',(56.0018424130945,61.9244554261448,-8.02741542932545));
#37430=CARTESIAN_POINT('Ctrl Pts',(55.5665629903511,59.8175594691311,-7.91049879143416));
#37431=CARTESIAN_POINT('Ctrl Pts',(56.1734756936798,57.75346990765,-7.79358215354287));
#37432=CARTESIAN_POINT('Ctrl Pts',(57.6800910891129,56.2176946794742,-7.67666551565158));
#37433=CARTESIAN_POINT('Ctrl Pts',(59.7318125659897,55.5707090627434,-7.55974887776029));
#37434=CARTESIAN_POINT('Ctrl Pts',(61.8471844203754,55.9658398691463,-7.442832239869));
#37435=CARTESIAN_POINT('Ctrl Pts',(63.5270051470539,57.3075470580582,-7.32591560197771));
#37436=CARTESIAN_POINT('Ctrl Pts',(64.380478840536,59.2861355757008,-7.20899896408642));
#37437=CARTESIAN_POINT('Ctrl Pts',(64.1981287157098,61.4241273111779,-7.09208232619514));
#37438=CARTESIAN_POINT('Ctrl Pts',(62.6563934133655,63.8527697384689,-6.93619347567341));
#37439=CARTESIAN_POINT('Ctrl Pts',(58.884831100295,64.8859182064014,-6.74133241252127));
#37440=CARTESIAN_POINT('Ctrl Pts',(55.3157987821893,61.7815884332733,-6.50749913673868));
#37441=CARTESIAN_POINT('Ctrl Pts',(55.8162418715298,57.9032337882602,-6.31263807358654));
#37442=CARTESIAN_POINT('Ctrl Pts',(58.0077618404077,56.0397714172571,-6.15674922306482));
#37443=CARTESIAN_POINT('Ctrl Pts',(60.099845472672,55.5628581079429,-6.03983258517353));
#37444=CARTESIAN_POINT('Ctrl Pts',(62.1776283014177,56.1338645739201,-5.92291594728224));
#37445=CARTESIAN_POINT('Ctrl Pts',(63.7392073095132,57.6115136716518,-5.80599930939095));
#37446=CARTESIAN_POINT('Ctrl Pts',(64.4237125823697,59.651704586228,-5.68908267149966));
#37447=CARTESIAN_POINT('Ctrl Pts',(64.0673374374772,61.7732955371631,-5.57216603360837));
#37448=CARTESIAN_POINT('Ctrl Pts',(62.7551996806536,63.4782266232161,-5.45524939571708));
#37449=CARTESIAN_POINT('Ctrl Pts',(60.79514883301,64.3653621384009,-5.33833275782579));
#37450=CARTESIAN_POINT('Ctrl Pts',(58.6482581397286,64.2262970457918,-5.2214161199345));
#37451=CARTESIAN_POINT('Ctrl Pts',(56.8191049128515,63.0936542171897,-5.10449948204321));
#37452=CARTESIAN_POINT('Ctrl Pts',(55.7377643917842,61.2337377679946,-4.98758284415192));
#37453=CARTESIAN_POINT('Ctrl Pts',(55.6584192407754,59.0837784907731,-4.87066620626063));
#37454=CARTESIAN_POINT('Ctrl Pts',(56.5997358427842,57.1492149390329,-4.75374956836934));
#37455=CARTESIAN_POINT('Ctrl Pts',(58.3404149507315,55.8848383788669,-4.63683293047805));
#37456=CARTESIAN_POINT('Ctrl Pts',(60.4712450534049,55.5878912131347,-4.51991629258676));
#37457=CARTESIAN_POINT('Ctrl Pts',(62.4912901862697,56.3281817758293,-4.40299965469547));
#37458=CARTESIAN_POINT('Ctrl Pts',(63.9256609020545,57.9316762017641,-4.28608301680419));
#37459=CARTESIAN_POINT('Ctrl Pts',(64.4371518363133,60.0214107080549,-4.16916637891289));
#37460=CARTESIAN_POINT('Ctrl Pts',(63.9055181472461,62.1061115940624,-4.0522497410216));
#37461=CARTESIAN_POINT('Ctrl Pts',(62.4557390612544,63.6956894339549,-3.93533310313032));
#37462=CARTESIAN_POINT('Ctrl Pts',(60.4286457331249,64.416450583848,-3.81841646523903));
#37463=CARTESIAN_POINT('Ctrl Pts',(58.3007764528946,64.0989553608512,-3.70149982734773));
#37464=CARTESIAN_POINT('Ctrl Pts',(56.5723889013868,62.8178364218386,-3.58458318945645));
#37465=CARTESIAN_POINT('Ctrl Pts',(55.649766313996,60.8742862975069,-3.46766655156516));
#37466=CARTESIAN_POINT('Ctrl Pts',(55.7498960513411,58.725181054322,-3.35074991367387));
#37467=CARTESIAN_POINT('Ctrl Pts',(56.8490435219964,56.8758306368631,-3.23383327578258));
#37468=CARTESIAN_POINT('Ctrl Pts',(58.6892214842404,55.7608765117494,-3.11691663789129));
#37469=CARTESIAN_POINT('Ctrl Pts',(60.1209711319459,55.6822646057641,-3.03897221263043));
#37470=CARTESIAN_POINT('Ctrl Pts',(60.8043894954945,55.8135783132205,-3.));
#37471=CARTESIAN_POINT('Ctrl Pts',(64.2626696975502,60.0000007546914,-8.67031832941094));
#37472=CARTESIAN_POINT('Ctrl Pts',(64.2626718116082,60.3472087819798,-8.65087842586793));
#37473=CARTESIAN_POINT('Ctrl Pts',(64.2207061566376,60.6944163006858,-8.63143852232491));
#37474=CARTESIAN_POINT('Ctrl Pts',(64.1367666391259,61.0311610743922,-8.6119986187819));
#37475=CARTESIAN_POINT('Ctrl Pts',(63.9684886064019,61.7062513027996,-8.57302640615147));
#37476=CARTESIAN_POINT('Ctrl Pts',(63.6315161016949,62.3392913805575,-8.53405419352104));
#37477=CARTESIAN_POINT('Ctrl Pts',(63.1654586895375,62.8558713854973,-8.49508198089061));
#37478=CARTESIAN_POINT('Ctrl Pts',(62.6994012773801,63.3724513904372,-8.45610976826018));
#37479=CARTESIAN_POINT('Ctrl Pts',(62.1042589577723,63.772571322559,-8.41713755562975));
#37480=CARTESIAN_POINT('Ctrl Pts',(61.4499867436435,64.0091983628713,-8.37816534299932));
#37481=CARTESIAN_POINT('Ctrl Pts',(60.7957145295146,64.2458254031836,-8.33919313036889));
#37482=CARTESIAN_POINT('Ctrl Pts',(60.0823124208646,64.3189595516863,-8.30022091773846));
#37483=CARTESIAN_POINT('Ctrl Pts',(59.3936383361739,64.2200063141816,-8.26124870510803));
#37484=CARTESIAN_POINT('Ctrl Pts',(58.7049642514831,64.1210530766769,-8.2222764924776));
#37485=CARTESIAN_POINT('Ctrl Pts',(58.0410181907516,63.8500124531648,-8.18330427984717));
#37486=CARTESIAN_POINT('Ctrl Pts',(57.4798402075649,63.4387394074908,-8.14433206721674));
#37487=CARTESIAN_POINT('Ctrl Pts',(56.9186622243782,63.0274663618168,-8.10535985458631));
#37488=CARTESIAN_POINT('Ctrl Pts',(56.4602523187364,62.4759608939808,-8.06638764195588));
#37489=CARTESIAN_POINT('Ctrl Pts',(56.1585007954582,61.8490588338939,-8.02741542932545));
#37490=CARTESIAN_POINT('Ctrl Pts',(55.85674927218,61.2221567738069,-7.98844321669502));
#37491=CARTESIAN_POINT('Ctrl Pts',(55.7116561312655,60.519858121469,-7.94947100406459));
#37492=CARTESIAN_POINT('Ctrl Pts',(55.7402616780298,59.8246938683866,-7.91049879143416));
#37493=CARTESIAN_POINT('Ctrl Pts',(55.768867224794,59.1295296153041,-7.87152657880373));
#37494=CARTESIAN_POINT('Ctrl Pts',(55.9711714592369,58.441499761477,-7.8325543661733));
#37495=CARTESIAN_POINT('Ctrl Pts',(56.3234261423639,57.8415222965342,-7.79358215354287));
#37496=CARTESIAN_POINT('Ctrl Pts',(56.6756808254908,57.2415448315914,-7.75460994091244));
#37497=CARTESIAN_POINT('Ctrl Pts',(57.1778859573018,56.7296197555328,-7.71563772828201));
#37498=CARTESIAN_POINT('Ctrl Pts',(57.7709421026868,56.3658262813817,-7.67666551565158));
#37499=CARTESIAN_POINT('Ctrl Pts',(58.3639982480718,56.0020328072306,-7.63769330302115));
#37500=CARTESIAN_POINT('Ctrl Pts',(59.0479054070308,55.786370934987,-7.59872109039072));
#37501=CARTESIAN_POINT('Ctrl Pts',(59.7424209622412,55.7443951332657,-7.55974887776029));
#37502=CARTESIAN_POINT('Ctrl Pts',(60.4369365174516,55.7024193315444,-7.52077666512986));
#37503=CARTESIAN_POINT('Ctrl Pts',(61.1420604689135,55.8341296003453,-7.48180445249943));
#37504=CARTESIAN_POINT('Ctrl Pts',(61.7745925657575,56.1236025995645,-7.442832239869));
#37505=CARTESIAN_POINT('Ctrl Pts',(62.4071246626015,56.4130755987836,-7.40386002723857));
#37506=CARTESIAN_POINT('Ctrl Pts',(62.9670649048277,56.8603113284209,-7.36488781460814));
#37507=CARTESIAN_POINT('Ctrl Pts',(63.3892806415212,57.41369394618,-7.32591560197771));
#37508=CARTESIAN_POINT('Ctrl Pts',(63.8114963782146,57.9670765639391,-7.28694338934728));
#37509=CARTESIAN_POINT('Ctrl Pts',(64.0959876093753,58.6266060698199,-7.24797117671685));
#37510=CARTESIAN_POINT('Ctrl Pts',(64.2078415374846,59.3127027786732,-7.20899896408642));
#37511=CARTESIAN_POINT('Ctrl Pts',(64.2448472281053,59.5396906276728,-7.1961054191946));
#37512=CARTESIAN_POINT('Ctrl Pts',(64.2629569487826,59.7695863827851,-7.18321187430277));
#37513=CARTESIAN_POINT('Ctrl Pts',(64.2625441198806,59.9995177541909,-7.17031832941094));
#37514=CARTESIAN_POINT('Ctrl Pts',(61.322884965569,55.0755938055567,-10.));
#37515=CARTESIAN_POINT('Ctrl Pts',(61.4613623534188,55.1251023381749,-10.));
#37516=CARTESIAN_POINT('Ctrl Pts',(61.5973330701288,55.1806177929913,-10.));
#37517=CARTESIAN_POINT('Ctrl Pts',(61.7304726735596,55.2418650003063,-10.));
#37518=CARTESIAN_POINT('Ctrl Pts',(61.8646634500372,55.3035957708277,-10.));
#37519=CARTESIAN_POINT('Ctrl Pts',(61.9959788862617,55.3711496178193,-10.));
#37520=CARTESIAN_POINT('Ctrl Pts',(62.1240611590226,55.4442909142459,-10.));
#37521=CARTESIAN_POINT('Ctrl Pts',(62.2511464727888,55.5168628979036,-10.));
#37522=CARTESIAN_POINT('Ctrl Pts',(62.3750493162488,55.5949362272756,-10.));
#37523=CARTESIAN_POINT('Ctrl Pts',(62.4953860692366,55.6783183026231,-10.));
#37524=CARTESIAN_POINT('Ctrl Pts',(62.6141471692546,55.7606085983489,-10.));
#37525=CARTESIAN_POINT('Ctrl Pts',(62.7294354281262,55.8480700429306,-10.));
#37526=CARTESIAN_POINT('Ctrl Pts',(62.8408412017621,55.9405463957895,-10.));
#37527=CARTESIAN_POINT('Ctrl Pts',(62.8725488687966,55.9668664805511,-10.));
#37528=CARTESIAN_POINT('Ctrl Pts',(62.9039417533278,55.9935929543698,-10.));
#37529=CARTESIAN_POINT('Ctrl Pts',(62.9350097121908,56.020722563045,-10.));
#37530=CARTESIAN_POINT('Ctrl Pts',(62.9507462780503,56.0344642728092,-10.));
#37531=CARTESIAN_POINT('Ctrl Pts',(62.9663994747131,56.048309414399,-10.));
#37532=CARTESIAN_POINT('Ctrl Pts',(62.9819679512752,56.0622575780891,-10.));
#37533=CARTESIAN_POINT('Ctrl Pts',(62.9973223809954,56.076013972188,-10.));
#37534=CARTESIAN_POINT('Ctrl Pts',(63.0125883643442,56.0898652018544,-10.));
#37535=CARTESIAN_POINT('Ctrl Pts',(63.027759913392,56.1038060602825,-10.));
#37536=CARTESIAN_POINT('Ctrl Pts',(63.1388330059994,56.2058690898602,-10.));
#37537=CARTESIAN_POINT('Ctrl Pts',(63.2449336421493,56.3128090269311,-10.));
#37538=CARTESIAN_POINT('Ctrl Pts',(63.34567176205,56.4243836549341,-10.));
#37539=CARTESIAN_POINT('Ctrl Pts',(63.4421342874271,56.5312227581038,-10.));
#37540=CARTESIAN_POINT('Ctrl Pts',(63.533679969545,56.642312423058,-10.));
#37541=CARTESIAN_POINT('Ctrl Pts',(63.6201051195375,56.7572698794827,-10.));
#37542=CARTESIAN_POINT('Ctrl Pts',(63.706379868931,56.8720272822158,-10.));
#37543=CARTESIAN_POINT('Ctrl Pts',(63.7875521943201,56.9906397862812,-10.));
#37544=CARTESIAN_POINT('Ctrl Pts',(63.8633716991881,57.1127463357118,-10.));
#37545=CARTESIAN_POINT('Ctrl Pts',(63.9290488453146,57.2185187184769,-10.));
#37546=CARTESIAN_POINT('Ctrl Pts',(63.9907088543825,57.3269134655884,-10.));
#37547=CARTESIAN_POINT('Ctrl Pts',(64.0481572658614,57.4377013353837,-10.));
#37548=CARTESIAN_POINT('Ctrl Pts',(64.0632545108638,57.466816006626,-10.));
#37549=CARTESIAN_POINT('Ctrl Pts',(64.0780607290788,57.4960959612206,-10.));
#37550=CARTESIAN_POINT('Ctrl Pts',(64.0925720318306,57.5255370454525,-10.));
#37551=CARTESIAN_POINT('Ctrl Pts',(64.1048378291218,57.5504223626014,-10.));
#37552=CARTESIAN_POINT('Ctrl Pts',(64.1168955869776,57.5754286797017,-10.));
#37553=CARTESIAN_POINT('Ctrl Pts',(64.1287279624461,57.6005212096262,-10.));
#37554=CARTESIAN_POINT('Ctrl Pts',(64.1887507851646,57.7278096378235,-10.));
#37555=CARTESIAN_POINT('Ctrl Pts',(64.2430415539658,57.8574379049107,-10.));
#37556=CARTESIAN_POINT('Ctrl Pts',(64.2914122956066,57.9890469751202,-10.));
#37557=CARTESIAN_POINT('Ctrl Pts',(64.3393952774439,58.1196010127734,-10.));
#37558=CARTESIAN_POINT('Ctrl Pts',(64.381552967519,58.2521049552159,-10.));
#37559=CARTESIAN_POINT('Ctrl Pts',(64.4176523161959,58.3862204475955,-10.));
#37560=CARTESIAN_POINT('Ctrl Pts',(64.426387292412,58.4186724357637,-10.));
#37561=CARTESIAN_POINT('Ctrl Pts',(64.4347673173568,58.4512188074512,-10.));
#37562=CARTESIAN_POINT('Ctrl Pts',(64.442788628001,58.4838548036334,-10.));
#37563=CARTESIAN_POINT('Ctrl Pts',(64.4762031615177,58.6198072229625,-10.));
#37564=CARTESIAN_POINT('Ctrl Pts',(64.5033968549748,58.7573155296226,-10.));
#37565=CARTESIAN_POINT('Ctrl Pts',(64.5243233337952,58.8959463037013,-10.));
#37566=CARTESIAN_POINT('Ctrl Pts',(64.5357566990593,58.9716884431454,-10.));
#37567=CARTESIAN_POINT('Ctrl Pts',(64.5453183547014,59.0477655330272,-10.));
#37568=CARTESIAN_POINT('Ctrl Pts',(64.5529943308661,59.1241052349256,-10.));
#37569=CARTESIAN_POINT('Ctrl Pts',(64.5578649402481,59.1725447897545,-10.));
#37570=CARTESIAN_POINT('Ctrl Pts',(64.5619762400323,59.2210900501072,-10.));
#37571=CARTESIAN_POINT('Ctrl Pts',(64.5653237282423,59.2697221490712,-10.));
#37572=CARTESIAN_POINT('Ctrl Pts',(64.5666136562909,59.2884621429351,-10.));
#37573=CARTESIAN_POINT('Ctrl Pts',(64.5677902998301,59.3072175547175,-10.));
#37574=CARTESIAN_POINT('Ctrl Pts',(64.5688529128554,59.3259790228935,-10.));
#37575=CARTESIAN_POINT('Ctrl Pts',(64.5766120890547,59.4629748378002,-10.));
#37576=CARTESIAN_POINT('Ctrl Pts',(64.57828067089,59.5999983793925,-10.));
#37577=CARTESIAN_POINT('Ctrl Pts',(64.5738795531211,59.736643965364,-10.));
#37578=CARTESIAN_POINT('Ctrl Pts',(64.5694908520678,59.8729040380465,-10.));
#37579=CARTESIAN_POINT('Ctrl Pts',(64.559066518732,60.0087890791135,-10.));
#37580=CARTESIAN_POINT('Ctrl Pts',(64.5425762131985,60.1438893634685,-10.));
#37581=CARTESIAN_POINT('Ctrl Pts',(64.5263562494215,60.2767748163219,-10.));
#37582=CARTESIAN_POINT('Ctrl Pts',(64.504267351696,60.4089017135858,-10.));
#37583=CARTESIAN_POINT('Ctrl Pts',(64.4762339793328,60.5398620574008,-10.));
#37584=CARTESIAN_POINT('Ctrl Pts',(64.4633631283279,60.599989360351,-10.));
#37585=CARTESIAN_POINT('Ctrl Pts',(64.4492385683906,60.6598704422786,-10.));
#37586=CARTESIAN_POINT('Ctrl Pts',(64.4338497987549,60.7194639158437,-10.));
#37587=CARTESIAN_POINT('Ctrl Pts',(64.4113888332848,60.8064446806276,-10.));
#37588=CARTESIAN_POINT('Ctrl Pts',(64.3862349033453,60.8928130777696,-10.));
#37589=CARTESIAN_POINT('Ctrl Pts',(64.3584258263513,60.9784471471686,-10.));
#37590=CARTESIAN_POINT('Ctrl Pts',(64.3510564629766,61.001140046138,-10.));
#37591=CARTESIAN_POINT('Ctrl Pts',(64.343500606592,61.0237813381838,-10.));
#37592=CARTESIAN_POINT('Ctrl Pts',(64.3357588821457,61.0463686652349,-10.));
#37593=CARTESIAN_POINT('Ctrl Pts',(64.328750676373,61.0668158714004,-10.));
#37594=CARTESIAN_POINT('Ctrl Pts',(64.3215927040502,61.0872113276609,-10.));
#37595=CARTESIAN_POINT('Ctrl Pts',(64.3142878250982,61.1075478141133,-10.));
#37596=CARTESIAN_POINT('Ctrl Pts',(64.2688704372543,61.2339879780998,-10.));
#37597=CARTESIAN_POINT('Ctrl Pts',(64.217753895083,61.3582207618557,-10.));
#37598=CARTESIAN_POINT('Ctrl Pts',(64.1611296716898,61.4798690695452,-10.));
#37599=CARTESIAN_POINT('Ctrl Pts',(64.1136394008877,61.5818945054559,-10.));
#37600=CARTESIAN_POINT('Ctrl Pts',(64.0622740433798,61.6821018049246,-10.));
#37601=CARTESIAN_POINT('Ctrl Pts',(64.0071247254933,61.7802504068033,-10.));
#37602=CARTESIAN_POINT('Ctrl Pts',(63.9749821154106,61.8374542374444,-10.));
#37603=CARTESIAN_POINT('Ctrl Pts',(63.9415537805714,61.8939584151892,-10.));
#37604=CARTESIAN_POINT('Ctrl Pts',(63.9068550735822,61.9497121072916,-10.));
#37605=CARTESIAN_POINT('Ctrl Pts',(63.8949352721664,61.9688647788382,-10.));
#37606=CARTESIAN_POINT('Ctrl Pts',(63.8828641359213,61.9879310381597,-10.));
#37607=CARTESIAN_POINT('Ctrl Pts',(63.8706469073994,62.0069015270467,-10.));
#37608=CARTESIAN_POINT('Ctrl Pts',(63.7998198500733,62.1168793261435,-10.));
#37609=CARTESIAN_POINT('Ctrl Pts',(63.7241685217449,62.2235155057234,-10.));
#37610=CARTESIAN_POINT('Ctrl Pts',(63.6438531183809,62.3264414594354,-10.));
#37611=CARTESIAN_POINT('Ctrl Pts',(63.5707659198607,62.4201043098569,-10.));
#37612=CARTESIAN_POINT('Ctrl Pts',(63.4938156723471,62.5106946649326,-10.));
#37613=CARTESIAN_POINT('Ctrl Pts',(63.4130998283308,62.5979052737863,-10.));
#37614=CARTESIAN_POINT('Ctrl Pts',(63.3520426893251,62.6638753485895,-10.));
#37615=CARTESIAN_POINT('Ctrl Pts',(63.2888302429821,62.7279108715258,-10.));
#37616=CARTESIAN_POINT('Ctrl Pts',(63.2235668510161,62.7899187021734,-10.));
#37617=CARTESIAN_POINT('Origin',(60.,60.,-6.));
#37618=CARTESIAN_POINT('Origin',(-60.,-60.,-3.));
#37619=CARTESIAN_POINT('Ctrl Pts',(-59.1956105045055,-64.1864216867795,
-3.));
#37620=CARTESIAN_POINT('Ctrl Pts',(-59.3195769752075,-64.2229459535633,
-3.));
#37621=CARTESIAN_POINT('Ctrl Pts',(-59.4450598371526,-64.2536518518579,
-3.));
#37622=CARTESIAN_POINT('Ctrl Pts',(-59.5716384336509,-64.2786228996525,
-3.));
#37623=CARTESIAN_POINT('Ctrl Pts',(-59.7000946411857,-64.3039643569495,
-3.));
#37624=CARTESIAN_POINT('Ctrl Pts',(-59.8296800110397,-64.3233998046748,
-3.));
#37625=CARTESIAN_POINT('Ctrl Pts',(-59.9599813689613,-64.3369699541931,
-3.));
#37626=CARTESIAN_POINT('Ctrl Pts',(-60.0181562008825,-64.3430285339344,
-3.));
#37627=CARTESIAN_POINT('Ctrl Pts',(-60.0764740369278,-64.3479173489061,
-3.));
#37628=CARTESIAN_POINT('Ctrl Pts',(-60.1348992109591,-64.3516368969462,
-3.));
#37629=CARTESIAN_POINT('Ctrl Pts',(-60.1584275239312,-64.3531347904801,
-3.));
#37630=CARTESIAN_POINT('Ctrl Pts',(-60.1819732500468,-64.3544430369817,
-2.99999999999999));
#37631=CARTESIAN_POINT('Ctrl Pts',(-60.205534079903,-64.3555615786038,-2.99999999999999));
#37632=CARTESIAN_POINT('Ctrl Pts',(-60.2289634916764,-64.3566738812014,
-2.99999999999999));
#37633=CARTESIAN_POINT('Ctrl Pts',(-60.2523983629866,-64.3575981241379,
-3.));
#37634=CARTESIAN_POINT('Ctrl Pts',(-60.2758335397625,-64.3583346103257,
-3.));
#37635=CARTESIAN_POINT('Ctrl Pts',(-60.4095526409971,-64.3625369371117,
-3.));
#37636=CARTESIAN_POINT('Ctrl Pts',(-60.5433093906275,-64.360631729286,-2.99999999999999));
#37637=CARTESIAN_POINT('Ctrl Pts',(-60.6766723905723,-64.3526712769133,
-2.99999999999999));
#37638=CARTESIAN_POINT('Ctrl Pts',(-60.7846048350664,-64.3462287772377,
-3.));
#37639=CARTESIAN_POINT('Ctrl Pts',(-60.8922800261175,-64.3358192861715,
-3.));
#37640=CARTESIAN_POINT('Ctrl Pts',(-60.9994757883914,-64.3214466528355,
-3.));
#37641=CARTESIAN_POINT('Ctrl Pts',(-61.0530736695283,-64.3142603361676,
-3.));
#37642=CARTESIAN_POINT('Ctrl Pts',(-61.1065517534524,-64.3060828957079,
-3.));
#37643=CARTESIAN_POINT('Ctrl Pts',(-61.1598824475224,-64.2969127553923,
-3.));
#37644=CARTESIAN_POINT('Ctrl Pts',(-61.1872713223749,-64.2922032756102,
-3.));
#37645=CARTESIAN_POINT('Ctrl Pts',(-61.2146213234789,-64.2872319479493,
-3.));
#37646=CARTESIAN_POINT('Ctrl Pts',(-61.2419287096427,-64.2819984158526,
-3.));
#37647=CARTESIAN_POINT('Ctrl Pts',(-61.2615201519558,-64.2782436646087,
-3.));
#37648=CARTESIAN_POINT('Ctrl Pts',(-61.2810874285119,-64.2743543242779,
-3.));
#37649=CARTESIAN_POINT('Ctrl Pts',(-61.3006182223717,-64.2703327355513,
-3.));
#37650=CARTESIAN_POINT('Ctrl Pts',(-61.3068719962591,-64.2690450200214,
-3.));
#37651=CARTESIAN_POINT('Ctrl Pts',(-61.3131223455695,-64.2677436853781,
-3.));
#37652=CARTESIAN_POINT('Ctrl Pts',(-61.319369225276,-64.2664287399395,-3.));
#37653=CARTESIAN_POINT('Ctrl Pts',(-61.4494243700941,-64.2390526053768,
-3.));
#37654=CARTESIAN_POINT('Ctrl Pts',(-61.5779747925235,-64.2057813906861,
-3.));
#37655=CARTESIAN_POINT('Ctrl Pts',(-61.7046919624325,-64.1669093068584,
-3.));
#37656=CARTESIAN_POINT('Ctrl Pts',(-61.8336750528799,-64.1273421234386,
-3.));
#37657=CARTESIAN_POINT('Ctrl Pts',(-61.9607594086197,-64.0819718837584,
-3.));
#37658=CARTESIAN_POINT('Ctrl Pts',(-62.0856033789978,-64.0310550776473,
-3.));
#37659=CARTESIAN_POINT('Ctrl Pts',(-62.2120505628986,-63.9794844112669,
-3.));
#37660=CARTESIAN_POINT('Ctrl Pts',(-62.3362002069323,-63.9222236565176,
-3.));
#37661=CARTESIAN_POINT('Ctrl Pts',(-62.4576913752432,-63.8594865308942,
-3.));
#37662=CARTESIAN_POINT('Ctrl Pts',(-62.5340612523311,-63.820049700717,-3.));
#37663=CARTESIAN_POINT('Ctrl Pts',(-62.6093804939423,-63.7784478743419,
-3.));
#37664=CARTESIAN_POINT('Ctrl Pts',(-62.6835561803521,-63.7347241134274,
-3.));
#37665=CARTESIAN_POINT('Ctrl Pts',(-62.7445592832535,-63.6987650921443,
-3.));
#37666=CARTESIAN_POINT('Ctrl Pts',(-62.8047888964893,-63.6613707234564,
-3.));
#37667=CARTESIAN_POINT('Ctrl Pts',(-62.8641913966604,-63.6225612636812,
-3.));
#37668=CARTESIAN_POINT('Ctrl Pts',(-62.8791977478544,-63.6127571581072,
-3.));
#37669=CARTESIAN_POINT('Ctrl Pts',(-62.8941494905117,-63.6028638609676,
-3.));
#37670=CARTESIAN_POINT('Ctrl Pts',(-62.9090364113711,-63.5928881663496,
-3.));
#37671=CARTESIAN_POINT('Ctrl Pts',(-63.0253586853184,-63.5149408531926,
-3.));
#37672=CARTESIAN_POINT('Ctrl Pts',(-63.137885912799,-63.4318617290311,-3.));
#37673=CARTESIAN_POINT('Ctrl Pts',(-63.246261646252,-63.3439219695934,-3.));
#37674=CARTESIAN_POINT('Ctrl Pts',(-63.2693906398052,-63.3251543168699,
-3.));
#37675=CARTESIAN_POINT('Ctrl Pts',(-63.2923305198638,-63.3061650953556,
-3.));
#37676=CARTESIAN_POINT('Ctrl Pts',(-63.3150777604115,-63.2869566419458,
-3.));
#37677=CARTESIAN_POINT('Ctrl Pts',(-63.4206897880943,-63.1977746724228,
-3.));
#37678=CARTESIAN_POINT('Ctrl Pts',(-63.5221510927373,-63.1038707715521,
-3.));
#37679=CARTESIAN_POINT('Ctrl Pts',(-63.6192855100693,-63.0056344766105,
-3.));
#37680=CARTESIAN_POINT('Ctrl Pts',(-63.717532292034,-62.9062731985461,-3.));
#37681=CARTESIAN_POINT('Ctrl Pts',(-63.8113530794893,-62.8024792577487,
-3.));
#37682=CARTESIAN_POINT('Ctrl Pts',(-63.9005375394928,-62.6946104879407,
-3.));
#37683=CARTESIAN_POINT('Ctrl Pts',(-63.9806728102355,-62.5976867293296,
-3.));
#37684=CARTESIAN_POINT('Ctrl Pts',(-64.0570647853735,-62.4974722229016,
-3.));
#37685=CARTESIAN_POINT('Ctrl Pts',(-64.129536208176,-62.3942009297676,-3.));
#37686=CARTESIAN_POINT('Ctrl Pts',(-64.1412822732054,-62.3774628656051,
-3.));
#37687=CARTESIAN_POINT('Ctrl Pts',(-64.1529252913588,-62.3606444563152,
-3.));
#37688=CARTESIAN_POINT('Ctrl Pts',(-64.1644644409263,-62.3437466478903,
-3.));
#37689=CARTESIAN_POINT('Ctrl Pts',(-64.1746328675554,-62.32885611162,-3.));
#37690=CARTESIAN_POINT('Ctrl Pts',(-64.184715292135,-62.3139117392423,-3.));
#37691=CARTESIAN_POINT('Ctrl Pts',(-64.1947108963489,-62.2989151294246,
-3.));
#37692=CARTESIAN_POINT('Ctrl Pts',(-64.2739894449572,-62.1799718984846,
-3.));
#37693=CARTESIAN_POINT('Ctrl Pts',(-64.3478188937706,-62.0577313604119,
-3.));
#37694=CARTESIAN_POINT('Ctrl Pts',(-64.4160215697397,-61.9326058716527,
-3.));
#37695=CARTESIAN_POINT('Ctrl Pts',(-64.4849569622618,-61.8061361318724,
-3.));
#37696=CARTESIAN_POINT('Ctrl Pts',(-64.5481446100938,-61.6767185791534,
-3.));
#37697=CARTESIAN_POINT('Ctrl Pts',(-64.6053684527712,-61.5447373590947,
-3.));
#37698=CARTESIAN_POINT('Ctrl Pts',(-64.6262260898092,-61.4966312506089,
-3.));
#37699=CARTESIAN_POINT('Ctrl Pts',(-64.6462910549685,-61.448184191749,-3.));
#37700=CARTESIAN_POINT('Ctrl Pts',(-64.6655515905053,-61.3994136515623,
-3.));
#37701=CARTESIAN_POINT('Ctrl Pts',(-64.7181182489016,-61.2663070553886,
-3.));
#37702=CARTESIAN_POINT('Ctrl Pts',(-64.764696319996,-61.13079266721,-3.));
#37703=CARTESIAN_POINT('Ctrl Pts',(-64.8052734588863,-60.993284910806,-3.));
#37704=CARTESIAN_POINT('Ctrl Pts',(-64.8290066045075,-60.9128580572618,
-3.));
#37705=CARTESIAN_POINT('Ctrl Pts',(-64.8506859899574,-60.831748786273,-3.));
#37706=CARTESIAN_POINT('Ctrl Pts',(-64.8703015413704,-60.750036894404,-3.));
#37707=CARTESIAN_POINT('Ctrl Pts',(-64.8777895131791,-60.7188444833486,
-3.));
#37708=CARTESIAN_POINT('Ctrl Pts',(-64.8849766776954,-60.6875642384272,
-3.));
#37709=CARTESIAN_POINT('Ctrl Pts',(-64.8918622508146,-60.656200539862,-3.));
#37710=CARTESIAN_POINT('Ctrl Pts',(-64.8973648511838,-60.6311362647006,
-3.));
#37711=CARTESIAN_POINT('Ctrl Pts',(-64.9026757017017,-60.6060140560556,
-3.));
#37712=CARTESIAN_POINT('Ctrl Pts',(-64.9077886731734,-60.5808652409076,
-3.));
#37713=CARTESIAN_POINT('Ctrl Pts',(-64.9369314962056,-60.4375224756745,
-3.));
#37714=CARTESIAN_POINT('Ctrl Pts',(-64.9596873210609,-60.293155610705,-3.));
#37715=CARTESIAN_POINT('Ctrl Pts',(-64.9761060740654,-60.1482217119791,
-3.));
#37716=CARTESIAN_POINT('Ctrl Pts',(-64.9926869198554,-60.0018569652858,
-3.));
#37717=CARTESIAN_POINT('Ctrl Pts',(-65.0028051887902,-59.8549132164108,
-3.));
#37718=CARTESIAN_POINT('Ctrl Pts',(-65.0064655295109,-59.707835000365,-3.));
#37719=CARTESIAN_POINT('Ctrl Pts',(-65.0101294137172,-59.5606144015204,
-3.));
#37720=CARTESIAN_POINT('Ctrl Pts',(-65.0073230416735,-59.4132582968452,
-3.));
#37721=CARTESIAN_POINT('Ctrl Pts',(-64.9980013952553,-59.2661977118922,
-3.));
#37722=CARTESIAN_POINT('Ctrl Pts',(-64.9923757136022,-59.1774455754613,
-3.));
#37723=CARTESIAN_POINT('Ctrl Pts',(-64.9843760617657,-59.0888008393423,
-3.));
#37724=CARTESIAN_POINT('Ctrl Pts',(-64.9739833680071,-59.0003574710342,
-3.));
#37725=CARTESIAN_POINT('Ctrl Pts',(-64.9615316286333,-58.8943913185524,
-3.));
#37726=CARTESIAN_POINT('Ctrl Pts',(-64.945645012555,-58.7887140863586,-3.));
#37727=CARTESIAN_POINT('Ctrl Pts',(-64.9263786176897,-58.683468154111,-3.));
#37728=CARTESIAN_POINT('Ctrl Pts',(-63.6032183801568,-56.3921449163111,
-3.));
#37729=CARTESIAN_POINT('Ctrl Pts',(-63.4898426947805,-56.2959035274869,
-3.));
#37730=CARTESIAN_POINT('Ctrl Pts',(-63.3723223864688,-56.2048634114124,
-3.));
#37731=CARTESIAN_POINT('Ctrl Pts',(-63.251055780641,-56.1192063947302,-3.));
#37732=CARTESIAN_POINT('Ctrl Pts',(-63.129678168823,-56.0334709686467,-3.));
#37733=CARTESIAN_POINT('Ctrl Pts',(-63.0045466457224,-55.9531282054953,
-3.));
#37734=CARTESIAN_POINT('Ctrl Pts',(-62.8760397304487,-55.8784080151765,
-3.));
#37735=CARTESIAN_POINT('Ctrl Pts',(-62.8196879527792,-55.8456423422685,
-3.));
#37736=CARTESIAN_POINT('Ctrl Pts',(-62.762686909838,-55.8139584898394,-3.00000000000001));
#37737=CARTESIAN_POINT('Ctrl Pts',(-62.7050678179436,-55.7833789513493,
-3.00000000000001));
#37738=CARTESIAN_POINT('Ctrl Pts',(-62.6757305829629,-55.7678091275846,
-3.00000000000001));
#37739=CARTESIAN_POINT('Ctrl Pts',(-62.6462331190597,-55.7525256196819,
-3.00000000000001));
#37740=CARTESIAN_POINT('Ctrl Pts',(-62.6165795262305,-55.737531594111,-3.00000000000001));
#37741=CARTESIAN_POINT('Ctrl Pts',(-62.5949658489926,-55.7266028668215,
-3.00000000000001));
#37742=CARTESIAN_POINT('Ctrl Pts',(-62.5732698365523,-55.7158283111196,
-3.));
#37743=CARTESIAN_POINT('Ctrl Pts',(-62.5515051559284,-55.7052148415274,
-3.));
#37744=CARTESIAN_POINT('Ctrl Pts',(-62.4199918158176,-55.6410828259762,
-3.));
#37745=CARTESIAN_POINT('Ctrl Pts',(-62.2858584006406,-55.5827701223888,
-3.));
#37746=CARTESIAN_POINT('Ctrl Pts',(-62.1494741826111,-55.5304873365666,
-3.));
#37747=CARTESIAN_POINT('Ctrl Pts',(-62.0315669656725,-55.4852876950014,
-3.));
#37748=CARTESIAN_POINT('Ctrl Pts',(-61.9119769355875,-55.4445954662697,
-3.00000000000001));
#37749=CARTESIAN_POINT('Ctrl Pts',(-61.7909378382297,-55.4085780791561,
-3.00000000000001));
#37750=CARTESIAN_POINT('Ctrl Pts',(-61.7304182895508,-55.3905693855993,
-3.00000000000001));
#37751=CARTESIAN_POINT('Ctrl Pts',(-61.6695364403128,-55.3737298700684,
-3.00000000000001));
#37752=CARTESIAN_POINT('Ctrl Pts',(-61.6083215243732,-55.3580833488014,
-3.00000000000001));
#37753=CARTESIAN_POINT('Ctrl Pts',(-61.5794892144394,-55.3507138156797,
-3.00000000000001));
#37754=CARTESIAN_POINT('Ctrl Pts',(-61.550583018072,-55.3436089674838,-3.));
#37755=CARTESIAN_POINT('Ctrl Pts',(-61.5216060047899,-55.3367714460112,
-3.));
#37756=CARTESIAN_POINT('Ctrl Pts',(-61.495341183815,-55.3305739033024,-3.));
#37757=CARTESIAN_POINT('Ctrl Pts',(-61.469014297269,-55.3245952282657,-3.00000000000001));
#37758=CARTESIAN_POINT('Ctrl Pts',(-61.4426542119394,-55.3188429929397,
-3.00000000000001));
#37759=CARTESIAN_POINT('Ctrl Pts',(-61.4363511262509,-55.3174675485241,
-3.00000000000001));
#37760=CARTESIAN_POINT('Ctrl Pts',(-61.4300458619349,-55.3161049811205,
-3.00000000000001));
#37761=CARTESIAN_POINT('Ctrl Pts',(-61.423738450879,-55.3147553063535,-3.00000000000001));
#37762=CARTESIAN_POINT('Ctrl Pts',(-61.2841865141129,-55.2848936521691,
-3.00000000000001));
#37763=CARTESIAN_POINT('Ctrl Pts',(-61.1435843785244,-55.2613388246454,
-3.00000000000001));
#37764=CARTESIAN_POINT('Ctrl Pts',(-61.0023538690712,-55.2440351533839,
-3.));
#37765=CARTESIAN_POINT('Ctrl Pts',(-60.8601845317392,-55.2266164562045,
-3.));
#37766=CARTESIAN_POINT('Ctrl Pts',(-60.7173776215922,-55.2155323614428,
-3.));
#37767=CARTESIAN_POINT('Ctrl Pts',(-60.5743626033957,-55.210778665957,-3.));
#37768=CARTESIAN_POINT('Ctrl Pts',(-60.4327944357155,-55.2060730625307,
-3.));
#37769=CARTESIAN_POINT('Ctrl Pts',(-60.2910215895177,-55.2075706082915,
-3.));
#37770=CARTESIAN_POINT('Ctrl Pts',(-60.1494715736686,-55.2153164997798,
-3.));
#37771=CARTESIAN_POINT('Ctrl Pts',(-60.0601035604392,-55.2202068908465,
-3.));
#37772=CARTESIAN_POINT('Ctrl Pts',(-59.9708246262431,-55.2275888864629,
-3.));
#37773=CARTESIAN_POINT('Ctrl Pts',(-59.8817466888378,-55.2374836515892,
-3.));
#37774=CARTESIAN_POINT('Ctrl Pts',(-59.8149382357838,-55.244904725434,-3.));
#37775=CARTESIAN_POINT('Ctrl Pts',(-59.7482429092863,-55.2537393878111,
-3.));
#37776=CARTESIAN_POINT('Ctrl Pts',(-59.6817096243707,-55.2639993082479,
-3.));
#37777=CARTESIAN_POINT('Ctrl Pts',(-59.6640768304109,-55.2667184143816,
-3.));
#37778=CARTESIAN_POINT('Ctrl Pts',(-59.6464554266234,-55.2695376386596,
-3.));
#37779=CARTESIAN_POINT('Ctrl Pts',(-59.6288463434743,-55.272457225627,-3.));
#37780=CARTESIAN_POINT('Ctrl Pts',(-59.6106485602809,-55.2754744190945,
-3.));
#37781=CARTESIAN_POINT('Ctrl Pts',(-59.5924726121038,-55.2785973698234,
-3.));
#37782=CARTESIAN_POINT('Ctrl Pts',(-59.5743220572586,-55.2818255665583,
-3.));
#37783=CARTESIAN_POINT('Ctrl Pts',(-59.4370113023005,-55.3062471963439,
-3.));
#37784=CARTESIAN_POINT('Ctrl Pts',(-59.301103309529,-55.3366962002016,-3.));
#37785=CARTESIAN_POINT('Ctrl Pts',(-59.1669958586959,-55.3731700865706,
-3.));
#37786=CARTESIAN_POINT('Ctrl Pts',(-59.1418080575942,-55.3800205411096,
-3.));
#37787=CARTESIAN_POINT('Ctrl Pts',(-59.116683813921,-55.3870836687706,-3.));
#37788=CARTESIAN_POINT('Ctrl Pts',(-59.0916258294163,-55.3943596481952,
-3.));
#37789=CARTESIAN_POINT('Ctrl Pts',(-58.9576617593453,-55.4332582203163,
-3.));
#37790=CARTESIAN_POINT('Ctrl Pts',(-58.8255893716933,-55.4782367586987,
-3.));
#37791=CARTESIAN_POINT('Ctrl Pts',(-58.6957822734934,-55.5290865431825,
-3.));
#37792=CARTESIAN_POINT('Ctrl Pts',(-58.5664089361555,-55.5797664090204,
-3.));
#37793=CARTESIAN_POINT('Ctrl Pts',(-58.4392851252412,-55.636278851372,-3.));
#37794=CARTESIAN_POINT('Ctrl Pts',(-58.3148123789666,-55.6984578656476,
-3.));
#37795=CARTESIAN_POINT('Ctrl Pts',(-58.2087252890362,-55.7514525241305,
-3.));
#37796=CARTESIAN_POINT('Ctrl Pts',(-58.1045642359244,-55.8085642160639,
-3.));
#37797=CARTESIAN_POINT('Ctrl Pts',(-58.0026013764877,-55.8697095384881,
-3.));
#37798=CARTESIAN_POINT('Ctrl Pts',(-57.984257187675,-55.8807102238922,-3.));
#37799=CARTESIAN_POINT('Ctrl Pts',(-57.9659842134992,-55.8918415103031,
-3.));
#37800=CARTESIAN_POINT('Ctrl Pts',(-57.9477841256088,-55.9031029645992,
-3.));
#37801=CARTESIAN_POINT('Ctrl Pts',(-57.9313889896199,-55.9132475900389,
-3.));
#37802=CARTESIAN_POINT('Ctrl Pts',(-57.9150608534493,-55.9234930063007,
-3.));
#37803=CARTESIAN_POINT('Ctrl Pts',(-57.8988041215737,-55.9338364228883,
-3.));
#37804=CARTESIAN_POINT('Ctrl Pts',(-57.7839056269251,-56.0069410914355,
-3.));
#37805=CARTESIAN_POINT('Ctrl Pts',(-57.6725153636961,-56.0849724426437,
-3.));
#37806=CARTESIAN_POINT('Ctrl Pts',(-57.5649776520738,-56.1677286853735,
-3.));
#37807=CARTESIAN_POINT('Ctrl Pts',(-57.4583964400229,-56.2497488485504,
-3.));
#37808=CARTESIAN_POINT('Ctrl Pts',(-57.3555989995654,-56.3364107540539,
-3.));
#37809=CARTESIAN_POINT('Ctrl Pts',(-57.2569565735731,-56.4275538681827,
-3.));
#37810=CARTESIAN_POINT('Ctrl Pts',(-57.224173905029,-56.4578442272297,-3.));
#37811=CARTESIAN_POINT('Ctrl Pts',(-57.1918504858555,-56.4886297926312,
-3.));
#37812=CARTESIAN_POINT('Ctrl Pts',(-57.1600009946507,-56.5199054102076,
-3.));
#37813=CARTESIAN_POINT('Ctrl Pts',(-57.063427842614,-56.6147384783981,-3.));
#37814=CARTESIAN_POINT('Ctrl Pts',(-56.9712084392596,-56.7140758024186,
-3.));
#37815=CARTESIAN_POINT('Ctrl Pts',(-56.8836152244926,-56.8175811575214,
-3.));
#37816=CARTESIAN_POINT('Ctrl Pts',(-56.8363965206617,-56.8733775878787,
-3.));
#37817=CARTESIAN_POINT('Ctrl Pts',(-56.7905229834664,-56.930385559123,-3.));
#37818=CARTESIAN_POINT('Ctrl Pts',(-56.7460434065629,-56.9885540563686,
-3.));
#37819=CARTESIAN_POINT('Ctrl Pts',(-56.7284856804581,-57.0115153031624,
-3.));
#37820=CARTESIAN_POINT('Ctrl Pts',(-56.711145206329,-57.034657388313,-3.));
#37821=CARTESIAN_POINT('Ctrl Pts',(-56.69402518081,-57.0579772003701,-3.));
#37822=CARTESIAN_POINT('Ctrl Pts',(-56.6800434073205,-57.077022284715,-3.));
#37823=CARTESIAN_POINT('Ctrl Pts',(-56.6662063227873,-57.0961893605202,
-3.));
#37824=CARTESIAN_POINT('Ctrl Pts',(-56.652531641636,-57.1154538907109,-3.));
#37825=CARTESIAN_POINT('Ctrl Pts',(-56.5757648226242,-57.2236009609155,
-3.));
#37826=CARTESIAN_POINT('Ctrl Pts',(-56.5040156722043,-57.33494533068,-3.));
#37827=CARTESIAN_POINT('Ctrl Pts',(-56.4374818319856,-57.4491372747288,
-3.));
#37828=CARTESIAN_POINT('Ctrl Pts',(-56.3711910735432,-57.5629120178389,
-3.));
#37829=CARTESIAN_POINT('Ctrl Pts',(-56.31007728771,-57.6795143228349,-3.));
#37830=CARTESIAN_POINT('Ctrl Pts',(-56.2543835770224,-57.7986178389126,
-3.));
#37831=CARTESIAN_POINT('Ctrl Pts',(-56.1996788698177,-57.9156063263675,
-3.));
#37832=CARTESIAN_POINT('Ctrl Pts',(-56.1502032929139,-58.0350086810399,
-3.));
#37833=CARTESIAN_POINT('Ctrl Pts',(-56.1062364267016,-58.1565237324278,
-3.));
#37834=CARTESIAN_POINT('Ctrl Pts',(-56.0839234950841,-58.2181919218099,
-3.));
#37835=CARTESIAN_POINT('Ctrl Pts',(-56.0630301391519,-58.2804043026903,
-3.));
#37836=CARTESIAN_POINT('Ctrl Pts',(-56.0435980798389,-58.3431214745369,
-3.));
#37837=CARTESIAN_POINT('Ctrl Pts',(-56.0170092495455,-58.4289371985343,
-3.));
#37838=CARTESIAN_POINT('Ctrl Pts',(-55.9931559588827,-58.5156982188528,
-3.));
#37839=CARTESIAN_POINT('Ctrl Pts',(-55.9720760639888,-58.6032685615972,
-3.));
#37840=CARTESIAN_POINT('Origin',(-60.,-60.,-13.3123464956316));
#37841=CARTESIAN_POINT('Ctrl Pts',(-54.9007452025866,-59.9999087514893,
-9.56234649563159));
#37842=CARTESIAN_POINT('Ctrl Pts',(-54.900655342442,-59.8930270619539,-9.55734157105847));
#37843=CARTESIAN_POINT('Ctrl Pts',(-54.9296018038888,-58.9539304600107,
-9.51336443385491));
#37844=CARTESIAN_POINT('Ctrl Pts',(-55.4826600864412,-57.2140033424977,
-9.43041508402093));
#37845=CARTESIAN_POINT('Ctrl Pts',(-57.3241694777564,-55.4165445512788,
-9.31349844612963));
#37846=CARTESIAN_POINT('Ctrl Pts',(-59.7947368654586,-54.6966046195577,
-9.19658180823835));
#37847=CARTESIAN_POINT('Ctrl Pts',(-62.3135594050244,-55.2234345982174,
-9.07966517034706));
#37848=CARTESIAN_POINT('Ctrl Pts',(-64.2884897146217,-56.8731819984634,
-8.96274853245577));
#37849=CARTESIAN_POINT('Ctrl Pts',(-65.2552435912467,-59.2580098856016,
-8.84583189456447));
#37850=CARTESIAN_POINT('Ctrl Pts',(-64.986547872926,-61.817271139308,-8.72891525667319));
#37851=CARTESIAN_POINT('Ctrl Pts',(-63.5455699794028,-63.9493126448601,
-8.6119986187819));
#37852=CARTESIAN_POINT('Ctrl Pts',(-61.2710678060581,-65.1529132589701,
-8.49508198089061));
#37853=CARTESIAN_POINT('Ctrl Pts',(-58.6977517372794,-65.1451236320635,
-8.37816534299932));
#37854=CARTESIAN_POINT('Ctrl Pts',(-56.4305796611695,-63.9277667709211,
-8.26124870510803));
#37855=CARTESIAN_POINT('Ctrl Pts',(-55.1447571992843,-62.0002411018557,
-8.15597575598545));
#37856=CARTESIAN_POINT('Ctrl Pts',(-54.9016527228214,-60.5836272117911,
-8.08967501949331));
#37857=CARTESIAN_POINT('Ctrl Pts',(-54.9011518411408,-59.9998830094301,
-8.06234649563159));
#37858=CARTESIAN_POINT('Ctrl Pts',(-54.9012106606313,-59.9998804662267,
-9.68765350436841));
#37859=CARTESIAN_POINT('Ctrl Pts',(-54.9010041861375,-59.7264420560186,
-9.67485236502099));
#37860=CARTESIAN_POINT('Ctrl Pts',(-54.9885269673505,-58.6206708842071,
-9.62307901304313));
#37861=CARTESIAN_POINT('Ctrl Pts',(-55.7768178205809,-56.785492732961,-9.53233344843484));
#37862=CARTESIAN_POINT('Ctrl Pts',(-57.7853302129478,-55.1767966332062,
-9.41541681054355));
#37863=CARTESIAN_POINT('Ctrl Pts',(-60.3144620635955,-54.7019555263241,
-9.29850017265227));
#37864=CARTESIAN_POINT('Ctrl Pts',(-62.7696789900454,-55.4726379404574,
-9.18158353476098));
#37865=CARTESIAN_POINT('Ctrl Pts',(-64.5737696881318,-57.3076474190762,
-9.06466689686968));
#37866=CARTESIAN_POINT('Ctrl Pts',(-65.3026202647668,-59.7756017648733,
-8.9477502589784));
#37867=CARTESIAN_POINT('Ctrl Pts',(-64.7848823729,-62.2963084445819,-8.8308336210871));
#37868=CARTESIAN_POINT('Ctrl Pts',(-63.1422721548051,-64.2771789992941,
-8.71391698319582));
#37869=CARTESIAN_POINT('Ctrl Pts',(-60.7609482822248,-65.252531849864,-8.59700034530452));
#37870=CARTESIAN_POINT('Ctrl Pts',(-58.2007340409931,-64.9930727838061,
-8.48008370741324));
#37871=CARTESIAN_POINT('Ctrl Pts',(-56.0635071815643,-63.5597974366436,
-8.36316706952195));
#37872=CARTESIAN_POINT('Ctrl Pts',(-55.0531943003858,-61.6671136005503,
-8.26569033517368));
#37873=CARTESIAN_POINT('Ctrl Pts',(-54.9013976662957,-60.4172707815651,
-8.20718581345583));
#37874=CARTESIAN_POINT('Ctrl Pts',(-54.901395125587,-59.9999990971874,-8.18765350436841));
#37875=CARTESIAN_POINT('Ctrl Pts',(-63.2233527839579,-57.2101674189746,
-10.));
#37876=CARTESIAN_POINT('Ctrl Pts',(-63.6787829722545,-57.7363682294924,
-9.96102778736957));
#37877=CARTESIAN_POINT('Ctrl Pts',(-64.3265775369929,-59.0156060985281,
-9.8830833621087));
#37878=CARTESIAN_POINT('Ctrl Pts',(-64.2810882742281,-61.1667237108393,
-9.76616672421743));
#37879=CARTESIAN_POINT('Ctrl Pts',(-63.22907753389,-63.0432886084162,-9.64925008632613));
#37880=CARTESIAN_POINT('Ctrl Pts',(-61.4179627144323,-64.2045560607698,
-9.53233344843485));
#37881=CARTESIAN_POINT('Ctrl Pts',(-59.2734876096321,-64.3773165471069,
-9.41541681054355));
#37882=CARTESIAN_POINT('Ctrl Pts',(-57.2998122798752,-63.5210484654286,
-9.29850017265226));
#37883=CARTESIAN_POINT('Ctrl Pts',(-55.9609186974804,-61.8370072168577,
-9.18158353476097));
#37884=CARTESIAN_POINT('Ctrl Pts',(-55.5715694949038,-59.7211123005161,
-9.06466689686968));
#37885=CARTESIAN_POINT('Ctrl Pts',(-56.2232947535789,-57.6707778484149,
-8.94775025897839));
#37886=CARTESIAN_POINT('Ctrl Pts',(-57.7628818363748,-56.1680191061191,
-8.83083362108711));
#37887=CARTESIAN_POINT('Ctrl Pts',(-59.8283905192097,-55.5661160017993,
-8.71391698319581));
#37888=CARTESIAN_POINT('Ctrl Pts',(-61.9342427424238,-56.0065702475388,
-8.59700034530453));
#37889=CARTESIAN_POINT('Ctrl Pts',(-63.5853758881021,-57.3858354303686,
-8.48008370741323));
#37890=CARTESIAN_POINT('Ctrl Pts',(-64.3936268737958,-59.3796619224004,
-8.36316706952195));
#37891=CARTESIAN_POINT('Ctrl Pts',(-64.1689848170786,-61.5193227822848,
-8.24625043163066));
#37892=CARTESIAN_POINT('Ctrl Pts',(-62.9642606044702,-63.3018081594506,
-8.12933379373937));
#37893=CARTESIAN_POINT('Ctrl Pts',(-61.0626715154394,-64.3080739797979,
-8.01241715584808));
#37894=CARTESIAN_POINT('Ctrl Pts',(-58.9112601796474,-64.3015614911722,
-7.89550051795679));
#37895=CARTESIAN_POINT('Ctrl Pts',(-57.0157993911679,-63.2837948116173,
-7.7785838800655));
#37896=CARTESIAN_POINT('Ctrl Pts',(-55.821891404445,-61.494054502106,-7.66166724217421));
#37897=CARTESIAN_POINT('Ctrl Pts',(-55.6102098839069,-59.3530565588066,
-7.54475060428292));
#37898=CARTESIAN_POINT('Ctrl Pts',(-56.4305207206919,-57.3641952812435,
-7.42783396639163));
#37899=CARTESIAN_POINT('Ctrl Pts',(-58.0899737985984,-55.9948801098928,
-7.31091732850034));
#37900=CARTESIAN_POINT('Ctrl Pts',(-60.1984589793919,-55.5673454264546,
-7.19400069060905));
#37901=CARTESIAN_POINT('Ctrl Pts',(-62.2602755454619,-56.1814013752741,
-7.07708405271777));
#37902=CARTESIAN_POINT('Ctrl Pts',(-63.7907548567845,-57.6941990354335,
-6.96016741482647));
#37903=CARTESIAN_POINT('Ctrl Pts',(-64.4300090149408,-59.7468405219862,
-6.84325077693519));
#37904=CARTESIAN_POINT('Ctrl Pts',(-64.027951567412,-61.8638120783306,-6.72633413904389));
#37905=CARTESIAN_POINT('Ctrl Pts',(-62.6786998800996,-63.5322833334212,
-6.60941750115261));
#37906=CARTESIAN_POINT('Ctrl Pts',(-60.0407216297232,-64.6795907924263,
-6.45352865063089));
#37907=CARTESIAN_POINT('Ctrl Pts',(-56.338126950977,-63.4214738666151,-6.25866758747873));
#37908=CARTESIAN_POINT('Ctrl Pts',(-55.1221049933237,-58.8502443951291,
-6.02483431169616));
#37909=CARTESIAN_POINT('Ctrl Pts',(-57.7101825725057,-55.9187055503882,
-5.829973248544));
#37910=CARTESIAN_POINT('Ctrl Pts',(-60.5695480146307,-55.6036294907912,
-5.67408439802229));
#37911=CARTESIAN_POINT('Ctrl Pts',(-62.5694772512366,-56.3811637301305,
-5.557167760131));
#37912=CARTESIAN_POINT('Ctrl Pts',(-63.9702557757387,-58.0185513710953,
-5.44025112223971));
#37913=CARTESIAN_POINT('Ctrl Pts',(-64.4353953405457,-60.1175101930552,
-5.32333448434842));
#37914=CARTESIAN_POINT('Ctrl Pts',(-63.8588751961196,-62.1908042402258,
-5.20641784645712));
#37915=CARTESIAN_POINT('Ctrl Pts',(-62.374688451214,-63.7481551854853,-5.08950120856584));
#37916=CARTESIAN_POINT('Ctrl Pts',(-60.3324645667982,-64.4247771397016,
-4.97258457067455));
#37917=CARTESIAN_POINT('Ctrl Pts',(-58.211977347927,-64.0609880370046,-4.85566793278326));
#37918=CARTESIAN_POINT('Ctrl Pts',(-56.5118828933347,-62.7425958741262,
-4.73875129489197));
#37919=CARTESIAN_POINT('Ctrl Pts',(-55.6317837173695,-60.7794079817936,
-4.62183465700068));
#37920=CARTESIAN_POINT('Ctrl Pts',(-55.7786142136362,-58.6330092626113,
-4.50491801910939));
#37921=CARTESIAN_POINT('Ctrl Pts',(-56.9178409549638,-56.807965963808,-4.3880013812181));
#37922=CARTESIAN_POINT('Ctrl Pts',(-58.7816513959293,-55.7333386780497,
-4.27108474332682));
#37923=CARTESIAN_POINT('Ctrl Pts',(-60.9318810589847,-55.6617543020258,
-4.15416810543552));
#37924=CARTESIAN_POINT('Ctrl Pts',(-62.8630363094296,-56.6100443537648,
-4.03725146754423));
#37925=CARTESIAN_POINT('Ctrl Pts',(-64.1211231401667,-58.355275016248,-3.92033482965294));
#37926=CARTESIAN_POINT('Ctrl Pts',(-64.4103797861807,-60.4871625360835,
-3.80341819176165));
#37927=CARTESIAN_POINT('Ctrl Pts',(-63.662804640575,-62.5045233774706,-3.68650155387036));
#37928=CARTESIAN_POINT('Ctrl Pts',(-62.0541453235499,-63.933098699237,-3.56958491597908));
#37929=CARTESIAN_POINT('Ctrl Pts',(-59.9625778280873,-64.4370457120861,
-3.45266827808779));
#37930=CARTESIAN_POINT('Ctrl Pts',(-57.8798107750803,-63.897893141119,-3.3357516401965));
#37931=CARTESIAN_POINT('Ctrl Pts',(-56.295470437015,-62.4423875072701,-3.21883500230521));
#37932=CARTESIAN_POINT('Ctrl Pts',(-55.5820374288072,-60.4127070705911,
-3.10191836441392));
#37933=CARTESIAN_POINT('Ctrl Pts',(-55.9071888340358,-58.2859968821596,
-2.98500172652263));
#37934=CARTESIAN_POINT('Ctrl Pts',(-57.1945761362646,-56.5622472138891,
-2.86808508863134));
#37935=CARTESIAN_POINT('Ctrl Pts',(-59.141343048511,-55.6466485015553,-2.75116845074005));
#37936=CARTESIAN_POINT('Ctrl Pts',(-61.2902328481645,-55.7545784974516,
-2.63425181284876));
#37937=CARTESIAN_POINT('Ctrl Pts',(-62.5200516280627,-56.4918932825098,
-2.5563073875879));
#37938=CARTESIAN_POINT('Ctrl Pts',(-63.0124573356753,-56.9836661655686,
-2.51733517495747));
#37939=CARTESIAN_POINT('Ctrl Pts',(-63.4340590883905,-57.0277997563163,
-10.1608882750142));
#37940=CARTESIAN_POINT('Ctrl Pts',(-63.9192601452004,-57.5883976172362,
-10.1219160623837));
#37941=CARTESIAN_POINT('Ctrl Pts',(-64.6094001830892,-58.9512575723235,
-10.0439716371229));
#37942=CARTESIAN_POINT('Ctrl Pts',(-64.5609373474359,-61.2429908953152,
-9.92705499923159));
#37943=CARTESIAN_POINT('Ctrl Pts',(-63.4401580576473,-63.2422243560614,
-9.81013836134031));
#37944=CARTESIAN_POINT('Ctrl Pts',(-61.5106530599844,-64.4794023244967,
-9.69322172344902));
#37945=CARTESIAN_POINT('Ctrl Pts',(-59.2259964564264,-64.6634559351264,
-9.57630508555773));
#37946=CARTESIAN_POINT('Ctrl Pts',(-57.1233045831027,-63.7512147424712,
-9.45938844766644));
#37947=CARTESIAN_POINT('Ctrl Pts',(-55.6968892996459,-61.9570899468048,
-9.34247180977515));
#37948=CARTESIAN_POINT('Ctrl Pts',(-55.2820888551148,-59.7028817807907,
-9.22555517188386));
#37949=CARTESIAN_POINT('Ctrl Pts',(-55.9764165311997,-57.5185196797758,
-9.10863853399257));
#37950=CARTESIAN_POINT('Ctrl Pts',(-57.616644383502,-55.917527587839,-8.99172189610128));
#37951=CARTESIAN_POINT('Ctrl Pts',(-59.817172634626,-55.2762788743854,-8.87480525820999));
#37952=CARTESIAN_POINT('Ctrl Pts',(-62.0606816299573,-55.7455250310983,
-8.75788862031871));
#37953=CARTESIAN_POINT('Ctrl Pts',(-63.8197471636086,-57.2149509530668,
-8.64097198242741));
#37954=CARTESIAN_POINT('Ctrl Pts',(-64.6808324462795,-59.3391112434675,
-8.52405534453613));
#37955=CARTESIAN_POINT('Ctrl Pts',(-64.4415058356944,-61.6186389012925,
-8.40713870664484));
#37956=CARTESIAN_POINT('Ctrl Pts',(-63.1580303961144,-63.5176429879204,
-8.29022206875354));
#37957=CARTESIAN_POINT('Ctrl Pts',(-61.1321369456456,-64.5896870728554,
-8.17330543086226));
#37958=CARTESIAN_POINT('Ctrl Pts',(-58.8400906988581,-64.5827488714692,
-8.05638879297096));
#37959=CARTESIAN_POINT('Ctrl Pts',(-56.8207261478351,-63.4984521313852,
-7.93947215507967));
#37960=CARTESIAN_POINT('Ctrl Pts',(-55.5487739765082,-61.5917188670885,
-7.82255551718839));
#37961=CARTESIAN_POINT('Ctrl Pts',(-55.3232551151952,-59.3107667224756,
-7.7056388792971));
#37962=CARTESIAN_POINT('Ctrl Pts',(-56.1971885854583,-57.1918962160405,
-7.58872224140581));
#37963=CARTESIAN_POINT('Ctrl Pts',(-57.9651179142938,-55.7330707246297,
-7.47180560351452));
#37964=CARTESIAN_POINT('Ctrl Pts',(-60.2114319801559,-55.277588664903,-7.35488896562322));
#37965=CARTESIAN_POINT('Ctrl Pts',(-62.4080267657298,-55.9317846382132,
-7.23797232773194));
#37966=CARTESIAN_POINT('Ctrl Pts',(-64.0385514835944,-57.543471878785,-7.12105568984065));
#37967=CARTESIAN_POINT('Ctrl Pts',(-64.7195928398286,-59.7302918220393,
-7.00413905194936));
#37968=CARTESIAN_POINT('Ctrl Pts',(-64.2912534291961,-61.985647006588,-6.88722241405807));
#37969=CARTESIAN_POINT('Ctrl Pts',(-62.8538029452151,-63.7631840189119,
-6.77030577616678));
#37970=CARTESIAN_POINT('Ctrl Pts',(-60.0433835487511,-64.9854894477136,
-6.61441692564506));
#37971=CARTESIAN_POINT('Ctrl Pts',(-56.0987551573276,-63.6451310839495,
-6.41955586249291));
#37972=CARTESIAN_POINT('Ctrl Pts',(-54.8032434540649,-58.7750863932782,
-6.18572258671033));
#37973=CARTESIAN_POINT('Ctrl Pts',(-57.5605002385166,-55.6519167350097,
-5.99086152355818));
#37974=CARTESIAN_POINT('Ctrl Pts',(-60.606778614383,-55.3162445704927,-5.83497267303647));
#37975=CARTESIAN_POINT('Ctrl Pts',(-62.7374405776916,-56.1446051937624,
-5.71805603514518));
#37976=CARTESIAN_POINT('Ctrl Pts',(-64.2297861399983,-57.8890266972534,
-5.60113939725388));
#37977=CARTESIAN_POINT('Ctrl Pts',(-64.7253312624079,-60.1251916788159,
-5.4842227593626));
#37978=CARTESIAN_POINT('Ctrl Pts',(-64.1111247593346,-62.3340142132361,
-5.3673061214713));
#37979=CARTESIAN_POINT('Ctrl Pts',(-62.5299186916718,-63.9931671281756,
-5.25038948358002));
#37980=CARTESIAN_POINT('Ctrl Pts',(-60.3541973354151,-64.714018963831,-5.13347284568873));
#37981=CARTESIAN_POINT('Ctrl Pts',(-58.0950966741345,-64.3264494490725,
-5.01655620779744));
#37982=CARTESIAN_POINT('Ctrl Pts',(-56.28386929562,-62.9218757357862,-4.89963956990615));
#37983=CARTESIAN_POINT('Ctrl Pts',(-55.3462392015919,-60.8303568497879,
-4.78272293201486));
#37984=CARTESIAN_POINT('Ctrl Pts',(-55.5026678130263,-58.5436508877221,
-4.66580629412357));
#37985=CARTESIAN_POINT('Ctrl Pts',(-56.7163642983331,-56.5993069244573,
-4.54888965623228));
#37986=CARTESIAN_POINT('Ctrl Pts',(-58.7020095605236,-55.454432675614,-4.43197301834099));
#37987=CARTESIAN_POINT('Ctrl Pts',(-60.9927968901921,-55.3781689236924,
-4.3150563804497));
#37988=CARTESIAN_POINT('Ctrl Pts',(-63.050189202907,-56.3884474407729,-4.19813974255841));
#37989=CARTESIAN_POINT('Ctrl Pts',(-64.3905155043218,-58.247761521337,-4.08122310466712));
#37990=CARTESIAN_POINT('Ctrl Pts',(-64.6986804743695,-60.5190077061645,
-3.96430646677583));
#37991=CARTESIAN_POINT('Ctrl Pts',(-63.902237331131,-62.668240755183,-3.84738982888454));
#37992=CARTESIAN_POINT('Ctrl Pts',(-62.1884220840853,-64.1902001545941,
-3.73047319099325));
#37993=CARTESIAN_POINT('Ctrl Pts',(-59.9601315902486,-64.7270895165512,
-3.61355655310196));
#37994=CARTESIAN_POINT('Ctrl Pts',(-57.7412168121408,-64.1526932557469,
-3.49663991521067));
#37995=CARTESIAN_POINT('Ctrl Pts',(-56.0533102435163,-62.6020431454028,
-3.37972327731938));
#37996=CARTESIAN_POINT('Ctrl Pts',(-55.2932410640001,-60.4396851854566,
-3.2628066394281));
#37997=CARTESIAN_POINT('Ctrl Pts',(-55.6396471861552,-58.1739547673332,
-3.1458900015368));
#37998=CARTESIAN_POINT('Ctrl Pts',(-57.0111892920952,-56.3375258651372,
-3.02897336364551));
#37999=CARTESIAN_POINT('Ctrl Pts',(-59.085213780277,-55.362075677042,-2.91205672575423));
#38000=CARTESIAN_POINT('Ctrl Pts',(-61.3745736614467,-55.477060913893,-2.79514008786294));
#38001=CARTESIAN_POINT('Ctrl Pts',(-62.6847840669602,-56.2625729903977,
-2.71719566260208));
#38002=CARTESIAN_POINT('Ctrl Pts',(-63.2093776838358,-56.7864924158161,
-2.67822344997165));
#38003=CARTESIAN_POINT('Ctrl Pts',(-63.6447653928232,-56.845432093658,-10.3217765500284));
#38004=CARTESIAN_POINT('Ctrl Pts',(-64.1597373181463,-57.44042700498,-10.2828043373979));
#38005=CARTESIAN_POINT('Ctrl Pts',(-64.8922228291855,-58.8869090461189,
-10.2048599121371));
#38006=CARTESIAN_POINT('Ctrl Pts',(-64.8407864206437,-61.3192580797911,
-10.0879432742458));
#38007=CARTESIAN_POINT('Ctrl Pts',(-63.6512385814046,-63.4411601037068,
-9.97102663635448));
#38008=CARTESIAN_POINT('Ctrl Pts',(-61.6033434055365,-64.7542485882237,
-9.8541099984632));
#38009=CARTESIAN_POINT('Ctrl Pts',(-59.1785053032208,-64.9495953231459,
-9.73719336057191));
#38010=CARTESIAN_POINT('Ctrl Pts',(-56.9467968863301,-63.9813810195139,
-9.62027672268061));
#38011=CARTESIAN_POINT('Ctrl Pts',(-55.4328599018113,-62.0771726767518,
-9.50336008478933));
#38012=CARTESIAN_POINT('Ctrl Pts',(-54.9926082153259,-59.6846512610652,
-9.38644344689804));
#38013=CARTESIAN_POINT('Ctrl Pts',(-55.7295383088205,-57.3662615111368,
-9.26952680900675));
#38014=CARTESIAN_POINT('Ctrl Pts',(-57.4704069306292,-55.6670360695589,
-9.15261017111546));
#38015=CARTESIAN_POINT('Ctrl Pts',(-59.8059547500423,-54.9864417469716,
-9.03569353322417));
#38016=CARTESIAN_POINT('Ctrl Pts',(-62.1871205174909,-55.4844798146578,
-8.91877689533288));
#38017=CARTESIAN_POINT('Ctrl Pts',(-64.0541184391152,-57.0440664757651,
-8.80186025744159));
#38018=CARTESIAN_POINT('Ctrl Pts',(-64.9680380187631,-59.2985605645345,
-8.6849436195503));
#38019=CARTESIAN_POINT('Ctrl Pts',(-64.7140268543102,-61.7179550203003,
-8.56802698165901));
#38020=CARTESIAN_POINT('Ctrl Pts',(-63.3518001877586,-63.7334778163903,
-8.45111034376772));
#38021=CARTESIAN_POINT('Ctrl Pts',(-61.2016023758519,-64.8713001659127,
-8.33419370587643));
#38022=CARTESIAN_POINT('Ctrl Pts',(-58.7689212180688,-64.8639362517664,
-8.21727706798514));
#38023=CARTESIAN_POINT('Ctrl Pts',(-56.6256529045023,-63.7131094511532,
-8.10036043009385));
#38024=CARTESIAN_POINT('Ctrl Pts',(-55.2756565485713,-61.689383232071,-7.98344379220256));
#38025=CARTESIAN_POINT('Ctrl Pts',(-55.0363003464836,-59.2684768861445,
-7.86652715431127));
#38026=CARTESIAN_POINT('Ctrl Pts',(-55.9638564502248,-57.0195971508376,
-7.74961051641999));
#38027=CARTESIAN_POINT('Ctrl Pts',(-57.8402620299891,-55.4712613393666,
-7.63269387852869));
#38028=CARTESIAN_POINT('Ctrl Pts',(-60.22440498092,-54.9878319033513,-7.51577724063741));
#38029=CARTESIAN_POINT('Ctrl Pts',(-62.5557779859977,-55.6821679011524,
-7.39886060274612));
#38030=CARTESIAN_POINT('Ctrl Pts',(-64.2863481104043,-57.3927447221366,
-7.28194396485483));
#38031=CARTESIAN_POINT('Ctrl Pts',(-65.0091766647164,-59.7137431220925,
-7.16502732696354));
#38032=CARTESIAN_POINT('Ctrl Pts',(-64.5545552909801,-62.1074819348455,
-7.04811068907225));
#38033=CARTESIAN_POINT('Ctrl Pts',(-63.0289060103307,-63.9940847044025,
-6.93119405118096));
#38034=CARTESIAN_POINT('Ctrl Pts',(-60.046045467779,-65.2913881030008,-6.77530520065924));
#38035=CARTESIAN_POINT('Ctrl Pts',(-55.8593833636781,-63.868788301284,-6.58044413750708));
#38036=CARTESIAN_POINT('Ctrl Pts',(-54.484381914806,-58.6999283914272,-6.34661086172452));
#38037=CARTESIAN_POINT('Ctrl Pts',(-57.4108179045277,-55.3851279196312,
-6.15174979857236));
#38038=CARTESIAN_POINT('Ctrl Pts',(-60.6440092141352,-55.0288596501941,
-5.99586094805064));
#38039=CARTESIAN_POINT('Ctrl Pts',(-62.9054039041467,-55.9080466573944,
-5.87894431015935));
#38040=CARTESIAN_POINT('Ctrl Pts',(-64.4893165042581,-57.7595020234115,
-5.76202767226806));
#38041=CARTESIAN_POINT('Ctrl Pts',(-65.0152671842702,-60.1328731645767,
-5.64511103437677));
#38042=CARTESIAN_POINT('Ctrl Pts',(-64.3633743225495,-62.4772241862465,
-5.52819439648548));
#38043=CARTESIAN_POINT('Ctrl Pts',(-62.6851489321296,-64.2381790708658,
-5.41127775859419));
#38044=CARTESIAN_POINT('Ctrl Pts',(-60.3759301040322,-65.0032607879604,
-5.2943611207029));
#38045=CARTESIAN_POINT('Ctrl Pts',(-57.9782160003419,-64.5919108611403,
-5.17744448281161));
#38046=CARTESIAN_POINT('Ctrl Pts',(-56.0558556979054,-63.1011555974462,
-5.06052784492032));
#38047=CARTESIAN_POINT('Ctrl Pts',(-55.0606946858144,-60.8813057177822,
-4.94361120702903));
#38048=CARTESIAN_POINT('Ctrl Pts',(-55.2267214124163,-58.454292512833,-4.82669456913775));
#38049=CARTESIAN_POINT('Ctrl Pts',(-56.5148876417024,-56.3906478851065,
-4.70977793124645));
#38050=CARTESIAN_POINT('Ctrl Pts',(-58.6223677251179,-55.1755266731783,
-4.59286129335517));
#38051=CARTESIAN_POINT('Ctrl Pts',(-61.0537127213995,-55.0945835453589,
-4.47594465546388));
#38052=CARTESIAN_POINT('Ctrl Pts',(-63.2373420963845,-56.1668505277811,
-4.35902801757259));
#38053=CARTESIAN_POINT('Ctrl Pts',(-64.6599078684769,-58.1402480264261,
-4.2421113796813));
#38054=CARTESIAN_POINT('Ctrl Pts',(-64.9869811625584,-60.5508528762455,
-4.12519474179001));
#38055=CARTESIAN_POINT('Ctrl Pts',(-64.141670021687,-62.8319581328956,-4.00827810389872));
#38056=CARTESIAN_POINT('Ctrl Pts',(-62.3226988446208,-64.4473016099512,
-3.89136146600743));
#38057=CARTESIAN_POINT('Ctrl Pts',(-59.9576853524099,-65.0171333210163,
-3.77444482811614));
#38058=CARTESIAN_POINT('Ctrl Pts',(-57.6026228492013,-64.4074933703747,
-3.65752819022485));
#38059=CARTESIAN_POINT('Ctrl Pts',(-55.8111500500176,-62.7616987835354,
-3.54061155233356));
#38060=CARTESIAN_POINT('Ctrl Pts',(-55.0044446991931,-60.466663300322,-3.42369491444227));
#38061=CARTESIAN_POINT('Ctrl Pts',(-55.3721055382745,-58.0619126525068,
-3.30677827655098));
#38062=CARTESIAN_POINT('Ctrl Pts',(-56.8278024479258,-56.1128045163852,
-3.18986163865969));
#38063=CARTESIAN_POINT('Ctrl Pts',(-59.029084512043,-55.0775028525288,-3.0729450007684));
#38064=CARTESIAN_POINT('Ctrl Pts',(-61.4589144747288,-55.1995433303345,
-2.95602836287711));
#38065=CARTESIAN_POINT('Ctrl Pts',(-62.8495165058577,-56.0332526982856,
-2.87808393761625));
#38066=CARTESIAN_POINT('Ctrl Pts',(-63.4062980319963,-56.5893186660636,
-2.83911172498582));
#38067=CARTESIAN_POINT('Ctrl Pts',(-63.8554716972558,-56.6630644309997,
-10.4826648250425));
#38068=CARTESIAN_POINT('Ctrl Pts',(-64.4002144910922,-57.2924563927238,
-10.4436926124121));
#38069=CARTESIAN_POINT('Ctrl Pts',(-65.1750454752818,-58.8225605199143,
-10.3657481871512));
#38070=CARTESIAN_POINT('Ctrl Pts',(-65.1206354938515,-61.3955252642669,
-10.24883154926));
#38071=CARTESIAN_POINT('Ctrl Pts',(-63.8623191051618,-63.6400958513521,
-10.1319149113687));
#38072=CARTESIAN_POINT('Ctrl Pts',(-61.6960337510886,-65.0290948519505,
-10.0149982734774));
#38073=CARTESIAN_POINT('Ctrl Pts',(-59.131014150015,-65.2357347111654,-9.89808163558608));
#38074=CARTESIAN_POINT('Ctrl Pts',(-56.7702891895575,-64.2115472965565,
-9.78116499769479));
#38075=CARTESIAN_POINT('Ctrl Pts',(-55.1688305039767,-62.1972554066989,
-9.6642483598035));
#38076=CARTESIAN_POINT('Ctrl Pts',(-54.703127575537,-59.6664207413398,-9.54733172191222));
#38077=CARTESIAN_POINT('Ctrl Pts',(-55.4826600864412,-57.2140033424977,
-9.43041508402093));
#38078=CARTESIAN_POINT('Ctrl Pts',(-57.3241694777564,-55.4165445512788,
-9.31349844612963));
#38079=CARTESIAN_POINT('Ctrl Pts',(-59.7947368654586,-54.6966046195577,
-9.19658180823835));
#38080=CARTESIAN_POINT('Ctrl Pts',(-62.3135594050244,-55.2234345982174,
-9.07966517034706));
#38081=CARTESIAN_POINT('Ctrl Pts',(-64.2884897146217,-56.8731819984634,
-8.96274853245577));
#38082=CARTESIAN_POINT('Ctrl Pts',(-65.2552435912467,-59.2580098856016,
-8.84583189456447));
#38083=CARTESIAN_POINT('Ctrl Pts',(-64.986547872926,-61.817271139308,-8.72891525667319));
#38084=CARTESIAN_POINT('Ctrl Pts',(-63.5455699794028,-63.9493126448601,
-8.6119986187819));
#38085=CARTESIAN_POINT('Ctrl Pts',(-61.2710678060581,-65.1529132589701,
-8.49508198089061));
#38086=CARTESIAN_POINT('Ctrl Pts',(-58.6977517372794,-65.1451236320635,
-8.37816534299932));
#38087=CARTESIAN_POINT('Ctrl Pts',(-56.4305796611695,-63.9277667709211,
-8.26124870510803));
#38088=CARTESIAN_POINT('Ctrl Pts',(-55.0025391206345,-61.7870475970534,
-8.14433206721674));
#38089=CARTESIAN_POINT('Ctrl Pts',(-54.7493455777719,-59.2261870498135,
-8.02741542932545));
#38090=CARTESIAN_POINT('Ctrl Pts',(-55.7305243149913,-56.8472980856346,
-7.91049879143416));
#38091=CARTESIAN_POINT('Ctrl Pts',(-57.7154061456845,-55.2094519541036,
-7.79358215354287));
#38092=CARTESIAN_POINT('Ctrl Pts',(-60.2373779816841,-54.6980751417997,
-7.67666551565158));
#38093=CARTESIAN_POINT('Ctrl Pts',(-62.7035292062656,-55.4325511640916,
-7.55974887776029));
#38094=CARTESIAN_POINT('Ctrl Pts',(-64.5341447372141,-57.2420175654881,
-7.442832239869));
#38095=CARTESIAN_POINT('Ctrl Pts',(-65.2987604896043,-59.6971944221457,
-7.32591560197771));
#38096=CARTESIAN_POINT('Ctrl Pts',(-64.8178571527642,-62.229316863103,-7.20899896408642));
#38097=CARTESIAN_POINT('Ctrl Pts',(-63.2040090754463,-64.2249853898932,
-7.09208232619513));
#38098=CARTESIAN_POINT('Ctrl Pts',(-60.048707386807,-65.597286758288,-6.93619347567342));
#38099=CARTESIAN_POINT('Ctrl Pts',(-55.6200115700286,-64.0924455186184,
-6.74133241252126));
#38100=CARTESIAN_POINT('Ctrl Pts',(-54.1655203755472,-58.6247703895763,
-6.50749913673869));
#38101=CARTESIAN_POINT('Ctrl Pts',(-57.2611355705387,-55.1183391042526,
-6.31263807358654));
#38102=CARTESIAN_POINT('Ctrl Pts',(-60.6812398138874,-54.7414747298955,
-6.15674922306482));
#38103=CARTESIAN_POINT('Ctrl Pts',(-63.0733672306018,-55.6714881210263,
-6.03983258517353));
#38104=CARTESIAN_POINT('Ctrl Pts',(-64.7488468685178,-57.6299773495695,
-5.92291594728224));
#38105=CARTESIAN_POINT('Ctrl Pts',(-65.3052031061324,-60.1405546503375,
-5.80599930939095));
#38106=CARTESIAN_POINT('Ctrl Pts',(-64.6156238857644,-62.6204341592567,
-5.68908267149966));
#38107=CARTESIAN_POINT('Ctrl Pts',(-62.8403791725874,-64.4831910135561,
-5.57216603360837));
#38108=CARTESIAN_POINT('Ctrl Pts',(-60.3976628726492,-65.2925026120897,
-5.45524939571708));
#38109=CARTESIAN_POINT('Ctrl Pts',(-57.8613353265494,-64.8573722732082,
-5.33833275782579));
#38110=CARTESIAN_POINT('Ctrl Pts',(-55.8278421001908,-63.2804354591061,
-5.2214161199345));
#38111=CARTESIAN_POINT('Ctrl Pts',(-54.7751501700368,-60.9322545857766,
-5.10449948204321));
#38112=CARTESIAN_POINT('Ctrl Pts',(-54.9507750118064,-58.3649341379439,
-4.98758284415192));
#38113=CARTESIAN_POINT('Ctrl Pts',(-56.3134109850716,-56.1819888457558,
-4.87066620626063));
#38114=CARTESIAN_POINT('Ctrl Pts',(-58.5427258897122,-54.8966206707426,
-4.75374956836934));
#38115=CARTESIAN_POINT('Ctrl Pts',(-61.1146285526069,-54.8109981670255,
-4.63683293047805));
#38116=CARTESIAN_POINT('Ctrl Pts',(-63.424494989862,-55.9452536147892,-4.51991629258676));
#38117=CARTESIAN_POINT('Ctrl Pts',(-64.9293002326319,-58.0327345315151,
-4.40299965469548));
#38118=CARTESIAN_POINT('Ctrl Pts',(-65.2752818507472,-60.5826980463265,
-4.28608301680418));
#38119=CARTESIAN_POINT('Ctrl Pts',(-64.381102712243,-62.9956755106081,-4.16916637891289));
#38120=CARTESIAN_POINT('Ctrl Pts',(-62.4569756051562,-64.7044030653083,
-4.0522497410216));
#38121=CARTESIAN_POINT('Ctrl Pts',(-59.9552391145712,-65.3071771254814,
-3.93533310313031));
#38122=CARTESIAN_POINT('Ctrl Pts',(-57.4640288862619,-64.6622934850025,
-3.81841646523903));
#38123=CARTESIAN_POINT('Ctrl Pts',(-55.5689898565188,-62.921354421668,-3.70149982734774));
#38124=CARTESIAN_POINT('Ctrl Pts',(-54.7156483343861,-60.4936414151875,
-3.58458318945645));
#38125=CARTESIAN_POINT('Ctrl Pts',(-55.1045638903938,-57.9498705376805,
-3.46766655156516));
#38126=CARTESIAN_POINT('Ctrl Pts',(-56.6444156037563,-55.8880831676333,
-3.35074991367387));
#38127=CARTESIAN_POINT('Ctrl Pts',(-58.972955243809,-54.7929300280156,-3.23383327578258));
#38128=CARTESIAN_POINT('Ctrl Pts',(-61.543255288011,-54.9220257467759,-3.11691663789129));
#38129=CARTESIAN_POINT('Ctrl Pts',(-63.0142489447553,-55.8039324061734,
-3.03897221263043));
#38130=CARTESIAN_POINT('Ctrl Pts',(-63.6032183801568,-56.3921449163111,
-3.));
#38131=CARTESIAN_POINT('Ctrl Pts',(-63.2233527839579,-57.2101674189746,
-10.));
#38132=CARTESIAN_POINT('Ctrl Pts',(-63.3163082537287,-57.298636481893,-10.));
#38133=CARTESIAN_POINT('Ctrl Pts',(-63.4049730938493,-57.3912022376077,
-10.));
#38134=CARTESIAN_POINT('Ctrl Pts',(-63.4892289732812,-57.487446019035,-10.));
#38135=CARTESIAN_POINT('Ctrl Pts',(-63.575043820607,-57.5854705778544,-10.));
#38136=CARTESIAN_POINT('Ctrl Pts',(-63.6562855651475,-57.6873109425664,
-10.));
#38137=CARTESIAN_POINT('Ctrl Pts',(-63.7328062531653,-57.7925737185367,
-10.));
#38138=CARTESIAN_POINT('Ctrl Pts',(-63.8104264609581,-57.8993490070937,
-10.));
#38139=CARTESIAN_POINT('Ctrl Pts',(-63.8831895396106,-58.0096462773425,
-10.));
#38140=CARTESIAN_POINT('Ctrl Pts',(-63.9509093234047,-58.1230977274475,
-10.));
#38141=CARTESIAN_POINT('Ctrl Pts',(-64.0184811880466,-58.2363013675129,
-10.));
#38142=CARTESIAN_POINT('Ctrl Pts',(-64.0810322758665,-58.3526460671589,
-10.));
#38143=CARTESIAN_POINT('Ctrl Pts',(-64.138338222228,-58.4717998619651,-10.));
#38144=CARTESIAN_POINT('Ctrl Pts',(-64.1498927790088,-58.4958247559796,
-10.));
#38145=CARTESIAN_POINT('Ctrl Pts',(-64.1612339549976,-58.5199639426201,
-10.));
#38146=CARTESIAN_POINT('Ctrl Pts',(-64.1723596873146,-58.5442148295044,
-10.));
#38147=CARTESIAN_POINT('Ctrl Pts',(-64.182565209477,-58.5664599237149,-10.));
#38148=CARTESIAN_POINT('Ctrl Pts',(-64.1925913312984,-58.5888035036185,
-10.));
#38149=CARTESIAN_POINT('Ctrl Pts',(-64.2024245248804,-58.6112158820566,
-10.));
#38150=CARTESIAN_POINT('Ctrl Pts',(-64.2596370057899,-58.7416178478921,
-10.));
#38151=CARTESIAN_POINT('Ctrl Pts',(-64.3103966435791,-58.8745017637267,
-10.));
#38152=CARTESIAN_POINT('Ctrl Pts',(-64.3545198337919,-59.0093933578834,
-10.));
#38153=CARTESIAN_POINT('Ctrl Pts',(-64.3960229534372,-59.1362749805502,
-10.));
#38154=CARTESIAN_POINT('Ctrl Pts',(-64.4316549185973,-59.2649338691195,
-10.));
#38155=CARTESIAN_POINT('Ctrl Pts',(-64.4614760968299,-59.39494826094,-10.));
#38156=CARTESIAN_POINT('Ctrl Pts',(-64.491676772499,-59.5266171859255,-10.));
#38157=CARTESIAN_POINT('Ctrl Pts',(-64.5159180688999,-59.6596770266619,
-10.));
#38158=CARTESIAN_POINT('Ctrl Pts',(-64.5342156697401,-59.7937149390323,
-10.));
#38159=CARTESIAN_POINT('Ctrl Pts',(-64.5504251659969,-59.9124565739497,
-10.));
#38160=CARTESIAN_POINT('Ctrl Pts',(-64.5619695449417,-60.0319664972129,
-10.));
#38161=CARTESIAN_POINT('Ctrl Pts',(-64.5688272622564,-60.1519670666326,
-10.));
#38162=CARTESIAN_POINT('Ctrl Pts',(-64.570543909647,-60.182006022003,-10.));
#38163=CARTESIAN_POINT('Ctrl Pts',(-64.5719667292107,-60.2120757463558,
-10.));
#38164=CARTESIAN_POINT('Ctrl Pts',(-64.5730950735929,-60.2421719198664,
-10.));
#38165=CARTESIAN_POINT('Ctrl Pts',(-64.5739024340997,-60.2637065349035,
-10.));
#38166=CARTESIAN_POINT('Ctrl Pts',(-64.5745589909509,-60.2852564219846,
-10.));
#38167=CARTESIAN_POINT('Ctrl Pts',(-64.5750641911246,-60.3067984108421,
-10.));
#38168=CARTESIAN_POINT('Ctrl Pts',(-64.5783094538577,-60.4451780418628,
-10.));
#38169=CARTESIAN_POINT('Ctrl Pts',(-64.5753216877452,-60.5834277992512,
-10.));
#38170=CARTESIAN_POINT('Ctrl Pts',(-64.5661669987375,-60.721106961686,-10.));
#38171=CARTESIAN_POINT('Ctrl Pts',(-64.5569093304397,-60.8603348498496,
-10.));
#38172=CARTESIAN_POINT('Ctrl Pts',(-64.5413454334492,-60.9989800078359,
-10.));
#38173=CARTESIAN_POINT('Ctrl Pts',(-64.5194941721477,-61.1366051442133,
-10.));
#38174=CARTESIAN_POINT('Ctrl Pts',(-64.5146774260464,-61.1669423101068,
-10.));
#38175=CARTESIAN_POINT('Ctrl Pts',(-64.5095549756123,-61.1972299566409,
-10.));
#38176=CARTESIAN_POINT('Ctrl Pts',(-64.5041266879631,-61.2274634597029,
-10.));
#38177=CARTESIAN_POINT('Ctrl Pts',(-64.4796518086955,-61.3637792530247,
-10.));
#38178=CARTESIAN_POINT('Ctrl Pts',(-64.4489637718321,-61.4989945357919,
-10.));
#38179=CARTESIAN_POINT('Ctrl Pts',(-64.4122747073138,-61.6327571482726,
-10.));
#38180=CARTESIAN_POINT('Ctrl Pts',(-64.3910362736552,-61.7101891680984,
-10.));
#38181=CARTESIAN_POINT('Ctrl Pts',(-64.3677859193463,-61.7871343917435,
-10.));
#38182=CARTESIAN_POINT('Ctrl Pts',(-64.3425569349254,-61.8635234393916,
-10.));
#38183=CARTESIAN_POINT('Ctrl Pts',(-64.3288269090093,-61.9050956083867,
-10.));
#38184=CARTESIAN_POINT('Ctrl Pts',(-64.3145107713356,-61.9465030334659,
-10.));
#38185=CARTESIAN_POINT('Ctrl Pts',(-64.2996131993035,-61.9877343379993,
-10.));
#38186=CARTESIAN_POINT('Ctrl Pts',(-64.2935454976476,-62.0045276284934,
-10.));
#38187=CARTESIAN_POINT('Ctrl Pts',(-64.2873813369501,-62.0212917006638,
-10.));
#38188=CARTESIAN_POINT('Ctrl Pts',(-64.2811210106928,-62.0380257775647,
-10.));
#38189=CARTESIAN_POINT('Ctrl Pts',(-64.2745734824793,-62.0555275556084,
-10.));
#38190=CARTESIAN_POINT('Ctrl Pts',(-64.2679239993545,-62.0729878447327,
-10.));
#38191=CARTESIAN_POINT('Ctrl Pts',(-64.2611741070867,-62.0904035730928,
-10.));
#38192=CARTESIAN_POINT('Ctrl Pts',(-64.2098991667657,-62.2227005634568,
-10.));
#38193=CARTESIAN_POINT('Ctrl Pts',(-64.1528186317814,-62.352468261667,-10.));
#38194=CARTESIAN_POINT('Ctrl Pts',(-64.090210802814,-62.4793487889625,-10.));
#38195=CARTESIAN_POINT('Ctrl Pts',(-64.0269891380834,-62.6074733109243,
-10.));
#38196=CARTESIAN_POINT('Ctrl Pts',(-63.9581310871743,-62.7326545166747,
-10.));
#38197=CARTESIAN_POINT('Ctrl Pts',(-63.8838698879073,-62.8545209615278,
-10.));
#38198=CARTESIAN_POINT('Ctrl Pts',(-63.8095390814517,-62.976501635355,-10.));
#38199=CARTESIAN_POINT('Ctrl Pts',(-63.7297947366439,-63.0951621008321,
-10.));
#38200=CARTESIAN_POINT('Ctrl Pts',(-63.6448209579058,-63.2101155285558,
-10.));
#38201=CARTESIAN_POINT('Ctrl Pts',(-63.6122160490883,-63.2542237944803,
-10.));
#38202=CARTESIAN_POINT('Ctrl Pts',(-63.5788407107611,-63.2977860624708,
-10.));
#38203=CARTESIAN_POINT('Ctrl Pts',(-63.5447035224235,-63.3407795482112,
-10.));
#38204=CARTESIAN_POINT('Ctrl Pts',(-63.481542259528,-63.4203268978285,-10.));
#38205=CARTESIAN_POINT('Ctrl Pts',(-63.415773551013,-63.4979276395244,-10.));
#38206=CARTESIAN_POINT('Ctrl Pts',(-63.3475133975382,-63.573497256696,-10.));
#38207=CARTESIAN_POINT('Ctrl Pts',(-63.3334676325742,-63.589047076425,-10.));
#38208=CARTESIAN_POINT('Ctrl Pts',(-63.3193163436957,-63.6045108685033,
-10.));
#38209=CARTESIAN_POINT('Ctrl Pts',(-63.3050604888266,-63.6198878504331,
-10.));
#38210=CARTESIAN_POINT('Ctrl Pts',(-63.2906483457391,-63.635433411598,-10.));
#38211=CARTESIAN_POINT('Ctrl Pts',(-63.2761359992246,-63.6508830429282,
-10.));
#38212=CARTESIAN_POINT('Ctrl Pts',(-63.2615262241673,-63.66623462277,-10.));
#38213=CARTESIAN_POINT('Ctrl Pts',(-63.1618951272996,-63.7709244439543,
-10.));
#38214=CARTESIAN_POINT('Ctrl Pts',(-63.0577151953492,-63.8710796986466,
-10.));
#38215=CARTESIAN_POINT('Ctrl Pts',(-62.9493854968739,-63.9665039076976,
-10.));
#38216=CARTESIAN_POINT('Ctrl Pts',(-62.8507323508008,-64.0534043474378,
-10.));
#38217=CARTESIAN_POINT('Ctrl Pts',(-62.7486367875531,-64.1363812377739,
-10.));
#38218=CARTESIAN_POINT('Ctrl Pts',(-62.6433691057641,-64.2152667242994,
-10.));
#38219=CARTESIAN_POINT('Ctrl Pts',(-62.5878604519608,-64.256863794618,-10.));
#38220=CARTESIAN_POINT('Ctrl Pts',(-62.5314693108184,-64.297322886992,-10.));
#38221=CARTESIAN_POINT('Ctrl Pts',(-62.4742324962258,-64.3366168410067,
-10.));
#38222=CARTESIAN_POINT('Ctrl Pts',(-62.4525293526399,-64.3515163830604,
-10.));
#38223=CARTESIAN_POINT('Ctrl Pts',(-62.4307046009612,-64.366248383477,-10.));
#38224=CARTESIAN_POINT('Ctrl Pts',(-62.4087601835023,-64.3808112872915,
-10.));
#38225=CARTESIAN_POINT('Ctrl Pts',(-62.3869960059937,-64.3952545790422,
-10.));
#38226=CARTESIAN_POINT('Ctrl Pts',(-62.3651201351428,-64.4095275023171,
-10.));
#38227=CARTESIAN_POINT('Ctrl Pts',(-62.3431409677063,-64.4236248482937,
-10.));
#38228=CARTESIAN_POINT('Ctrl Pts',(-62.2178094000758,-64.5040119910634,
-10.));
#38229=CARTESIAN_POINT('Ctrl Pts',(-62.0890600530759,-64.5787341474093,
-10.));
#38230=CARTESIAN_POINT('Ctrl Pts',(-61.9572867191326,-64.6475637787053,
-10.));
#38231=CARTESIAN_POINT('Ctrl Pts',(-61.8473201863352,-64.7050029864785,
-10.));
#38232=CARTESIAN_POINT('Ctrl Pts',(-61.7352467477612,-64.7583382089978,
-10.));
#38233=CARTESIAN_POINT('Ctrl Pts',(-61.6212758651111,-64.8074173245507,
-10.));
#38234=CARTESIAN_POINT('Ctrl Pts',(-61.5232159544034,-64.8496447213806,
-10.));
#38235=CARTESIAN_POINT('Ctrl Pts',(-61.4237510374481,-64.8887212067715,
-10.));
#38236=CARTESIAN_POINT('Ctrl Pts',(-61.3230392926944,-64.9246350552985,
-10.));
#38237=CARTESIAN_POINT('Ctrl Pts',(-55.7371269462215,-59.9999021904687,
-7.57968167058906));
#38238=CARTESIAN_POINT('Ctrl Pts',(-55.7375457064891,-60.487939361417,-7.60701019445078));
#38239=CARTESIAN_POINT('Ctrl Pts',(-55.8213219914856,-60.9761189733716,
-7.63433871831249));
#38240=CARTESIAN_POINT('Ctrl Pts',(-55.9855958154758,-61.4355115631413,
-7.66166724217421));
#38241=CARTESIAN_POINT('Ctrl Pts',(-56.2198607333526,-62.0906346052765,
-7.70063945480464));
#38242=CARTESIAN_POINT('Ctrl Pts',(-56.6178300622603,-62.6872147084469,
-7.73961166743507));
#38243=CARTESIAN_POINT('Ctrl Pts',(-57.1327248581274,-63.1551325399579,
-7.7785838800655));
#38244=CARTESIAN_POINT('Ctrl Pts',(-57.6476196539944,-63.6230503714689,
-7.81755609269593));
#38245=CARTESIAN_POINT('Ctrl Pts',(-58.2794399168209,-63.9623059313205,
-7.85652830532636));
#38246=CARTESIAN_POINT('Ctrl Pts',(-58.9539186041995,-64.1330191260173,
-7.89550051795679));
#38247=CARTESIAN_POINT('Ctrl Pts',(-59.6283972915781,-64.3037323207141,
-7.93447273058722));
#38248=CARTESIAN_POINT('Ctrl Pts',(-60.3455344035087,-64.305903150256,-7.97344494321765));
#38249=CARTESIAN_POINT('Ctrl Pts',(-61.0210344743125,-64.1392775949691,
-8.01241715584808));
#38250=CARTESIAN_POINT('Ctrl Pts',(-61.6965345451164,-63.9726520396822,
-8.05138936847851));
#38251=CARTESIAN_POINT('Ctrl Pts',(-62.3303975747933,-63.6372300995664,
-8.09036158110894));
#38252=CARTESIAN_POINT('Ctrl Pts',(-62.8481164583998,-63.1724382333142,
-8.12933379373937));
#38253=CARTESIAN_POINT('Ctrl Pts',(-63.3658353420063,-62.707646367062,-8.1683060063698));
#38254=CARTESIAN_POINT('Ctrl Pts',(-63.7674100795425,-62.1134845746734,
-8.20727821900023));
#38255=CARTESIAN_POINT('Ctrl Pts',(-64.0056377910967,-61.459793535165,-8.24625043163066));
#38256=CARTESIAN_POINT('Ctrl Pts',(-64.243865502651,-60.8061024956567,-8.28522264426109));
#38257=CARTESIAN_POINT('Ctrl Pts',(-64.3187461882234,-60.0928822090285,
-8.32419485689152));
#38258=CARTESIAN_POINT('Ctrl Pts',(-64.221478033394,-59.4039676503758,-8.36316706952195));
#38259=CARTESIAN_POINT('Ctrl Pts',(-64.1242098785646,-58.7150530917231,
-8.40213928215238));
#38260=CARTESIAN_POINT('Ctrl Pts',(-63.8547928833333,-58.0504442610459,
-8.4411114947828));
#38261=CARTESIAN_POINT('Ctrl Pts',(-63.4448955281047,-57.4882623152356,
-8.48008370741324));
#38262=CARTESIAN_POINT('Ctrl Pts',(-63.034998172876,-56.9260803694254,-8.51905592004366));
#38263=CARTESIAN_POINT('Ctrl Pts',(-62.4846204576499,-56.4663253084821,
-8.5580281326741));
#38264=CARTESIAN_POINT('Ctrl Pts',(-61.8584562295012,-56.1630387370539,
-8.59700034530453));
#38265=CARTESIAN_POINT('Ctrl Pts',(-61.2322920013524,-55.8597521656257,
-8.63597255793496));
#38266=CARTESIAN_POINT('Ctrl Pts',(-60.530341260281,-55.7129340837125,-8.67494477056539));
#38267=CARTESIAN_POINT('Ctrl Pts',(-59.8351144426062,-55.7398422268092,
-8.71391698319581));
#38268=CARTESIAN_POINT('Ctrl Pts',(-59.1398876249314,-55.7667503699059,
-8.75288919582624));
#38269=CARTESIAN_POINT('Ctrl Pts',(-58.4513847306531,-55.9673847380125,
-8.79186140845667));
#38270=CARTESIAN_POINT('Ctrl Pts',(-57.8505354363813,-56.3181617124484,
-8.8308336210871));
#38271=CARTESIAN_POINT('Ctrl Pts',(-57.2496861421095,-56.6689386868844,
-8.86980583371754));
#38272=CARTESIAN_POINT('Ctrl Pts',(-56.7364904478442,-57.1698582676496,
-8.90877804634796));
#38273=CARTESIAN_POINT('Ctrl Pts',(-56.3712717242657,-57.7620404667158,
-8.94775025897839));
#38274=CARTESIAN_POINT('Ctrl Pts',(-56.0060530006872,-58.354222665782,-8.98672247160882));
#38275=CARTESIAN_POINT('Ctrl Pts',(-55.7888112477955,-59.037667483149,-9.02569468423925));
#38276=CARTESIAN_POINT('Ctrl Pts',(-55.7450819051124,-59.7320390445562,
-9.06466689686969));
#38277=CARTESIAN_POINT('Ctrl Pts',(-55.7394660561013,-59.8212122542869,
-9.06967182144281));
#38278=CARTESIAN_POINT('Ctrl Pts',(-55.7367118503295,-59.9105656727024,
-9.07467674601594));
#38279=CARTESIAN_POINT('Ctrl Pts',(-55.7367869775695,-59.9999237120217,
-9.07968167058906));
#38280=CARTESIAN_POINT('Ctrl Pts',(-58.677115034431,-64.9244061944433,-10.));
#38281=CARTESIAN_POINT('Ctrl Pts',(-57.8732233401272,-64.7084499564018,
-9.96102778736957));
#38282=CARTESIAN_POINT('Ctrl Pts',(-56.3739727010425,-63.8754866332611,
-9.88308336210871));
#38283=CARTESIAN_POINT('Ctrl Pts',(-54.9770228002682,-61.7140882090784,
-9.76616672421742));
#38284=CARTESIAN_POINT('Ctrl Pts',(-54.7611834296551,-59.14993732374,-9.64925008632613));
#38285=CARTESIAN_POINT('Ctrl Pts',(-55.7768178205809,-56.785492732961,-9.53233344843484));
#38286=CARTESIAN_POINT('Ctrl Pts',(-57.7853302129478,-55.1767966332062,
-9.41541681054355));
#38287=CARTESIAN_POINT('Ctrl Pts',(-60.3144620635955,-54.7019555263241,
-9.29850017265227));
#38288=CARTESIAN_POINT('Ctrl Pts',(-62.7696789900454,-55.4726379404574,
-9.18158353476098));
#38289=CARTESIAN_POINT('Ctrl Pts',(-64.5737696881318,-57.3076474190762,
-9.06466689686968));
#38290=CARTESIAN_POINT('Ctrl Pts',(-65.3026202647668,-59.7756017648733,
-8.9477502589784));
#38291=CARTESIAN_POINT('Ctrl Pts',(-64.7848823729,-62.2963084445819,-8.8308336210871));
#38292=CARTESIAN_POINT('Ctrl Pts',(-63.1422721548051,-64.2771789992941,
-8.71391698319582));
#38293=CARTESIAN_POINT('Ctrl Pts',(-60.7609482822248,-65.252531849864,-8.59700034530452));
#38294=CARTESIAN_POINT('Ctrl Pts',(-58.2007340409931,-64.9930727838061,
-8.48008370741324));
#38295=CARTESIAN_POINT('Ctrl Pts',(-56.0635071815643,-63.5597974366436,
-8.36316706952195));
#38296=CARTESIAN_POINT('Ctrl Pts',(-54.8517063751933,-61.2896533639402,
-8.24625043163066));
#38297=CARTESIAN_POINT('Ctrl Pts',(-54.8502120579674,-58.7163255954642,
-8.12933379373937));
#38298=CARTESIAN_POINT('Ctrl Pts',(-56.0593765808925,-56.444776458995,-8.01241715584808));
#38299=CARTESIAN_POINT('Ctrl Pts',(-58.1949365065413,-55.009018880156,-7.89550051795679));
#38300=CARTESIAN_POINT('Ctrl Pts',(-60.754850176949,-54.7465903023206,-7.7785838800655));
#38301=CARTESIAN_POINT('Ctrl Pts',(-63.1372997996482,-55.7191702494578,
-7.6616672421742));
#38302=CARTESIAN_POINT('Ctrl Pts',(-64.7822203636214,-57.6981473048777,
-7.54475060428292));
#38303=CARTESIAN_POINT('Ctrl Pts',(-65.3028606509933,-60.2182181776382,
-7.42783396639163));
#38304=CARTESIAN_POINT('Ctrl Pts',(-64.5769288134183,-62.6870882382886,
-7.31091732850035));
#38305=CARTESIAN_POINT('Ctrl Pts',(-62.7748568790513,-64.5240380041187,
-7.19400069060905));
#38306=CARTESIAN_POINT('Ctrl Pts',(-60.3207808627358,-65.2979018325692,
-7.07708405271776));
#38307=CARTESIAN_POINT('Ctrl Pts',(-57.7905711249098,-64.8252826799559,
-6.96016741482647));
#38308=CARTESIAN_POINT('Ctrl Pts',(-55.7813289378715,-63.2204602274652,
-6.84325077693518));
#38309=CARTESIAN_POINT('Ctrl Pts',(-54.760481380096,-60.8538559480399,-6.72633413904389));
#38310=CARTESIAN_POINT('Ctrl Pts',(-54.9785971562446,-58.2965966407732,
-6.60941750115261));
#38311=CARTESIAN_POINT('Ctrl Pts',(-56.8226683737146,-55.391675711492,-6.45352865063088));
#38312=CARTESIAN_POINT('Ctrl Pts',(-61.3338598105922,-54.1559235864261,
-6.25866758747874));
#38313=CARTESIAN_POINT('Ctrl Pts',(-65.6028015656481,-57.869031736986,-6.02483431169615));
#38314=CARTESIAN_POINT('Ctrl Pts',(-65.0042219447148,-62.5079576829526,
-5.82997324854401));
#38315=CARTESIAN_POINT('Ctrl Pts',(-62.382923622443,-64.736849642231,-5.67408439802229));
#38316=CARTESIAN_POINT('Ctrl Pts',(-59.8805760101181,-65.3072934023813,
-5.557167760131));
#38317=CARTESIAN_POINT('Ctrl Pts',(-57.3953244921747,-64.6243069865738,
-5.44025112223971));
#38318=CARTESIAN_POINT('Ctrl Pts',(-55.5275122251888,-62.8568832667251,
-5.32333448434841));
#38319=CARTESIAN_POINT('Ctrl Pts',(-54.7087704381597,-60.4165980237737,
-5.20641784645713));
#38320=CARTESIAN_POINT('Ctrl Pts',(-55.135033382092,-57.8789506444978,-5.08950120856584));
#38321=CARTESIAN_POINT('Ctrl Pts',(-56.7044889980166,-55.8396721524265,
-4.97258457067455));
#38322=CARTESIAN_POINT('Ctrl Pts',(-59.0489177395961,-54.7785641063853,
-4.85566793278326));
#38323=CARTESIAN_POINT('Ctrl Pts',(-61.6168265507944,-54.9449006597622,
-4.73875129489197));
#38324=CARTESIAN_POINT('Ctrl Pts',(-63.8046877645853,-56.2996615825733,
-4.62183465700068));
#38325=CARTESIAN_POINT('Ctrl Pts',(-65.0980856519831,-58.5243188288231,
-4.50491801910939));
#38326=CARTESIAN_POINT('Ctrl Pts',(-65.1929908727149,-61.0958980618402,
-4.3880013812181));
#38327=CARTESIAN_POINT('Ctrl Pts',(-64.0670764169607,-63.4098411642031,
-4.27108474332681));
#38328=CARTESIAN_POINT('Ctrl Pts',(-61.9850396640587,-64.922169576908,-4.15416810543552));
#38329=CARTESIAN_POINT('Ctrl Pts',(-59.4363409557176,-65.2773498680853,
-4.03725146754424));
#38330=CARTESIAN_POINT('Ctrl Pts',(-57.0201528179928,-64.3918838717894,
-3.92033482965294));
#38331=CARTESIAN_POINT('Ctrl Pts',(-55.3044933735877,-62.4739345405712,
-3.80341819176166));
#38332=CARTESIAN_POINT('Ctrl Pts',(-54.6926959899439,-59.9743905229704,
-3.68650155387037));
#38333=CARTESIAN_POINT('Ctrl Pts',(-55.3285862434613,-57.4808672502626,
-3.56958491597908));
#38334=CARTESIAN_POINT('Ctrl Pts',(-57.0626757333642,-55.5795636292569,
-3.45266827808779));
#38335=CARTESIAN_POINT('Ctrl Pts',(-59.4872942572559,-54.7174568855574,
-3.3357516401965));
#38336=CARTESIAN_POINT('Ctrl Pts',(-62.032451512693,-55.097214824058,-3.21883500230521));
#38337=CARTESIAN_POINT('Ctrl Pts',(-64.0997862511836,-56.6295689181909,
-3.10191836441392));
#38338=CARTESIAN_POINT('Ctrl Pts',(-65.2033406964322,-58.954260889118,-2.98500172652263));
#38339=CARTESIAN_POINT('Ctrl Pts',(-65.0835748708919,-61.5248187245729,
-2.86808508863134));
#38340=CARTESIAN_POINT('Ctrl Pts',(-63.7688779976231,-63.7368378312184,
-2.75116845074005));
#38341=CARTESIAN_POINT('Ctrl Pts',(-61.5678299178988,-65.0704417919735,
-2.63425181284876));
#38342=CARTESIAN_POINT('Ctrl Pts',(-59.8553056997907,-65.1644693350243,
-2.5563073875879));
#38343=CARTESIAN_POINT('Ctrl Pts',(-59.0378648750817,-65.0074042178956,
-2.51733517495747));
#38344=CARTESIAN_POINT('Ctrl Pts',(-58.7494123365958,-64.655281295538,-10.1608882750142));
#38345=CARTESIAN_POINT('Ctrl Pts',(-57.9894543192508,-64.4511273334331,
-10.1219160623837));
#38346=CARTESIAN_POINT('Ctrl Pts',(-56.5721395848712,-63.6636864877811,
-10.0439716371229));
#38347=CARTESIAN_POINT('Ctrl Pts',(-55.2515347267228,-61.6204111650312,
-9.9270549992316));
#38348=CARTESIAN_POINT('Ctrl Pts',(-55.0474912450966,-59.1963943020595,
-9.81013836134031));
#38349=CARTESIAN_POINT('Ctrl Pts',(-56.0076199583853,-56.9611695372523,
-9.69322172344901));
#38350=CARTESIAN_POINT('Ctrl Pts',(-57.9063646603542,-55.4403906722099,
-9.57630508555773));
#38351=CARTESIAN_POINT('Ctrl Pts',(-60.2972763222628,-54.9915002200545,
-9.45938844766644));
#38352=CARTESIAN_POINT('Ctrl Pts',(-62.6183126021472,-55.7200638855301,
-9.34247180977516));
#38353=CARTESIAN_POINT('Ctrl Pts',(-64.3238075086667,-57.4547878229235,
-9.22555517188386));
#38354=CARTESIAN_POINT('Ctrl Pts',(-65.0128254983848,-59.7878654064087,
-9.10863853399257));
#38355=CARTESIAN_POINT('Ctrl Pts',(-64.5233826236848,-62.1708123434071,
-8.99172189610128));
#38356=CARTESIAN_POINT('Ctrl Pts',(-62.9705430888825,-64.043425868392,-8.87480525820999));
#38357=CARTESIAN_POINT('Ctrl Pts',(-60.7193615159347,-64.9654744774063,
-8.7578886203187));
#38358=CARTESIAN_POINT('Ctrl Pts',(-58.2990661545925,-64.7201951707276,
-8.64097198242741));
#38359=CARTESIAN_POINT('Ctrl Pts',(-56.2786413906388,-63.3652500968363,
-8.52405534453612));
#38360=CARTESIAN_POINT('Ctrl Pts',(-55.1330669995209,-61.2191722099718,
-8.40713870664483));
#38361=CARTESIAN_POINT('Ctrl Pts',(-55.1316543485825,-58.7864799918943,
-8.29022206875355));
#38362=CARTESIAN_POINT('Ctrl Pts',(-56.2747365324107,-56.6390738297396,
-8.17330543086225));
#38363=CARTESIAN_POINT('Ctrl Pts',(-58.2935854625805,-55.2817821812078,
-8.05638879297097));
#38364=CARTESIAN_POINT('Ctrl Pts',(-60.7135966796666,-55.033695650249,-7.93947215507967));
#38365=CARTESIAN_POINT('Ctrl Pts',(-62.9658424790948,-55.9531228984382,
-7.82255551718839));
#38366=CARTESIAN_POINT('Ctrl Pts',(-64.520866096511,-57.8239464062127,-7.7056388792971));
#38367=CARTESIAN_POINT('Ctrl Pts',(-65.0130527472063,-60.2062922839005,
-7.5887222414058));
#38368=CARTESIAN_POINT('Ctrl Pts',(-64.3267939838427,-62.5402355372878,
-7.47180560351452));
#38369=CARTESIAN_POINT('Ctrl Pts',(-62.6232075131046,-64.2767937227928,
-7.35488896562323));
#38370=CARTESIAN_POINT('Ctrl Pts',(-60.3032497912023,-65.008364934352,-7.23797232773194));
#38371=CARTESIAN_POINT('Ctrl Pts',(-57.9113191499851,-64.5615750039121,
-7.12105568984065));
#38372=CARTESIAN_POINT('Ctrl Pts',(-56.0118845375275,-63.044458086512,-7.00413905194936));
#38373=CARTESIAN_POINT('Ctrl Pts',(-55.0468275634157,-60.8071916627186,
-6.88722241405807));
#38374=CARTESIAN_POINT('Ctrl Pts',(-55.2530230421947,-58.3896897445395,
-6.77030577616678));
#38375=CARTESIAN_POINT('Ctrl Pts',(-56.9963134831854,-55.6435263426741,
-6.61441692564506));
#38376=CARTESIAN_POINT('Ctrl Pts',(-61.2609627195511,-54.475309602099,-6.41955586249291));
#38377=CARTESIAN_POINT('Ctrl Pts',(-65.2966015193069,-57.9854917924139,
-6.18572258671033));
#38378=CARTESIAN_POINT('Ctrl Pts',(-64.730735016181,-62.3708946887088,-5.99086152355818));
#38379=CARTESIAN_POINT('Ctrl Pts',(-62.2526938944988,-64.47797494125,-5.83497267303646));
#38380=CARTESIAN_POINT('Ctrl Pts',(-59.8871026791081,-65.0172432432395,
-5.71805603514517));
#38381=CARTESIAN_POINT('Ctrl Pts',(-57.5376732353624,-64.371582881143,-5.60113939725389));
#38382=CARTESIAN_POINT('Ctrl Pts',(-55.7719392226224,-62.7007510570773,
-5.48422275936259));
#38383=CARTESIAN_POINT('Ctrl Pts',(-54.9979426885158,-60.3938304256908,
-5.36730612147131));
#38384=CARTESIAN_POINT('Ctrl Pts',(-55.4009098345056,-57.9948686193426,
-5.25038948358002));
#38385=CARTESIAN_POINT('Ctrl Pts',(-56.8845927567705,-56.0670392231313,
-5.13347284568873));
#38386=CARTESIAN_POINT('Ctrl Pts',(-59.1008955633327,-55.0639220463122,
-5.01655620779744));
#38387=CARTESIAN_POINT('Ctrl Pts',(-61.5284649768607,-55.2211681009885,
-4.89963956990615));
#38388=CARTESIAN_POINT('Ctrl Pts',(-63.5967568649845,-56.5018896610834,
-4.78272293201485));
#38389=CARTESIAN_POINT('Ctrl Pts',(-64.8194689555683,-58.6049666329092,
-4.66580629412357));
#38390=CARTESIAN_POINT('Ctrl Pts',(-64.909187488418,-61.0360058751566,-4.54888965623228));
#38391=CARTESIAN_POINT('Ctrl Pts',(-63.8448056524592,-63.2234891204512,
-4.43197301834099));
#38392=CARTESIAN_POINT('Ctrl Pts',(-61.8765547873409,-64.6531669119217,
-4.3150563804497));
#38393=CARTESIAN_POINT('Ctrl Pts',(-59.4671456207512,-64.9889361601871,
-4.19813974255841));
#38394=CARTESIAN_POINT('Ctrl Pts',(-57.1830051579391,-64.1518619775084,
-4.08122310466712));
#38395=CARTESIAN_POINT('Ctrl Pts',(-55.5611086275382,-62.3387309532065,
-3.96430646677583));
#38396=CARTESIAN_POINT('Ctrl Pts',(-54.9827467288082,-59.9757901126153,
-3.84738982888454));
#38397=CARTESIAN_POINT('Ctrl Pts',(-55.5838847922268,-57.61854097575,-3.73047319099325));
#38398=CARTESIAN_POINT('Ctrl Pts',(-57.2232041433078,-55.8211459529767,
-3.61355655310196));
#38399=CARTESIAN_POINT('Ctrl Pts',(-59.5153142612392,-55.0061544108024,
-3.49663991521067));
#38400=CARTESIAN_POINT('Ctrl Pts',(-61.9213755197133,-55.365158107518,-3.37972327731939));
#38401=CARTESIAN_POINT('Ctrl Pts',(-63.8757278537207,-56.8137671521186,
-3.26280663942809));
#38402=CARTESIAN_POINT('Ctrl Pts',(-64.9189716814477,-59.0114118269946,
-3.14589000153681));
#38403=CARTESIAN_POINT('Ctrl Pts',(-64.8057512066397,-61.441485492322,-3.02897336364551));
#38404=CARTESIAN_POINT('Ctrl Pts',(-63.5629041461481,-63.5326150145289,
-2.91205672575423));
#38405=CARTESIAN_POINT('Ctrl Pts',(-61.4821460706501,-64.7933358667535,
-2.79514008786293));
#38406=CARTESIAN_POINT('Ctrl Pts',(-59.8632134225452,-64.8822246880948,
-2.71719566260207));
#38407=CARTESIAN_POINT('Ctrl Pts',(-59.0904467515563,-64.7337433741902,
-2.67822344997165));
#38408=CARTESIAN_POINT('Ctrl Pts',(-58.8217096387607,-64.3861563966327,
-10.3217765500284));
#38409=CARTESIAN_POINT('Ctrl Pts',(-58.1056852983744,-64.1938047104644,
-10.2828043373979));
#38410=CARTESIAN_POINT('Ctrl Pts',(-56.7703064687,-63.4518863423012,-10.2048599121371));
#38411=CARTESIAN_POINT('Ctrl Pts',(-55.5260466531774,-61.5267341209841,
-10.0879432742458));
#38412=CARTESIAN_POINT('Ctrl Pts',(-55.3337990605381,-59.2428512803789,
-9.97102663635449));
#38413=CARTESIAN_POINT('Ctrl Pts',(-56.2384220961897,-57.1368463415437,
-9.85410999846319));
#38414=CARTESIAN_POINT('Ctrl Pts',(-58.0273991077606,-55.7039847112136,
-9.73719336057191));
#38415=CARTESIAN_POINT('Ctrl Pts',(-60.2800905809301,-55.2810449137848,
-9.62027672268061));
#38416=CARTESIAN_POINT('Ctrl Pts',(-62.4669462142492,-55.9674898306028,
-9.50336008478933));
#38417=CARTESIAN_POINT('Ctrl Pts',(-64.0738453292015,-57.6019282267708,
-9.38644344689803));
#38418=CARTESIAN_POINT('Ctrl Pts',(-64.7230307320029,-59.800129047944,-9.26952680900675));
#38419=CARTESIAN_POINT('Ctrl Pts',(-64.2618828744696,-62.0453162422323,
-9.15261017111546));
#38420=CARTESIAN_POINT('Ctrl Pts',(-62.79881402296,-63.8096727374899,-9.03569353322417));
#38421=CARTESIAN_POINT('Ctrl Pts',(-60.6777747496446,-64.6784171049485,
-8.91877689533288));
#38422=CARTESIAN_POINT('Ctrl Pts',(-58.3973982681919,-64.4473175576491,
-8.80186025744159));
#38423=CARTESIAN_POINT('Ctrl Pts',(-56.4937755997133,-63.1707027570288,
-8.6849436195503));
#38424=CARTESIAN_POINT('Ctrl Pts',(-55.4144276238484,-61.1486910560035,
-8.56802698165901));
#38425=CARTESIAN_POINT('Ctrl Pts',(-55.4130966391976,-58.8566343883245,
-8.45111034376773));
#38426=CARTESIAN_POINT('Ctrl Pts',(-56.4900964839289,-56.8333712004842,
-8.33419370587643));
#38427=CARTESIAN_POINT('Ctrl Pts',(-58.3922344186197,-55.5545454822596,
-8.21727706798514));
#38428=CARTESIAN_POINT('Ctrl Pts',(-60.6723431823842,-55.3208009981773,
-8.10036043009385));
#38429=CARTESIAN_POINT('Ctrl Pts',(-62.7943851585413,-56.1870755474186,
-7.98344379220256));
#38430=CARTESIAN_POINT('Ctrl Pts',(-64.2595118294006,-57.9497455075478,
-7.86652715431127));
#38431=CARTESIAN_POINT('Ctrl Pts',(-64.7232448434193,-60.1943663901628,
-7.74961051641998));
#38432=CARTESIAN_POINT('Ctrl Pts',(-64.0766591542672,-62.393382836287,-7.6326938785287));
#38433=CARTESIAN_POINT('Ctrl Pts',(-62.4715581471579,-64.0295494414668,
-7.51577724063741));
#38434=CARTESIAN_POINT('Ctrl Pts',(-60.2857187196689,-64.7188280361349,
-7.39886060274612));
#38435=CARTESIAN_POINT('Ctrl Pts',(-58.0320671750603,-64.2978673278682,
-7.28194396485483));
#38436=CARTESIAN_POINT('Ctrl Pts',(-56.2424401371836,-62.8684559455588,
-7.16502732696354));
#38437=CARTESIAN_POINT('Ctrl Pts',(-55.3331737467353,-60.7605273773972,
-7.04811068907224));
#38438=CARTESIAN_POINT('Ctrl Pts',(-55.5274489281449,-58.4827828483059,
-6.93119405118096));
#38439=CARTESIAN_POINT('Ctrl Pts',(-57.1699585926562,-55.8953769738562,
-6.77530520065923));
#38440=CARTESIAN_POINT('Ctrl Pts',(-61.18806562851,-54.7946956177719,-6.58044413750709));
#38441=CARTESIAN_POINT('Ctrl Pts',(-64.9904014729656,-58.1019518478416,
-6.3466108617245));
#38442=CARTESIAN_POINT('Ctrl Pts',(-64.4572480876472,-62.233831694465,-6.15174979857236));
#38443=CARTESIAN_POINT('Ctrl Pts',(-62.1224641665546,-64.2191002402691,
-5.99586094805064));
#38444=CARTESIAN_POINT('Ctrl Pts',(-59.8936293480983,-64.7271930840978,
-5.87894431015935));
#38445=CARTESIAN_POINT('Ctrl Pts',(-57.68002197855,-64.1188587757121,-5.76202767226806));
#38446=CARTESIAN_POINT('Ctrl Pts',(-56.016366220056,-62.5446188474295,-5.64511103437677));
#38447=CARTESIAN_POINT('Ctrl Pts',(-55.287114938872,-60.3710628276078,-5.52819439648548));
#38448=CARTESIAN_POINT('Ctrl Pts',(-55.6667862869192,-58.1107865941873,
-5.41127775859419));
#38449=CARTESIAN_POINT('Ctrl Pts',(-57.0646965155244,-56.2944062938361,
-5.2943611207029));
#38450=CARTESIAN_POINT('Ctrl Pts',(-59.1528733870691,-55.3492799862391,
-5.17744448281161));
#38451=CARTESIAN_POINT('Ctrl Pts',(-61.440103402927,-55.4974355422148,-5.06052784492032));
#38452=CARTESIAN_POINT('Ctrl Pts',(-63.3888259653837,-56.7041177395935,
-4.94361120702903));
#38453=CARTESIAN_POINT('Ctrl Pts',(-64.5408522591534,-58.6856144369952,
-4.82669456913774));
#38454=CARTESIAN_POINT('Ctrl Pts',(-64.6253841041211,-60.976113688473,-4.70977793124645));
#38455=CARTESIAN_POINT('Ctrl Pts',(-63.6225348879577,-63.0371370766992,
-4.59286129335517));
#38456=CARTESIAN_POINT('Ctrl Pts',(-61.768069910623,-64.3841642469354,-4.47594465546388));
#38457=CARTESIAN_POINT('Ctrl Pts',(-59.4979502857849,-64.7005224522889,
-4.35902801757259));
#38458=CARTESIAN_POINT('Ctrl Pts',(-57.3458574978853,-63.9118400832274,
-4.2421113796813));
#38459=CARTESIAN_POINT('Ctrl Pts',(-55.8177238814887,-62.2035273658419,
-4.12519474179001));
#38460=CARTESIAN_POINT('Ctrl Pts',(-55.2727974676725,-59.97718970226,-4.00827810389872));
#38461=CARTESIAN_POINT('Ctrl Pts',(-55.8391833409923,-57.7562147012374,
-3.89136146600743));
#38462=CARTESIAN_POINT('Ctrl Pts',(-57.3837325532514,-56.0627282766964,
-3.77444482811614));
#38463=CARTESIAN_POINT('Ctrl Pts',(-59.5433342652227,-55.2948519360475,
-3.65752819022485));
#38464=CARTESIAN_POINT('Ctrl Pts',(-61.8102995267335,-55.633101390978,-3.54061155233356));
#38465=CARTESIAN_POINT('Ctrl Pts',(-63.6516694562579,-56.9979653860463,
-3.42369491444227));
#38466=CARTESIAN_POINT('Ctrl Pts',(-64.6346026664633,-59.0685627648711,
-3.30677827655098));
#38467=CARTESIAN_POINT('Ctrl Pts',(-64.5279275423875,-61.358152260071,-3.18986163865969));
#38468=CARTESIAN_POINT('Ctrl Pts',(-63.3569302946731,-63.3283921978395,
-3.0729450007684));
#38469=CARTESIAN_POINT('Ctrl Pts',(-61.3964622234014,-64.5162299415336,
-2.95602836287711));
#38470=CARTESIAN_POINT('Ctrl Pts',(-59.8711211452996,-64.5999800411654,
-2.87808393761625));
#38471=CARTESIAN_POINT('Ctrl Pts',(-59.1430286280309,-64.4600825304849,
-2.83911172498582));
#38472=CARTESIAN_POINT('Ctrl Pts',(-58.8940069409255,-64.1170314977274,
-10.4826648250425));
#38473=CARTESIAN_POINT('Ctrl Pts',(-58.221916277498,-63.9364820874957,-10.4436926124121));
#38474=CARTESIAN_POINT('Ctrl Pts',(-56.9684733525287,-63.2400861968213,
-10.3657481871512));
#38475=CARTESIAN_POINT('Ctrl Pts',(-55.800558579632,-61.4330570769369,-10.2488315492599));
#38476=CARTESIAN_POINT('Ctrl Pts',(-55.6201068759796,-59.2893082586984,
-10.1319149113687));
#38477=CARTESIAN_POINT('Ctrl Pts',(-56.4692242339942,-57.312523145835,-10.0149982734774));
#38478=CARTESIAN_POINT('Ctrl Pts',(-58.1484335551669,-55.9675787502173,
-9.89808163558608));
#38479=CARTESIAN_POINT('Ctrl Pts',(-60.2629048395975,-55.5705896075151,
-9.78116499769479));
#38480=CARTESIAN_POINT('Ctrl Pts',(-62.3155798263509,-56.2149157756756,
-9.6642483598035));
#38481=CARTESIAN_POINT('Ctrl Pts',(-63.8238831497364,-57.7490686306181,
-9.54733172191221));
#38482=CARTESIAN_POINT('Ctrl Pts',(-64.4332359656209,-59.8123926894793,
-9.43041508402093));
#38483=CARTESIAN_POINT('Ctrl Pts',(-64.0003831252545,-61.9198201410576,
-9.31349844612963));
#38484=CARTESIAN_POINT('Ctrl Pts',(-62.6270849570375,-63.5759196065878,
-9.19658180823835));
#38485=CARTESIAN_POINT('Ctrl Pts',(-60.6361879833545,-64.3913597324907,
-9.07966517034706));
#38486=CARTESIAN_POINT('Ctrl Pts',(-58.4957303817913,-64.1744399445706,
-8.96274853245577));
#38487=CARTESIAN_POINT('Ctrl Pts',(-56.7089098087877,-62.9761554172214,
-8.84583189456448));
#38488=CARTESIAN_POINT('Ctrl Pts',(-55.6957882481759,-61.0782099020351,
-8.72891525667319));
#38489=CARTESIAN_POINT('Ctrl Pts',(-55.6945389298127,-58.9267887847546,
-8.6119986187819));
#38490=CARTESIAN_POINT('Ctrl Pts',(-56.7054564354471,-57.0276685712288,
-8.49508198089061));
#38491=CARTESIAN_POINT('Ctrl Pts',(-58.4908833746589,-55.8273087833114,
-8.37816534299932));
#38492=CARTESIAN_POINT('Ctrl Pts',(-60.6310896851017,-55.6079063461057,
-8.26124870510803));
#38493=CARTESIAN_POINT('Ctrl Pts',(-62.6229278379879,-56.421028196399,-8.14433206721674));
#38494=CARTESIAN_POINT('Ctrl Pts',(-63.9981575622902,-58.0755446088829,
-8.02741542932545));
#38495=CARTESIAN_POINT('Ctrl Pts',(-64.4334369396322,-60.1824404964251,
-7.91049879143416));
#38496=CARTESIAN_POINT('Ctrl Pts',(-63.8265243246915,-62.2465301352862,
-7.79358215354287));
#38497=CARTESIAN_POINT('Ctrl Pts',(-62.3199087812112,-63.7823051601408,
-7.67666551565158));
#38498=CARTESIAN_POINT('Ctrl Pts',(-60.2681876481355,-64.4292911379178,
-7.55974887776029));
#38499=CARTESIAN_POINT('Ctrl Pts',(-58.1528152001354,-64.0341596518243,
-7.442832239869));
#38500=CARTESIAN_POINT('Ctrl Pts',(-56.4729957368398,-62.6924538046056,
-7.32591560197771));
#38501=CARTESIAN_POINT('Ctrl Pts',(-55.6195199300548,-60.7138630920758,
-7.20899896408642));
#38502=CARTESIAN_POINT('Ctrl Pts',(-55.8018748140951,-58.5758759520722,
-7.09208232619513));
#38503=CARTESIAN_POINT('Ctrl Pts',(-57.3436037021269,-56.1472276050383,
-6.93619347567341));
#38504=CARTESIAN_POINT('Ctrl Pts',(-61.115168537469,-55.1140816334448,-6.74133241252127));
#38505=CARTESIAN_POINT('Ctrl Pts',(-64.6842014266244,-58.2184119032695,
-6.50749913673868));
#38506=CARTESIAN_POINT('Ctrl Pts',(-64.1837611591134,-62.0967687002211,
-6.31263807358653));
#38507=CARTESIAN_POINT('Ctrl Pts',(-61.9922344386104,-63.9602255392882,
-6.15674922306482));
#38508=CARTESIAN_POINT('Ctrl Pts',(-59.9001560170883,-64.4371429249561,
-6.03983258517352));
#38509=CARTESIAN_POINT('Ctrl Pts',(-57.8223707217377,-63.8661346702813,
-5.92291594728224));
#38510=CARTESIAN_POINT('Ctrl Pts',(-56.2607932174897,-62.3884866377817,
-5.80599930939095));
#38511=CARTESIAN_POINT('Ctrl Pts',(-55.5762871892282,-60.3482952295248,
-5.68908267149966));
#38512=CARTESIAN_POINT('Ctrl Pts',(-55.9326627393328,-58.226704569032,-5.57216603360837));
#38513=CARTESIAN_POINT('Ctrl Pts',(-57.2448002742782,-56.5217733645409,
-5.45524939571708));
#38514=CARTESIAN_POINT('Ctrl Pts',(-59.2048512108057,-55.634637926166,-5.33833275782579));
#38515=CARTESIAN_POINT('Ctrl Pts',(-61.3517418289932,-55.7737029834411,
-5.2214161199345));
#38516=CARTESIAN_POINT('Ctrl Pts',(-63.1808950657829,-56.9063458181036,
-5.10449948204321));
#38517=CARTESIAN_POINT('Ctrl Pts',(-64.2622355627386,-58.7662622410812,
-4.98758284415192));
#38518=CARTESIAN_POINT('Ctrl Pts',(-64.3415807198242,-60.9162215017895,
-4.87066620626063));
#38519=CARTESIAN_POINT('Ctrl Pts',(-63.4002641234563,-62.8507850329473,
-4.75374956836934));
#38520=CARTESIAN_POINT('Ctrl Pts',(-61.6595850339052,-64.1151615819491,
-4.63683293047805));
#38521=CARTESIAN_POINT('Ctrl Pts',(-59.5287549508186,-64.4121087443906,
-4.51991629258676));
#38522=CARTESIAN_POINT('Ctrl Pts',(-57.5087098378316,-63.6718181889464,
-4.40299965469547));
#38523=CARTESIAN_POINT('Ctrl Pts',(-56.0743391354391,-62.0683237784772,
-4.28608301680418));
#38524=CARTESIAN_POINT('Ctrl Pts',(-55.5628482065368,-59.9785892919048,
-4.1691663789129));
#38525=CARTESIAN_POINT('Ctrl Pts',(-56.0944818897578,-57.8938884267248,
-4.0522497410216));
#38526=CARTESIAN_POINT('Ctrl Pts',(-57.5442609631951,-56.3043106004162,
-3.93533310313032));
#38527=CARTESIAN_POINT('Ctrl Pts',(-59.5713542692061,-55.5835494612926,
-3.81841646523903));
#38528=CARTESIAN_POINT('Ctrl Pts',(-61.6992235337538,-55.901044674438,-3.70149982734774));
#38529=CARTESIAN_POINT('Ctrl Pts',(-63.427611058795,-57.1821636199741,-3.58458318945645));
#38530=CARTESIAN_POINT('Ctrl Pts',(-64.3502336514788,-59.1257137027476,
-3.46766655156516));
#38531=CARTESIAN_POINT('Ctrl Pts',(-64.2501038781353,-61.27481902782,-3.35074991367387));
#38532=CARTESIAN_POINT('Ctrl Pts',(-63.1509564431981,-63.12416938115,-3.23383327578258));
#38533=CARTESIAN_POINT('Ctrl Pts',(-61.3107783761527,-64.2391240163136,
-3.11691663789129));
#38534=CARTESIAN_POINT('Ctrl Pts',(-59.8790288680541,-64.3177353942359,
-3.03897221263043));
#38535=CARTESIAN_POINT('Ctrl Pts',(-59.1956105045054,-64.1864216867795,
-3.));
#38536=CARTESIAN_POINT('Ctrl Pts',(-55.7373303432786,-59.9999992452069,
-8.67031832941095));
#38537=CARTESIAN_POINT('Ctrl Pts',(-55.7373282291776,-59.6527912211962,
-8.65087842586793));
#38538=CARTESIAN_POINT('Ctrl Pts',(-55.7792938837216,-59.3055837057915,
-8.63143852232492));
#38539=CARTESIAN_POINT('Ctrl Pts',(-55.863233400479,-58.9688389353804,-8.6119986187819));
#38540=CARTESIAN_POINT('Ctrl Pts',(-56.0315114316909,-58.2937487135794,
-8.57302640615147));
#38541=CARTESIAN_POINT('Ctrl Pts',(-56.368483933569,-57.6607086424041,-8.53405419352104));
#38542=CARTESIAN_POINT('Ctrl Pts',(-56.8345413410433,-57.1441286421636,
-8.49508198089061));
#38543=CARTESIAN_POINT('Ctrl Pts',(-57.3005987485177,-56.627548641923,-8.45610976826018));
#38544=CARTESIAN_POINT('Ctrl Pts',(-57.8957410615883,-56.2274287126172,
-8.41713755562975));
#38545=CARTESIAN_POINT('Ctrl Pts',(-58.5500132698641,-55.9908016750967,
-8.37816534299932));
#38546=CARTESIAN_POINT('Ctrl Pts',(-59.2042854781398,-55.7541746375761,
-8.33919313036889));
#38547=CARTESIAN_POINT('Ctrl Pts',(-59.9176875816208,-55.6810404918409,
-8.30022091773846));
#38548=CARTESIAN_POINT('Ctrl Pts',(-60.6063616588423,-55.7799937273555,
-8.26124870510803));
#38549=CARTESIAN_POINT('Ctrl Pts',(-61.2950357360638,-55.8789469628701,
-8.2222764924776));
#38550=CARTESIAN_POINT('Ctrl Pts',(-61.9589817870259,-56.1499875796345,
-8.18330427984717));
#38551=CARTESIAN_POINT('Ctrl Pts',(-62.5201597665573,-56.5612606234307,
-8.14433206721674));
#38552=CARTESIAN_POINT('Ctrl Pts',(-63.0813377460887,-56.9725336672269,
-8.10535985458631));
#38553=CARTESIAN_POINT('Ctrl Pts',(-63.5397476541895,-57.5240391380549,
-8.06638764195588));
#38554=CARTESIAN_POINT('Ctrl Pts',(-63.8414991711302,-58.1509411880593,
-8.02741542932545));
#38555=CARTESIAN_POINT('Ctrl Pts',(-64.1432506880709,-58.7778432380636,
-7.98844321669502));
#38556=CARTESIAN_POINT('Ctrl Pts',(-64.2883438138515,-59.4801418672444,
-7.94947100406459));
#38557=CARTESIAN_POINT('Ctrl Pts',(-64.2597382742518,-60.1753061216449,
-7.91049879143416));
#38558=CARTESIAN_POINT('Ctrl Pts',(-64.231132734652,-60.8704703760455,-7.87152657880373));
#38559=CARTESIAN_POINT('Ctrl Pts',(-64.0288285296718,-61.5585002556659,
-7.83255436617331));
#38560=CARTESIAN_POINT('Ctrl Pts',(-63.6765738366016,-62.1584776996185,
-7.79358215354288));
#38561=CARTESIAN_POINT('Ctrl Pts',(-63.3243191435314,-62.7584551435711,
-7.75460994091245));
#38562=CARTESIAN_POINT('Ctrl Pts',(-62.8221139623713,-63.2703801518559,
-7.71563772828202));
#38563=CARTESIAN_POINT('Ctrl Pts',(-62.2290578496119,-63.6341736522945,
-7.67666551565159));
#38564=CARTESIAN_POINT('Ctrl Pts',(-61.6360017368526,-63.9979671527331,
-7.63769330302116));
#38565=CARTESIAN_POINT('Ctrl Pts',(-60.952094692494,-64.2136291453254,-7.59872109039073));
#38566=CARTESIAN_POINT('Ctrl Pts',(-60.2575790956481,-64.2556048939393,
-7.5597488777603));
#38567=CARTESIAN_POINT('Ctrl Pts',(-59.5630634988021,-64.2975806425533,
-7.52077666512987));
#38568=CARTESIAN_POINT('Ctrl Pts',(-58.8579393494688,-64.1658701471888,
-7.48180445249944));
#38569=CARTESIAN_POINT('Ctrl Pts',(-58.2254073642528,-63.8763972583034,
-7.44283223986901));
#38570=CARTESIAN_POINT('Ctrl Pts',(-57.5928753790369,-63.5869243694181,
-7.40386002723858));
#38571=CARTESIAN_POINT('Ctrl Pts',(-57.0329355579383,-63.1396890870119,
-7.36488781460815));
#38572=CARTESIAN_POINT('Ctrl Pts',(-56.6107196795916,-62.5863063270538,
-7.32591560197772));
#38573=CARTESIAN_POINT('Ctrl Pts',(-56.1885038012448,-62.0329235670957,
-7.28694338934729));
#38574=CARTESIAN_POINT('Ctrl Pts',(-55.9040118656498,-61.3733933295857,
-7.24797117671686));
#38575=CARTESIAN_POINT('Ctrl Pts',(-55.7921583785257,-60.6872970208302,
-7.20899896408643));
#38576=CARTESIAN_POINT('Ctrl Pts',(-55.7551528338003,-60.4603093041987,
-7.1961054191946));
#38577=CARTESIAN_POINT('Ctrl Pts',(-55.7370433843899,-60.2304138053273,
-7.18321187430277));
#38578=CARTESIAN_POINT('Ctrl Pts',(-55.7374565106948,-60.0004827185225,
-7.17031832941094));
#38579=CARTESIAN_POINT('Ctrl Pts',(-58.677115034431,-64.9244061944433,-10.));
#38580=CARTESIAN_POINT('Ctrl Pts',(-58.5386375956257,-64.8748976436074,
-10.));
#38581=CARTESIAN_POINT('Ctrl Pts',(-58.4026668278543,-64.8193821760874,
-10.));
#38582=CARTESIAN_POINT('Ctrl Pts',(-58.2695271742903,-64.7581349586174,
-10.));
#38583=CARTESIAN_POINT('Ctrl Pts',(-58.1353363850557,-64.6964041952369,
-10.));
#38584=CARTESIAN_POINT('Ctrl Pts',(-58.0040209353978,-64.6288503612551,
-10.));
#38585=CARTESIAN_POINT('Ctrl Pts',(-57.8759386493091,-64.5557090804722,
-10.));
#38586=CARTESIAN_POINT('Ctrl Pts',(-57.7488533653713,-64.4831371369214,
-10.));
#38587=CARTESIAN_POINT('Ctrl Pts',(-57.6249505496883,-64.4050638539788,
-10.));
#38588=CARTESIAN_POINT('Ctrl Pts',(-57.5046138228123,-64.321681828014,-10.));
#38589=CARTESIAN_POINT('Ctrl Pts',(-57.3858527597443,-64.239391588771,-10.));
#38590=CARTESIAN_POINT('Ctrl Pts',(-57.2705645355474,-64.1519302045263,
-10.));
#38591=CARTESIAN_POINT('Ctrl Pts',(-57.1591587945395,-64.059453912537,-10.));
#38592=CARTESIAN_POINT('Ctrl Pts',(-57.1274511512158,-64.0331338570733,
-10.));
#38593=CARTESIAN_POINT('Ctrl Pts',(-57.096058289943,-64.0064074129648,-10.));
#38594=CARTESIAN_POINT('Ctrl Pts',(-57.0649903538766,-63.9792778343301,
-10.));
#38595=CARTESIAN_POINT('Ctrl Pts',(-57.049250105535,-63.9655329140301,-10.));
#38596=CARTESIAN_POINT('Ctrl Pts',(-57.0335932654157,-63.9516845134244,
-10.));
#38597=CARTESIAN_POINT('Ctrl Pts',(-57.0180211853758,-63.9377330425149,
-10.));
#38598=CARTESIAN_POINT('Ctrl Pts',(-57.002669719216,-63.9239792258767,-10.));
#38599=CARTESIAN_POINT('Ctrl Pts',(-56.9874066729589,-63.9101306161073,
-10.));
#38600=CARTESIAN_POINT('Ctrl Pts',(-56.9722380221926,-63.8961924090838,
-10.));
#38601=CARTESIAN_POINT('Ctrl Pts',(-56.8611656542019,-63.7941299591337,
-10.));
#38602=CARTESIAN_POINT('Ctrl Pts',(-56.7550656862477,-63.6871906566774,
-10.));
#38603=CARTESIAN_POINT('Ctrl Pts',(-56.6543281719513,-63.5756167101953,
-10.));
#38604=CARTESIAN_POINT('Ctrl Pts',(-56.5578656553598,-63.4687776270703,
-10.));
#38605=CARTESIAN_POINT('Ctrl Pts',(-56.4663199828182,-63.3576879748886,
-10.));
#38606=CARTESIAN_POINT('Ctrl Pts',(-56.3798948426675,-63.2427305259782,
-10.));
#38607=CARTESIAN_POINT('Ctrl Pts',(-56.2936200930167,-63.127973117336,-10.));
#38608=CARTESIAN_POINT('Ctrl Pts',(-56.2124477688271,-63.009360601218,-10.));
#38609=CARTESIAN_POINT('Ctrl Pts',(-56.1366282661676,-62.8872540357093,
-10.));
#38610=CARTESIAN_POINT('Ctrl Pts',(-56.0709511215055,-62.7814816382945,
-10.));
#38611=CARTESIAN_POINT('Ctrl Pts',(-56.0092911147144,-62.6730868734753,
-10.));
#38612=CARTESIAN_POINT('Ctrl Pts',(-55.9518427060363,-62.5622989843102,
-10.));
#38613=CARTESIAN_POINT('Ctrl Pts',(-55.936745519732,-62.5331844197562,-10.));
#38614=CARTESIAN_POINT('Ctrl Pts',(-55.9219393580168,-62.5039045730043,
-10.));
#38615=CARTESIAN_POINT('Ctrl Pts',(-55.9074281095161,-62.4744635977475,
-10.));
#38616=CARTESIAN_POINT('Ctrl Pts',(-55.8951622346766,-62.4495781223432,
-10.));
#38617=CARTESIAN_POINT('Ctrl Pts',(-55.883104401859,-62.4245716453768,-10.));
#38618=CARTESIAN_POINT('Ctrl Pts',(-55.8712719542368,-62.3994789544369,
-10.));
#38619=CARTESIAN_POINT('Ctrl Pts',(-55.8112491416254,-62.2721905070847,
-10.));
#38620=CARTESIAN_POINT('Ctrl Pts',(-55.7569583829528,-62.1425622200571,
-10.));
#38621=CARTESIAN_POINT('Ctrl Pts',(-55.708587651022,-62.0109531311258,-10.));
#38622=CARTESIAN_POINT('Ctrl Pts',(-55.6606046751908,-61.8803990650351,
-10.));
#38623=CARTESIAN_POINT('Ctrl Pts',(-55.6184469915901,-61.7478950950569,
-10.));
#38624=CARTESIAN_POINT('Ctrl Pts',(-55.5823476494758,-61.6137795780905,
-10.));
#38625=CARTESIAN_POINT('Ctrl Pts',(-55.5736126866464,-61.5813276278073,
-10.));
#38626=CARTESIAN_POINT('Ctrl Pts',(-55.5652326741346,-61.5487812944326,
-10.));
#38627=CARTESIAN_POINT('Ctrl Pts',(-55.5572113749489,-61.5161453370011,
-10.));
#38628=CARTESIAN_POINT('Ctrl Pts',(-55.5237968456527,-61.3801929020576,
-10.));
#38629=CARTESIAN_POINT('Ctrl Pts',(-55.4966031557185,-61.2426845833312,
-10.));
#38630=CARTESIAN_POINT('Ctrl Pts',(-55.4756766798638,-61.1040537999156,
-10.));
#38631=CARTESIAN_POINT('Ctrl Pts',(-55.4642433163067,-61.0283116559445,
-10.));
#38632=CARTESIAN_POINT('Ctrl Pts',(-55.4546816621768,-60.9522345623555,
-10.));
#38633=CARTESIAN_POINT('Ctrl Pts',(-55.4470056873523,-60.8758948574348,
-10.));
#38634=CARTESIAN_POINT('Ctrl Pts',(-55.4421350791058,-60.8274553035258,
-10.));
#38635=CARTESIAN_POINT('Ctrl Pts',(-55.438023780299,-60.7789100443811,-10.));
#38636=CARTESIAN_POINT('Ctrl Pts',(-55.434676292913,-60.730277946875,-10.));
#38637=CARTESIAN_POINT('Ctrl Pts',(-55.4333863651453,-60.7115379530405,
-10.));
#38638=CARTESIAN_POINT('Ctrl Pts',(-55.4322097218707,-60.6927825413258,
-10.));
#38639=CARTESIAN_POINT('Ctrl Pts',(-55.4311471090937,-60.6740210732465,
-10.));
#38640=CARTESIAN_POINT('Ctrl Pts',(-55.4233879343862,-60.5370252533725,
-10.));
#38641=CARTESIAN_POINT('Ctrl Pts',(-55.4217193536866,-60.4000017086151,
-10.));
#38642=CARTESIAN_POINT('Ctrl Pts',(-55.4261204723732,-60.2633561204773,
-10.));
#38643=CARTESIAN_POINT('Ctrl Pts',(-55.4305091743339,-60.1270960458709,
-10.));
#38644=CARTESIAN_POINT('Ctrl Pts',(-55.4409335083392,-59.9912110038732,
-10.));
#38645=CARTESIAN_POINT('Ctrl Pts',(-55.4574238144397,-59.8561107187901,
-10.));
#38646=CARTESIAN_POINT('Ctrl Pts',(-55.4736437792729,-59.7232252611376,
-10.));
#38647=CARTESIAN_POINT('Ctrl Pts',(-55.4957326783158,-59.5910983593183,
-10.));
#38648=CARTESIAN_POINT('Ctrl Pts',(-55.523766052396,-59.4601380104691,-10.));
#38649=CARTESIAN_POINT('Ctrl Pts',(-55.536636902664,-59.4000107123332,-10.));
#38650=CARTESIAN_POINT('Ctrl Pts',(-55.5507614616516,-59.3401296350604,
-10.));
#38651=CARTESIAN_POINT('Ctrl Pts',(-55.5661502301349,-59.2805361659048,
-10.));
#38652=CARTESIAN_POINT('Ctrl Pts',(-55.588611195713,-59.1935554006261,-10.));
#38653=CARTESIAN_POINT('Ctrl Pts',(-55.613765125758,-59.1071870025639,-10.));
#38654=CARTESIAN_POINT('Ctrl Pts',(-55.6415742028502,-59.0215529319106,
-10.));
#38655=CARTESIAN_POINT('Ctrl Pts',(-55.6489435652431,-58.998860035712,-10.));
#38656=CARTESIAN_POINT('Ctrl Pts',(-55.6564994205945,-58.9762187463995,
-10.));
#38657=CARTESIAN_POINT('Ctrl Pts',(-55.6642411439561,-58.9536314220447,
-10.));
#38658=CARTESIAN_POINT('Ctrl Pts',(-55.6712493505471,-58.9331842130678,
-10.));
#38659=CARTESIAN_POINT('Ctrl Pts',(-55.6784073237258,-58.9127887539849,
-10.));
#38660=CARTESIAN_POINT('Ctrl Pts',(-55.6857122035675,-58.8924522647103,
-10.));
#38661=CARTESIAN_POINT('Ctrl Pts',(-55.7311295916962,-58.7660120977842,
-10.));
#38662=CARTESIAN_POINT('Ctrl Pts',(-55.7822461341829,-58.6417793104773,
-10.));
#38663=CARTESIAN_POINT('Ctrl Pts',(-55.8388703579017,-58.5201309989478,
-10.));
#38664=CARTESIAN_POINT('Ctrl Pts',(-55.886360628764,-58.4181055602739,-10.));
#38665=CARTESIAN_POINT('Ctrl Pts',(-55.9377259863045,-58.3178982578221,
-10.));
#38666=CARTESIAN_POINT('Ctrl Pts',(-55.9928753041857,-58.2197496529292,
-10.));
#38667=CARTESIAN_POINT('Ctrl Pts',(-56.0250179144583,-58.1625458201878,
-10.));
#38668=CARTESIAN_POINT('Ctrl Pts',(-56.0584462494898,-58.1060416403406,
-10.));
#38669=CARTESIAN_POINT('Ctrl Pts',(-56.0931449566715,-58.0502879461722,
-10.));
#38670=CARTESIAN_POINT('Ctrl Pts',(-56.105064758014,-58.0311352741399,-10.));
#38671=CARTESIAN_POINT('Ctrl Pts',(-56.1171358941824,-58.0120690143348,
-10.));
#38672=CARTESIAN_POINT('Ctrl Pts',(-56.1293531226239,-57.9930985249683,
-10.));
#38673=CARTESIAN_POINT('Ctrl Pts',(-56.2001801780243,-57.8831207253578,
-10.));
#38674=CARTESIAN_POINT('Ctrl Pts',(-56.2758315041106,-57.7764845452586,
-10.));
#38675=CARTESIAN_POINT('Ctrl Pts',(-56.3561469049115,-57.6735585912939,
-10.));
#38676=CARTESIAN_POINT('Ctrl Pts',(-56.4292341049692,-57.5798957356827,
-10.));
#38677=CARTESIAN_POINT('Ctrl Pts',(-56.5061843541636,-57.489305375963,-9.99999999999999));
#38678=CARTESIAN_POINT('Ctrl Pts',(-56.5869001999823,-57.4020947632679,
-9.99999999999999));
#38679=CARTESIAN_POINT('Ctrl Pts',(-56.6479573387169,-57.3361246873252,
-9.99999999999999));
#38680=CARTESIAN_POINT('Ctrl Pts',(-56.711169784743,-57.2720891636053,-10.));
#38681=CARTESIAN_POINT('Ctrl Pts',(-56.7764331763494,-57.2100813324657,
-10.));
#38682=CARTESIAN_POINT('Origin',(-60.,-60.,-6.));
#38683=CARTESIAN_POINT('Origin',(60.,-60.,-3.));
#38684=CARTESIAN_POINT('Ctrl Pts',(60.8043894954945,-64.1864216867795,-3.));
#38685=CARTESIAN_POINT('Ctrl Pts',(60.6804231397008,-64.2229459197079,-3.));
#38686=CARTESIAN_POINT('Ctrl Pts',(60.5549403917413,-64.2536517808237,-3.));
#38687=CARTESIAN_POINT('Ctrl Pts',(60.4283619083555,-64.2786227926487,-3.));
#38688=CARTESIAN_POINT('Ctrl Pts',(60.2999057760435,-64.3039642212482,-3.));
#38689=CARTESIAN_POINT('Ctrl Pts',(60.1703204798203,-64.3233996378784,-3.));
#38690=CARTESIAN_POINT('Ctrl Pts',(60.0400191944093,-64.3369697586679,-3.));
#38691=CARTESIAN_POINT('Ctrl Pts',(59.9818444362653,-64.3430283212709,-3.));
#38692=CARTESIAN_POINT('Ctrl Pts',(59.9235266739776,-64.3479171212406,-3.));
#38693=CARTESIAN_POINT('Ctrl Pts',(59.8651015736501,-64.3516366568403,-3.));
#38694=CARTESIAN_POINT('Ctrl Pts',(59.8415724972579,-64.3531345958559,-3.));
#38695=CARTESIAN_POINT('Ctrl Pts',(59.8180260065396,-64.3544428754694,-3.));
#38696=CARTESIAN_POINT('Ctrl Pts',(59.7944644111293,-64.3555614378551,-3.));
#38697=CARTESIAN_POINT('Ctrl Pts',(59.7710353638239,-64.3566737076565,-3.));
#38698=CARTESIAN_POINT('Ctrl Pts',(59.7476008580321,-64.3575979236003,-3.));
#38699=CARTESIAN_POINT('Ctrl Pts',(59.7241660463876,-64.3583343886706,-3.));
#38700=CARTESIAN_POINT('Ctrl Pts',(59.590446995345,-64.3625366588587,-3.));
#38701=CARTESIAN_POINT('Ctrl Pts',(59.456690295917,-64.3606313991924,-3.));
#38702=CARTESIAN_POINT('Ctrl Pts',(59.3233273468215,-64.352670904561,-3.));
#38703=CARTESIAN_POINT('Ctrl Pts',(59.2153949205287,-64.346228369315,-3.));
#38704=CARTESIAN_POINT('Ctrl Pts',(59.1077197482123,-64.3358188472649,-3.));
#38705=CARTESIAN_POINT('Ctrl Pts',(59.0005240056913,-64.321446190102,-3.));
#38706=CARTESIAN_POINT('Ctrl Pts',(58.9469261344308,-64.3142598615205,-3.));
#38707=CARTESIAN_POINT('Ctrl Pts',(58.8934480606378,-64.3060824109368,-3.));
#38708=CARTESIAN_POINT('Ctrl Pts',(58.8401173770145,-64.2969122626104,-3.));
#38709=CARTESIAN_POINT('Ctrl Pts',(58.8127284789263,-64.2922027737965,-3.));
#38710=CARTESIAN_POINT('Ctrl Pts',(58.785378454751,-64.2872314371142,-3.));
#38711=CARTESIAN_POINT('Ctrl Pts',(58.7580710457004,-64.2819978960498,-3.));
#38712=CARTESIAN_POINT('Ctrl Pts',(58.7384795978033,-64.2782431404488,-3.));
#38713=CARTESIAN_POINT('Ctrl Pts',(58.7189123157833,-64.274353795948,-3.));
#38714=CARTESIAN_POINT('Ctrl Pts',(58.6993815165312,-64.2703322032461,-3.));
#38715=CARTESIAN_POINT('Ctrl Pts',(58.6931277820086,-64.2690444949044,-3.));
#38716=CARTESIAN_POINT('Ctrl Pts',(58.6868774720263,-64.2677431676485,-3.));
#38717=CARTESIAN_POINT('Ctrl Pts',(58.6806306316105,-64.2664282297966,-3.));
#38718=CARTESIAN_POINT('Ctrl Pts',(58.5505753781477,-64.2390520581277,-3.));
#38719=CARTESIAN_POINT('Ctrl Pts',(58.4220248522783,-64.2057808086917,-3.));
#38720=CARTESIAN_POINT('Ctrl Pts',(58.2953075841536,-64.1669086900382,-3.));
#38721=CARTESIAN_POINT('Ctrl Pts',(58.1663244201018,-64.1273414792585,-3.));
#38722=CARTESIAN_POINT('Ctrl Pts',(58.0392399953926,-64.0819712145089,-3.));
#38723=CARTESIAN_POINT('Ctrl Pts',(57.9143959605215,-64.031054382879,-3.));
#38724=CARTESIAN_POINT('Ctrl Pts',(57.7879487637979,-63.9794837120631,-3.));
#38725=CARTESIAN_POINT('Ctrl Pts',(57.6637991096253,-63.9222229571421,-3.));
#38726=CARTESIAN_POINT('Ctrl Pts',(57.5423079332954,-63.8594858324879,-3.));
#38727=CARTESIAN_POINT('Ctrl Pts',(57.4659381105853,-63.8200490336033,-3.));
#38728=CARTESIAN_POINT('Ctrl Pts',(57.390618922556,-63.7784472423405,-3.));
#38729=CARTESIAN_POINT('Ctrl Pts',(57.3164432885815,-63.7347235194873,-3.));
#38730=CARTESIAN_POINT('Ctrl Pts',(57.2554400683084,-63.6987644349004,-3.));
#38731=CARTESIAN_POINT('Ctrl Pts',(57.1952103409945,-63.6613699973526,-3.));
#38732=CARTESIAN_POINT('Ctrl Pts',(57.1358077302662,-63.6225604628414,-3.));
#38733=CARTESIAN_POINT('Ctrl Pts',(57.1208013426853,-63.6127563328618,-3.));
#38734=CARTESIAN_POINT('Ctrl Pts',(57.1058495643152,-63.6028630110964,-3.));
#38735=CARTESIAN_POINT('Ctrl Pts',(57.090962608004,-63.5928872913616,-3.));
#38736=CARTESIAN_POINT('Ctrl Pts',(56.9746403128356,-63.5149399533527,-3.));
#38737=CARTESIAN_POINT('Ctrl Pts',(56.8621130676035,-63.4318607996292,-3.));
#38738=CARTESIAN_POINT('Ctrl Pts',(56.7537373195155,-63.3439210028432,-3.));
#38739=CARTESIAN_POINT('Ctrl Pts',(56.7306086425202,-63.3251536015493,-3.));
#38740=CARTESIAN_POINT('Ctrl Pts',(56.707669073934,-63.3061646372347,-3.));
#38741=CARTESIAN_POINT('Ctrl Pts',(56.6849221396237,-63.2869564466686,-3.));
#38742=CARTESIAN_POINT('Ctrl Pts',(56.579310135636,-63.1977745168753,-3.));
#38743=CARTESIAN_POINT('Ctrl Pts',(56.4778488517895,-63.1038706522824,-3.));
#38744=CARTESIAN_POINT('Ctrl Pts',(56.3807144526095,-63.0056343911719,-3.));
#38745=CARTESIAN_POINT('Ctrl Pts',(56.2824676805631,-62.9062731387887,-3.));
#38746=CARTESIAN_POINT('Ctrl Pts',(56.1886469010809,-62.8024792204072,-3.));
#38747=CARTESIAN_POINT('Ctrl Pts',(56.099462447388,-62.6946104708653,-3.));
#38748=CARTESIAN_POINT('Ctrl Pts',(56.0193271670832,-62.5976867120404,-3.));
#38749=CARTESIAN_POINT('Ctrl Pts',(55.9429351824628,-62.4974722024114,-3.));
#38750=CARTESIAN_POINT('Ctrl Pts',(55.8704637505503,-62.3942009040218,-3.));
#38751=CARTESIAN_POINT('Ctrl Pts',(55.8587176889594,-62.3774628460112,-3.));
#38752=CARTESIAN_POINT('Ctrl Pts',(55.847074674168,-62.3606444428867,-3.));
#38753=CARTESIAN_POINT('Ctrl Pts',(55.8355355278864,-62.343746640643,-3.));
#38754=CARTESIAN_POINT('Ctrl Pts',(55.8253670832934,-62.3288560792734,-3.));
#38755=CARTESIAN_POINT('Ctrl Pts',(55.8152846409939,-62.3139116815137,-3.));
#38756=CARTESIAN_POINT('Ctrl Pts',(55.8052890193779,-62.2989150461428,-3.));
#38757=CARTESIAN_POINT('Ctrl Pts',(55.7260104810182,-62.179971834986,-3.));
#38758=CARTESIAN_POINT('Ctrl Pts',(55.6521810405761,-62.0577313161164,-3.));
#38759=CARTESIAN_POINT('Ctrl Pts',(55.5839783713857,-61.9326058470642,-3.));
#38760=CARTESIAN_POINT('Ctrl Pts',(55.5150429786189,-61.8061361141837,-3.));
#38761=CARTESIAN_POINT('Ctrl Pts',(55.4518553300978,-61.6767185682717,-3.));
#38762=CARTESIAN_POINT('Ctrl Pts',(55.3946314866188,-61.5447373561503,-3.));
#38763=CARTESIAN_POINT('Ctrl Pts',(55.3737738336291,-61.4966312144404,-3.));
#38764=CARTESIAN_POINT('Ctrl Pts',(55.3537088536932,-61.4481841219945,-3.));
#38765=CARTESIAN_POINT('Ctrl Pts',(55.3344483045972,-61.3994135479579,-3.));
#38766=CARTESIAN_POINT('Ctrl Pts',(55.2818816460659,-61.2663069527623,-3.));
#38767=CARTESIAN_POINT('Ctrl Pts',(55.2353035754996,-61.1307925669745,-3.));
#38768=CARTESIAN_POINT('Ctrl Pts',(55.1947264376106,-60.9932848139183,-3.));
#38769=CARTESIAN_POINT('Ctrl Pts',(55.1709932925155,-60.9128579621302,-3.));
#38770=CARTESIAN_POINT('Ctrl Pts',(55.149313907764,-60.8317486932218,-3.));
#38771=CARTESIAN_POINT('Ctrl Pts',(55.1296983571844,-60.7500368036683,-3.));
#38772=CARTESIAN_POINT('Ctrl Pts',(55.1222103856338,-60.7188443932466,-3.));
#38773=CARTESIAN_POINT('Ctrl Pts',(55.1150232214001,-60.6875641489917,-3.));
#38774=CARTESIAN_POINT('Ctrl Pts',(55.1081376485859,-60.656200451121,-3.));
#38775=CARTESIAN_POINT('Ctrl Pts',(55.1026350484047,-60.6311361762608,-3.));
#38776=CARTESIAN_POINT('Ctrl Pts',(55.0973241980932,-60.6060139679337,-3.));
#38777=CARTESIAN_POINT('Ctrl Pts',(55.0922112268448,-60.5808651531185,-3.));
#38778=CARTESIAN_POINT('Ctrl Pts',(55.0630684054444,-60.4375223915442,-3.));
#38779=CARTESIAN_POINT('Ctrl Pts',(55.0403125826176,-60.293155530728,-3.));
#38780=CARTESIAN_POINT('Ctrl Pts',(55.0238938318386,-60.148221636185,-3.));
#38781=CARTESIAN_POINT('Ctrl Pts',(55.007312988479,-60.0018568953307,-3.));
#38782=CARTESIAN_POINT('Ctrl Pts',(54.997194722033,-59.8549131523385,-3.));
#38783=CARTESIAN_POINT('Ctrl Pts',(54.9935343836614,-59.7078349417394,-3.));
#38784=CARTESIAN_POINT('Ctrl Pts',(54.9898705017823,-59.5606143473797,-3.));
#38785=CARTESIAN_POINT('Ctrl Pts',(54.9926768760983,-59.4132582467513,-3.));
#38786=CARTESIAN_POINT('Ctrl Pts',(55.0019985245375,-59.2661976649384,-3.));
#38787=CARTESIAN_POINT('Ctrl Pts',(55.007624207338,-59.1774455315433,-3.));
#38788=CARTESIAN_POINT('Ctrl Pts',(55.0156238601694,-59.0888007981271,-3.));
#38789=CARTESIAN_POINT('Ctrl Pts',(55.0260165547263,-59.0003574320813,-3.));
#38790=CARTESIAN_POINT('Ctrl Pts',(55.0384682951938,-58.8943912811428,-3.));
#38791=CARTESIAN_POINT('Ctrl Pts',(55.0543549121591,-58.7887140498665,-3.));
#38792=CARTESIAN_POINT('Ctrl Pts',(55.0736213077518,-58.683468118019,-3.));
#38793=CARTESIAN_POINT('Ctrl Pts',(56.3967816198431,-56.3921449163111,-3.));
#38794=CARTESIAN_POINT('Ctrl Pts',(56.5101573174658,-56.2959035170913,-3.));
#38795=CARTESIAN_POINT('Ctrl Pts',(56.6276776345426,-56.2048633879271,-2.99999999999999));
#38796=CARTESIAN_POINT('Ctrl Pts',(56.7489442469526,-56.1192063567908,-2.99999999999999));
#38797=CARTESIAN_POINT('Ctrl Pts',(56.870321847077,-56.0334709291534,-3.));
#38798=CARTESIAN_POINT('Ctrl Pts',(56.9954533551651,-55.9531281614561,-3.));
#38799=CARTESIAN_POINT('Ctrl Pts',(57.1239602535777,-55.8784079648384,-3.));
#38800=CARTESIAN_POINT('Ctrl Pts',(57.1803120252051,-55.8456422883824,-3.));
#38801=CARTESIAN_POINT('Ctrl Pts',(57.2373130617797,-55.81395843212,-3.));
#38802=CARTESIAN_POINT('Ctrl Pts',(57.2949321471059,-55.7833788896179,-3.));
#38803=CARTESIAN_POINT('Ctrl Pts',(57.3242693939211,-55.7678090557547,-3.));
#38804=CARTESIAN_POINT('Ctrl Pts',(57.3537668697723,-55.7525255380034,-3.));
#38805=CARTESIAN_POINT('Ctrl Pts',(57.3834204746729,-55.7375315028531,-3.));
#38806=CARTESIAN_POINT('Ctrl Pts',(57.405034144051,-55.7266027770044,-3.));
#38807=CARTESIAN_POINT('Ctrl Pts',(57.42673014855,-55.7158282226589,-3.));
#38808=CARTESIAN_POINT('Ctrl Pts',(57.4484948211874,-55.70521475433,-3.));
#38809=CARTESIAN_POINT('Ctrl Pts',(57.5800081375807,-55.641082734445,-3.));
#38810=CARTESIAN_POINT('Ctrl Pts',(57.7141415282411,-55.5827700253566,-3.));
#38811=CARTESIAN_POINT('Ctrl Pts',(57.8505257224348,-55.5304872340483,-3.));
#38812=CARTESIAN_POINT('Ctrl Pts',(57.9684329260342,-55.4852875849543,-3.));
#38813=CARTESIAN_POINT('Ctrl Pts',(58.0880229434954,-55.4445953492595,-3.));
#38814=CARTESIAN_POINT('Ctrl Pts',(58.2090620298704,-55.4085779565464,-3.));
#38815=CARTESIAN_POINT('Ctrl Pts',(58.2695815730579,-55.3905692601899,-3.));
#38816=CARTESIAN_POINT('Ctrl Pts',(58.330463417215,-55.3737297422003,-3.));
#38817=CARTESIAN_POINT('Ctrl Pts',(58.3916783286023,-55.3580832189175,-3.));
#38818=CARTESIAN_POINT('Ctrl Pts',(58.4205106378725,-55.3507136844679,-3.));
#38819=CARTESIAN_POINT('Ctrl Pts',(58.4494168337012,-55.3436088350695,-3.));
#38820=CARTESIAN_POINT('Ctrl Pts',(58.4783938465815,-55.3367713125311,-3.));
#38821=CARTESIAN_POINT('Ctrl Pts',(58.5046586640999,-55.3305737695858,-3.));
#38822=CARTESIAN_POINT('Ctrl Pts',(58.5309855472865,-55.3245950943735,-3.));
#38823=CARTESIAN_POINT('Ctrl Pts',(58.5573456293696,-55.3188428589396,-3.));
#38824=CARTESIAN_POINT('Ctrl Pts',(58.5636487149566,-55.3174674143511,-3.));
#38825=CARTESIAN_POINT('Ctrl Pts',(58.5699539791781,-55.316104846781,-3.));
#38826=CARTESIAN_POINT('Ctrl Pts',(58.5762613901465,-55.3147551718543,-3.));
#38827=CARTESIAN_POINT('Ctrl Pts',(58.7158133058752,-55.2848935182244,-3.));
#38828=CARTESIAN_POINT('Ctrl Pts',(58.856415423564,-55.2613386928272,-3.));
#38829=CARTESIAN_POINT('Ctrl Pts',(58.9976459175114,-55.2440350244678,-3.));
#38830=CARTESIAN_POINT('Ctrl Pts',(59.1398152514854,-55.2266163287087,-3.));
#38831=CARTESIAN_POINT('Ctrl Pts',(59.282622160811,-55.2155322372454,-3.));
#38832=CARTESIAN_POINT('Ctrl Pts',(59.4256371798734,-55.2107785461175,-3.));
#38833=CARTESIAN_POINT('Ctrl Pts',(59.5672053579002,-55.2060729466897,-3.));
#38834=CARTESIAN_POINT('Ctrl Pts',(59.7089782161267,-55.2075704983195,-3.));
#38835=CARTESIAN_POINT('Ctrl Pts',(59.8505282447802,-55.2153163967581,-3.));
#38836=CARTESIAN_POINT('Ctrl Pts',(59.9398962674022,-55.2202067922845,-3.));
#38837=CARTESIAN_POINT('Ctrl Pts',(60.0291752112974,-55.2275887928648,-3.));
#38838=CARTESIAN_POINT('Ctrl Pts',(60.1182531584719,-55.2374835632598,-3.));
#38839=CARTESIAN_POINT('Ctrl Pts',(60.1850616188527,-55.2449046410561,-3.));
#38840=CARTESIAN_POINT('Ctrl Pts',(60.2517569527163,-55.2537393075563,-3.));
#38841=CARTESIAN_POINT('Ctrl Pts',(60.3182902449357,-55.2639992322029,-3.));
#38842=CARTESIAN_POINT('Ctrl Pts',(60.3359230334911,-55.2667183383203,-3.));
#38843=CARTESIAN_POINT('Ctrl Pts',(60.3535444318793,-55.2695375625048,-3.));
#38844=CARTESIAN_POINT('Ctrl Pts',(60.3711535096332,-55.2724571492995,-3.));
#38845=CARTESIAN_POINT('Ctrl Pts',(60.3893513068264,-55.2754743458341,-3.));
#38846=CARTESIAN_POINT('Ctrl Pts',(60.4075272689998,-55.2785972997792,-3.));
#38847=CARTESIAN_POINT('Ctrl Pts',(60.4256778377815,-55.2818254998691,-3.));
#38848=CARTESIAN_POINT('Ctrl Pts',(60.5629886030953,-55.3062471381247,-3.));
#38849=CARTESIAN_POINT('Ctrl Pts',(60.6988966057003,-55.3366961501879,-3.));
#38850=CARTESIAN_POINT('Ctrl Pts',(60.8330040649825,-55.3731700437297,-3.));
#38851=CARTESIAN_POINT('Ctrl Pts',(60.8581918683798,-55.3800204998087,-3.));
#38852=CARTESIAN_POINT('Ctrl Pts',(60.8833161142963,-55.3870836289852,-3.));
#38853=CARTESIAN_POINT('Ctrl Pts',(60.9083741009857,-55.3943596098957,-3.));
#38854=CARTESIAN_POINT('Ctrl Pts',(61.0423381780513,-55.4332581886002,-3.));
#38855=CARTESIAN_POINT('Ctrl Pts',(61.1744105711619,-55.4782367322963,-3.));
#38856=CARTESIAN_POINT('Ctrl Pts',(61.3042176736396,-55.529086521121,-3.));
#38857=CARTESIAN_POINT('Ctrl Pts',(61.4335910147022,-55.5797663910742,-3.));
#38858=CARTESIAN_POINT('Ctrl Pts',(61.5607148281865,-55.6362788365258,-3.));
#38859=CARTESIAN_POINT('Ctrl Pts',(61.6851875762294,-55.6984578531799,-3.));
#38860=CARTESIAN_POINT('Ctrl Pts',(61.7912746668737,-55.7514525132937,-3.));
#38861=CARTESIAN_POINT('Ctrl Pts',(61.8954357201455,-55.8085642062721,-3.));
#38862=CARTESIAN_POINT('Ctrl Pts',(61.9973985794147,-55.8697095293407,-3.));
#38863=CARTESIAN_POINT('Ctrl Pts',(62.0157427701011,-55.8807102160024,-3.));
#38864=CARTESIAN_POINT('Ctrl Pts',(62.0340157461252,-55.8918415036851,-3.));
#38865=CARTESIAN_POINT('Ctrl Pts',(62.0522158358394,-55.9031029592681,-3.));
#38866=CARTESIAN_POINT('Ctrl Pts',(62.0686109696278,-55.9132475834889,-3.));
#38867=CARTESIAN_POINT('Ctrl Pts',(62.0849391036014,-55.9234929984919,-3.));
#38868=CARTESIAN_POINT('Ctrl Pts',(62.1011958332953,-55.9338364137878,-3.));
#38869=CARTESIAN_POINT('Ctrl Pts',(62.216094328377,-56.0069410832934,-3.));
#38870=CARTESIAN_POINT('Ctrl Pts',(62.327484591668,-56.0849724350915,-3.));
#38871=CARTESIAN_POINT('Ctrl Pts',(62.4350223033254,-56.1677286783298,-3.));
#38872=CARTESIAN_POINT('Ctrl Pts',(62.5416035161753,-56.2497488425985,-3.));
#38873=CARTESIAN_POINT('Ctrl Pts',(62.6444009573507,-56.3364107491799,-3.));
#38874=CARTESIAN_POINT('Ctrl Pts',(62.7430433843076,-56.4275538646491,-3.));
#38875=CARTESIAN_POINT('Ctrl Pts',(62.7758260507536,-56.4578442219066,-3.));
#38876=CARTESIAN_POINT('Ctrl Pts',(62.8081494679239,-56.4886297854746,-3.));
#38877=CARTESIAN_POINT('Ctrl Pts',(62.839998957236,-56.5199054011849,-3.));
#38878=CARTESIAN_POINT('Ctrl Pts',(62.9365721091775,-56.6147384692591,-3.));
#38879=CARTESIAN_POINT('Ctrl Pts',(63.0287915129428,-56.7140757933899,-3.));
#38880=CARTESIAN_POINT('Ctrl Pts',(63.1163847284822,-56.8175811487369,-3.));
#38881=CARTESIAN_POINT('Ctrl Pts',(63.1636034329842,-56.8733775795267,-3.));
#38882=CARTESIAN_POINT('Ctrl Pts',(63.2094769709409,-56.9303855512555,-3.));
#38883=CARTESIAN_POINT('Ctrl Pts',(63.253956548673,-56.988554049022,-3.));
#38884=CARTESIAN_POINT('Ctrl Pts',(63.2715142745527,-57.0115152952992,-3.));
#38885=CARTESIAN_POINT('Ctrl Pts',(63.2888547484807,-57.0346573799277,-3.));
#38886=CARTESIAN_POINT('Ctrl Pts',(63.3059747738216,-57.0579771914561,-3.));
#38887=CARTESIAN_POINT('Ctrl Pts',(63.3199565484319,-57.0770222770943,-3.));
#38888=CARTESIAN_POINT('Ctrl Pts',(63.3337936340754,-57.0961893542109,-3.));
#38889=CARTESIAN_POINT('Ctrl Pts',(63.3474683163229,-57.1154538857274,-3.));
#38890=CARTESIAN_POINT('Ctrl Pts',(63.42423513697,-57.2236009570091,-3.));
#38891=CARTESIAN_POINT('Ctrl Pts',(63.4959842891767,-57.3349453279282,-3.));
#38892=CARTESIAN_POINT('Ctrl Pts',(63.5625181311883,-57.4491372731137,-3.));
#38893=CARTESIAN_POINT('Ctrl Pts',(63.6288088907953,-57.5629120162892,-3.));
#38894=CARTESIAN_POINT('Ctrl Pts',(63.6899226778965,-57.6795143212801,-3.00000000000001));
#38895=CARTESIAN_POINT('Ctrl Pts',(63.7456163898184,-57.7986178371963,-3.));
#38896=CARTESIAN_POINT('Ctrl Pts',(63.8003210973205,-57.9156063225357,-3.));
#38897=CARTESIAN_POINT('Ctrl Pts',(63.8497966746643,-58.0350086748614,-3.));
#38898=CARTESIAN_POINT('Ctrl Pts',(63.8937635413419,-58.1565237236026,-3.));
#38899=CARTESIAN_POINT('Ctrl Pts',(63.9160764751396,-58.2181919170143,-3.));
#38900=CARTESIAN_POINT('Ctrl Pts',(63.9369698330113,-58.2804043019419,-3.));
#38901=CARTESIAN_POINT('Ctrl Pts',(63.9564018939967,-58.3431214778336,-3.));
#38902=CARTESIAN_POINT('Ctrl Pts',(63.982990724922,-58.4289372020198,-3.));
#38903=CARTESIAN_POINT('Ctrl Pts',(64.0068440160574,-58.5156982224054,-3.));
#38904=CARTESIAN_POINT('Ctrl Pts',(64.0279239112946,-58.6032685651143,-3.));
#38905=CARTESIAN_POINT('Origin',(60.,-60.,-13.3123464956316));
#38906=CARTESIAN_POINT('Ctrl Pts',(65.0992547697949,-59.9999087515425,-9.56234649563159));
#38907=CARTESIAN_POINT('Ctrl Pts',(65.0993446299649,-59.8930270626359,-9.55734157105847));
#38908=CARTESIAN_POINT('Ctrl Pts',(65.0703981688746,-58.9539304661534,-9.51336443385491));
#38909=CARTESIAN_POINT('Ctrl Pts',(64.5173398889406,-57.2140033571025,-9.43041508402093));
#38910=CARTESIAN_POINT('Ctrl Pts',(62.675830507843,-55.416544576301,-9.31349844612964));
#38911=CARTESIAN_POINT('Ctrl Pts',(60.2052631333967,-54.6966046481226,-9.19658180823834));
#38912=CARTESIAN_POINT('Ctrl Pts',(57.6864406075043,-55.2234346241344,-9.07966517034706));
#38913=CARTESIAN_POINT('Ctrl Pts',(55.7115103085732,-56.8731820153015,-8.96274853245577));
#38914=CARTESIAN_POINT('Ctrl Pts',(54.7447564371768,-59.2580098897298,-8.84583189456448));
#38915=CARTESIAN_POINT('Ctrl Pts',(55.0134521540628,-61.8172711292634,-8.72891525667319));
#38916=CARTESIAN_POINT('Ctrl Pts',(56.4544300397442,-63.9493126239243,-8.6119986187819));
#38917=CARTESIAN_POINT('Ctrl Pts',(58.7289322008878,-65.1529132302293,-8.4950819808906));
#38918=CARTESIAN_POINT('Ctrl Pts',(61.3022482555275,-65.145123605987,-8.37816534299932));
#38919=CARTESIAN_POINT('Ctrl Pts',(63.5694203198369,-63.9277667461252,-8.26124870510802));
#38920=CARTESIAN_POINT('Ctrl Pts',(64.8552427738849,-62.0002410971054,-8.15597575598546));
#38921=CARTESIAN_POINT('Ctrl Pts',(65.09834724995,-60.583627205272,-8.08967501949331));
#38922=CARTESIAN_POINT('Ctrl Pts',(65.0988481317111,-59.9998830050765,-8.06234649563159));
#38923=CARTESIAN_POINT('Ctrl Pts',(65.0987893869763,-59.9998803238954,-9.68765350436841));
#38924=CARTESIAN_POINT('Ctrl Pts',(65.0989958636635,-59.7264419125984,-9.67485236502099));
#38925=CARTESIAN_POINT('Ctrl Pts',(65.0114730856874,-58.6206707254151,-9.62307901304313));
#38926=CARTESIAN_POINT('Ctrl Pts',(64.2231822374133,-56.7854927040709,-9.53233344843484));
#38927=CARTESIAN_POINT('Ctrl Pts',(62.2146698199313,-55.1767965300925,-9.41541681054356));
#38928=CARTESIAN_POINT('Ctrl Pts',(59.6855379300098,-54.7019554558395,-9.29850017265226));
#38929=CARTESIAN_POINT('Ctrl Pts',(57.2303209690299,-55.4726378662523,-9.18158353476098));
#38930=CARTESIAN_POINT('Ctrl Pts',(55.4262302424911,-57.3076473811431,-9.06466689686968));
#38931=CARTESIAN_POINT('Ctrl Pts',(54.6973796557714,-59.775601760132,-8.9477502589784));
#38932=CARTESIAN_POINT('Ctrl Pts',(55.2151175549311,-62.2963084797734,-8.8308336210871));
#38933=CARTESIAN_POINT('Ctrl Pts',(56.8577277980376,-64.2771790632985,-8.71391698319582));
#38934=CARTESIAN_POINT('Ctrl Pts',(59.2390517062358,-65.2525319290857,-8.59700034530453));
#38935=CARTESIAN_POINT('Ctrl Pts',(61.7992659861865,-64.9930728587382,-8.48008370741324));
#38936=CARTESIAN_POINT('Ctrl Pts',(63.9364928774652,-63.5597974904555,-8.36316706952195));
#38937=CARTESIAN_POINT('Ctrl Pts',(64.9468057743096,-61.667113625277,-8.26569033517367));
#38938=CARTESIAN_POINT('Ctrl Pts',(65.0986024103333,-60.4172707879301,-8.20718581345583));
#38939=CARTESIAN_POINT('Ctrl Pts',(65.0986049509612,-59.9999990973777,-8.18765350436841));
#38940=CARTESIAN_POINT('Ctrl Pts',(56.7766472160421,-57.2101674189746,-10.));
#38941=CARTESIAN_POINT('Ctrl Pts',(56.3212170277455,-57.7363682294923,-9.96102778736957));
#38942=CARTESIAN_POINT('Ctrl Pts',(55.6734222457032,-59.0156058825944,-9.88308336210871));
#38943=CARTESIAN_POINT('Ctrl Pts',(55.718911726351,-61.1667236883496,-9.76616672421742));
#38944=CARTESIAN_POINT('Ctrl Pts',(56.7709224459031,-63.0432885509004,-9.64925008632614));
#38945=CARTESIAN_POINT('Ctrl Pts',(58.5820372950378,-64.2045560436868,-9.53233344843484));
#38946=CARTESIAN_POINT('Ctrl Pts',(60.7265123811851,-64.3773165159145,-9.41541681054356));
#38947=CARTESIAN_POINT('Ctrl Pts',(62.7001877066388,-63.5210484489301,-9.29850017265226));
#38948=CARTESIAN_POINT('Ctrl Pts',(64.0390812798309,-61.8370072052861,-9.18158353476097));
#38949=CARTESIAN_POINT('Ctrl Pts',(64.4284304814287,-59.7211123027545,-9.06466689686969));
#38950=CARTESIAN_POINT('Ctrl Pts',(63.7767052258391,-57.6707778606252,-8.9477502589784));
#38951=CARTESIAN_POINT('Ctrl Pts',(62.2371181515856,-56.1680191270389,-8.83083362108711));
#38952=CARTESIAN_POINT('Ctrl Pts',(60.1716094798333,-55.5661160256809,-8.71391698319581));
#38953=CARTESIAN_POINT('Ctrl Pts',(58.0657572680508,-56.0065702692067,-8.59700034530453));
#38954=CARTESIAN_POINT('Ctrl Pts',(56.4146241312899,-57.385835444446,-8.48008370741324));
#38955=CARTESIAN_POINT('Ctrl Pts',(55.6063731499676,-59.3796619258518,-8.36316706952194));
#38956=CARTESIAN_POINT('Ctrl Pts',(55.8310152054854,-61.519322773887,-8.24625043163066));
#38957=CARTESIAN_POINT('Ctrl Pts',(57.0357394115374,-63.3018081419473,-8.12933379373937));
#38958=CARTESIAN_POINT('Ctrl Pts',(58.9373284903676,-64.3080739557693,-8.01241715584808));
#38959=CARTESIAN_POINT('Ctrl Pts',(61.0887398143388,-64.301561469371,-7.89550051795679));
#38960=CARTESIAN_POINT('Ctrl Pts',(62.9842005929525,-63.2837947908868,-7.7785838800655));
#38961=CARTESIAN_POINT('Ctrl Pts',(64.1781085723986,-61.4940544999883,-7.66166724217421));
#38962=CARTESIAN_POINT('Ctrl Pts',(64.3897900935251,-59.3530565503543,-7.54475060428292));
#38963=CARTESIAN_POINT('Ctrl Pts',(63.5694792575328,-57.3641953191966,-7.42783396639163));
#38964=CARTESIAN_POINT('Ctrl Pts',(61.9100261963604,-55.9948800845054,-7.31091732850034));
#38965=CARTESIAN_POINT('Ctrl Pts',(59.80154101086,-55.5673455413723,-7.19400069060905));
#38966=CARTESIAN_POINT('Ctrl Pts',(57.7397244908903,-56.1814012155801,-7.07708405271776));
#38967=CARTESIAN_POINT('Ctrl Pts',(56.2092451179269,-57.6941993755668,-6.96016741482647));
#38968=CARTESIAN_POINT('Ctrl Pts',(55.5699911243389,-59.7468398452376,-6.84325077693518));
#38969=CARTESIAN_POINT('Ctrl Pts',(55.9720482818244,-61.8638130771427,-6.7263341390439));
#38970=CARTESIAN_POINT('Ctrl Pts',(57.3213007331271,-63.5322807113462,-6.60941750115261));
#38971=CARTESIAN_POINT('Ctrl Pts',(59.9592778669654,-64.6795929264981,-6.45352865063088));
#38972=CARTESIAN_POINT('Ctrl Pts',(63.6618729284737,-63.4214740641546,-6.25866758747874));
#38973=CARTESIAN_POINT('Ctrl Pts',(64.8778950002124,-58.8502441638021,-6.02483431169615));
#38974=CARTESIAN_POINT('Ctrl Pts',(62.2898180510687,-55.9187034483083,-5.82997324854401));
#38975=CARTESIAN_POINT('Ctrl Pts',(59.4304512147069,-55.6036320709857,-5.67408439802228));
#38976=CARTESIAN_POINT('Ctrl Pts',(57.4305231142087,-56.3811627884273,-5.557167760131));
#38977=CARTESIAN_POINT('Ctrl Pts',(56.0297440088743,-58.0185520275981,-5.4402511222397));
#38978=CARTESIAN_POINT('Ctrl Pts',(55.5646048065108,-60.1175098853142,-5.32333448434842));
#38979=CARTESIAN_POINT('Ctrl Pts',(56.1411247560802,-62.1908043968745,-5.20641784645713));
#38980=CARTESIAN_POINT('Ctrl Pts',(57.6253115974258,-63.7481550809134,-5.08950120856584));
#38981=CARTESIAN_POINT('Ctrl Pts',(59.6675354162127,-64.4247771592285,-4.97258457067455));
#38982=CARTESIAN_POINT('Ctrl Pts',(61.7880226520338,-64.0609879932485,-4.85566793278326));
#38983=CARTESIAN_POINT('Ctrl Pts',(63.4881170828804,-62.7425958702478,-4.73875129489197));
#38984=CARTESIAN_POINT('Ctrl Pts',(64.368216261483,-60.7794079721259,-4.62183465700068));
#38985=CARTESIAN_POINT('Ctrl Pts',(64.2213857622817,-58.6330092727112,-4.50491801910939));
#38986=CARTESIAN_POINT('Ctrl Pts',(63.0821590289871,-56.8079659797403,-4.3880013812181));
#38987=CARTESIAN_POINT('Ctrl Pts',(61.2183485971665,-55.7333387017859,-4.27108474332681));
#38988=CARTESIAN_POINT('Ctrl Pts',(59.0681189462196,-55.6617543251732,-4.15416810543552));
#38989=CARTESIAN_POINT('Ctrl Pts',(57.13696370596,-56.6100443722557,-4.03725146754423));
#38990=CARTESIAN_POINT('Ctrl Pts',(55.8788768822095,-58.3552750250779,-3.92033482965294));
#38991=CARTESIAN_POINT('Ctrl Pts',(55.5896202375636,-60.4871625334629,-3.80341819176165));
#38992=CARTESIAN_POINT('Ctrl Pts',(56.3371953794376,-62.5045233639532,-3.68650155387036));
#38993=CARTESIAN_POINT('Ctrl Pts',(57.9458546871605,-63.9330986778457,-3.56958491597908));
#38994=CARTESIAN_POINT('Ctrl Pts',(60.0374221724598,-64.4370456883152,-3.45266827808778));
#38995=CARTESIAN_POINT('Ctrl Pts',(62.1201892117601,-63.8978931193146,-3.3357516401965));
#38996=CARTESIAN_POINT('Ctrl Pts',(63.7045295455676,-62.4423874949933,-3.2188350023052));
#38997=CARTESIAN_POINT('Ctrl Pts',(64.4179625394253,-60.412707063655,-3.10191836441392));
#38998=CARTESIAN_POINT('Ctrl Pts',(64.0928111495996,-58.285996892823,-2.98500172652263));
#38999=CARTESIAN_POINT('Ctrl Pts',(62.8054238049257,-56.5622471978326,-2.86808508863134));
#39000=CARTESIAN_POINT('Ctrl Pts',(60.8586569290977,-55.6466485037356,-2.75116845074005));
#39001=CARTESIAN_POINT('Ctrl Pts',(58.7097669209642,-55.7545782960891,-2.63425181284876));
#39002=CARTESIAN_POINT('Ctrl Pts',(57.4799483719373,-56.4918932825098,-2.5563073875879));
#39003=CARTESIAN_POINT('Ctrl Pts',(56.9875426643246,-56.9836661655686,-2.51733517495747));
#39004=CARTESIAN_POINT('Ctrl Pts',(56.5659409116095,-57.0277997563163,-10.1608882750142));
#39005=CARTESIAN_POINT('Ctrl Pts',(56.0807398547996,-57.5883976172362,-10.1219160623837));
#39006=CARTESIAN_POINT('Ctrl Pts',(55.3905995854019,-58.9512573422744,-10.0439716371229));
#39007=CARTESIAN_POINT('Ctrl Pts',(55.4390626531811,-61.2429908713554,-9.9270549992316));
#39008=CARTESIAN_POINT('Ctrl Pts',(56.5598419208249,-63.242224294786,-9.81013836134031));
#39009=CARTESIAN_POINT('Ctrl Pts',(58.4893469501049,-64.4794023062971,-9.69322172344902));
#39010=CARTESIAN_POINT('Ctrl Pts',(60.7740035337905,-64.663455901895,-9.57630508555773));
#39011=CARTESIAN_POINT('Ctrl Pts',(62.8766954025297,-63.7512147248943,-9.45938844766644));
#39012=CARTESIAN_POINT('Ctrl Pts',(64.3031106761823,-61.9570899344768,-9.34247180977515));
#39013=CARTESIAN_POINT('Ctrl Pts',(64.7179111196705,-59.7028817831754,-9.22555517188386));
#39014=CARTESIAN_POINT('Ctrl Pts',(64.0235834468729,-57.5185196927843,-9.10863853399257));
#39015=CARTESIAN_POINT('Ctrl Pts',(62.3833556036714,-55.9175276101262,-8.99172189610129));
#39016=CARTESIAN_POINT('Ctrl Pts',(60.1828273643545,-55.2762788998282,-8.87480525820999));
#39017=CARTESIAN_POINT('Ctrl Pts',(57.9393183812019,-55.7455250541826,-8.7578886203187));
#39018=CARTESIAN_POINT('Ctrl Pts',(56.180252857051,-57.2149509680645,-8.64097198242742));
#39019=CARTESIAN_POINT('Ctrl Pts',(55.3191675790373,-59.3391112471445,-8.52405534453612));
#39020=CARTESIAN_POINT('Ctrl Pts',(55.5584941883445,-61.6186388923458,-8.40713870664483));
#39021=CARTESIAN_POINT('Ctrl Pts',(56.8419696209397,-63.5176429692729,-8.29022206875355));
#39022=CARTESIAN_POINT('Ctrl Pts',(58.867863060541,-64.589687047256,-8.17330543086226));
#39023=CARTESIAN_POINT('Ctrl Pts',(61.159909294735,-64.5827488482429,-8.05638879297097));
#39024=CARTESIAN_POINT('Ctrl Pts',(63.1792738352472,-63.4984521092996,-7.93947215507967));
#39025=CARTESIAN_POINT('Ctrl Pts',(64.4512259988217,-61.5917188648323,-7.82255551718839));
#39026=CARTESIAN_POINT('Ctrl Pts',(64.6767448607616,-59.3107667134707,-7.70563887929709));
#39027=CARTESIAN_POINT('Ctrl Pts',(63.8028113913429,-57.1918962564746,-7.58872224140581));
#39028=CARTESIAN_POINT('Ctrl Pts',(62.0348820803355,-55.7330706975828,-7.47180560351451));
#39029=CARTESIAN_POINT('Ctrl Pts',(59.7885680094587,-55.2775887873327,-7.35488896562323));
#39030=CARTESIAN_POINT('Ctrl Pts',(57.5919732729987,-55.9317844680803,-7.23797232773194));
#39031=CARTESIAN_POINT('Ctrl Pts',(55.9614484894639,-57.5434722411524,-7.12105568984065));
#39032=CARTESIAN_POINT('Ctrl Pts',(55.2804073085556,-59.7302911010526,-7.00413905194936));
#39033=CARTESIAN_POINT('Ctrl Pts',(55.7087464101851,-61.9856480706912,-6.88722241405807));
#39034=CARTESIAN_POINT('Ctrl Pts',(57.1461977080973,-63.7631812254352,-6.77030577616678));
#39035=CARTESIAN_POINT('Ctrl Pts',(59.9566159150367,-64.9854917212868,-6.61441692564506));
#39036=CARTESIAN_POINT('Ctrl Pts',(63.901244714243,-63.6451312944018,-6.41955586249291));
#39037=CARTESIAN_POINT('Ctrl Pts',(65.1967565390488,-58.7750861468296,-6.18572258671033));
#39038=CARTESIAN_POINT('Ctrl Pts',(62.4395004258199,-55.6519144955196,-5.99086152355818));
#39039=CARTESIAN_POINT('Ctrl Pts',(59.3932205645775,-55.316247319351,-5.83497267303646));
#39040=CARTESIAN_POINT('Ctrl Pts',(57.2625598116423,-56.1446041905014,-5.71805603514517));
#39041=CARTESIAN_POINT('Ctrl Pts',(55.770213630535,-57.8890273966708,-5.60113939725388));
#39042=CARTESIAN_POINT('Ctrl Pts',(55.2746688942615,-60.1251913509584,-5.48422275936259));
#39043=CARTESIAN_POINT('Ctrl Pts',(55.8888751897406,-62.3340143801247,-5.36730612147131));
#39044=CARTESIAN_POINT('Ctrl Pts',(57.4700813601475,-63.9931670167679,-5.25038948358002));
#39045=CARTESIAN_POINT('Ctrl Pts',(59.6458026464851,-64.7140189846344,-5.13347284568873));
#39046=CARTESIAN_POINT('Ctrl Pts',(61.9049033258238,-64.3264494024561,-5.01655620779743));
#39047=CARTESIAN_POINT('Ctrl Pts',(63.7161306790402,-62.9218757316543,-4.89963956990615));
#39048=CARTESIAN_POINT('Ctrl Pts',(64.6537607758782,-60.8303568394882,-4.78272293201486));
#39049=CARTESIAN_POINT('Ctrl Pts',(64.4973321613174,-58.5436508984823,-4.66580629412357));
#39050=CARTESIAN_POINT('Ctrl Pts',(63.2836356845687,-56.5993069414311,-4.54888965623228));
#39051=CARTESIAN_POINT('Ctrl Pts',(61.2979904321209,-55.4544327009018,-4.43197301834099));
#39052=CARTESIAN_POINT('Ctrl Pts',(59.0072031153524,-55.3781689483529,-4.3150563804497));
#39053=CARTESIAN_POINT('Ctrl Pts',(56.9498108134885,-56.3884474604725,-4.19813974255841));
#39054=CARTESIAN_POINT('Ctrl Pts',(55.6094845195171,-58.2477615307441,-4.08122310466712));
#39055=CARTESIAN_POINT('Ctrl Pts',(55.3013195509269,-60.5190077033726,-3.96430646677583));
#39056=CARTESIAN_POINT('Ctrl Pts',(56.0977626901898,-62.6682407407822,-3.84738982888454));
#39057=CARTESIAN_POINT('Ctrl Pts',(57.8115779273252,-64.1902001318044,-3.73047319099325));
#39058=CARTESIAN_POINT('Ctrl Pts',(60.0398684103342,-64.7270894912265,-3.61355655310196));
#39059=CARTESIAN_POINT('Ctrl Pts',(62.2587831738394,-64.1526932325171,-3.49663991521067));
#39060=CARTESIAN_POINT('Ctrl Pts',(63.9466897379277,-62.6020431323234,-3.37972327731938));
#39061=CARTESIAN_POINT('Ctrl Pts',(64.7067589021557,-60.4396851780671,-3.26280663942809));
#39062=CARTESIAN_POINT('Ctrl Pts',(64.3603527964105,-58.1739547786936,-3.1458900015368));
#39063=CARTESIAN_POINT('Ctrl Pts',(62.9888106452508,-56.3375258480311,-3.02897336364551));
#39064=CARTESIAN_POINT('Ctrl Pts',(60.9147861958681,-55.3620756793649,-2.91205672575422));
#39065=CARTESIAN_POINT('Ctrl Pts',(58.6254260925902,-55.4770606993678,-2.79514008786293));
#39066=CARTESIAN_POINT('Ctrl Pts',(57.3152159330397,-56.2625729903977,-2.71719566260207));
#39067=CARTESIAN_POINT('Ctrl Pts',(56.7906223161641,-56.7864924158161,-2.67822344997164));
#39068=CARTESIAN_POINT('Ctrl Pts',(56.3552346071769,-56.845432093658,-10.3217765500284));
#39069=CARTESIAN_POINT('Ctrl Pts',(55.8402626818537,-57.44042700498,-10.2828043373979));
#39070=CARTESIAN_POINT('Ctrl Pts',(55.1077769251007,-58.8869088019546,-10.2048599121371));
#39071=CARTESIAN_POINT('Ctrl Pts',(55.1592135800111,-61.3192580543611,-10.0879432742458));
#39072=CARTESIAN_POINT('Ctrl Pts',(56.3487613957467,-63.4411600386716,-9.97102663635449));
#39073=CARTESIAN_POINT('Ctrl Pts',(58.3966566051718,-64.7542485689073,-9.85410999846319));
#39074=CARTESIAN_POINT('Ctrl Pts',(60.8214946863959,-64.9495952878756,-9.73719336057191));
#39075=CARTESIAN_POINT('Ctrl Pts',(63.0532030984208,-63.9813810008584,-9.62027672268061));
#39076=CARTESIAN_POINT('Ctrl Pts',(64.5671400725337,-62.0771726636675,-9.50336008478933));
#39077=CARTESIAN_POINT('Ctrl Pts',(65.0073917579124,-59.6846512635963,-9.38644344689803));
#39078=CARTESIAN_POINT('Ctrl Pts',(64.2704616679068,-57.3662615249434,-9.26952680900675));
#39079=CARTESIAN_POINT('Ctrl Pts',(62.5295930557572,-55.6670360932137,-9.15261017111546));
#39080=CARTESIAN_POINT('Ctrl Pts',(60.1940452488756,-54.9864417739754,-9.03569353322417));
#39081=CARTESIAN_POINT('Ctrl Pts',(57.8128794943531,-55.4844798391586,-8.91877689533288));
#39082=CARTESIAN_POINT('Ctrl Pts',(55.9458815828121,-57.044066491683,-8.80186025744159));
#39083=CARTESIAN_POINT('Ctrl Pts',(55.0319620081071,-59.2985605684372,-8.6849436195503));
#39084=CARTESIAN_POINT('Ctrl Pts',(55.2859731712037,-61.7179550108046,-8.56802698165902));
#39085=CARTESIAN_POINT('Ctrl Pts',(56.6481998303419,-63.7334777965986,-8.45111034376772));
#39086=CARTESIAN_POINT('Ctrl Pts',(58.7983976307144,-64.8713001387427,-8.33419370587643));
#39087=CARTESIAN_POINT('Ctrl Pts',(61.2310787751313,-64.863936227115,-8.21727706798515));
#39088=CARTESIAN_POINT('Ctrl Pts',(63.374347077542,-63.7131094277124,-8.10036043009385));
#39089=CARTESIAN_POINT('Ctrl Pts',(64.7243434252448,-61.6893832296763,-7.98344379220257));
#39090=CARTESIAN_POINT('Ctrl Pts',(64.9636996279981,-59.2684768765872,-7.86652715431127));
#39091=CARTESIAN_POINT('Ctrl Pts',(64.0361435251531,-57.0195971937526,-7.74961051641999));
#39092=CARTESIAN_POINT('Ctrl Pts',(62.1597379643106,-55.4712613106602,-7.6326938785287));
#39093=CARTESIAN_POINT('Ctrl Pts',(59.7755950080574,-54.9878320332931,-7.5157772406374));
#39094=CARTESIAN_POINT('Ctrl Pts',(57.4442220551071,-55.6821677205805,-7.39886060274612));
#39095=CARTESIAN_POINT('Ctrl Pts',(55.7136518610009,-57.3927451067379,-7.28194396485483));
#39096=CARTESIAN_POINT('Ctrl Pts',(54.9908234927723,-59.7137423568676,-7.16502732696353));
#39097=CARTESIAN_POINT('Ctrl Pts',(55.4454445385458,-62.1074830642397,-7.04811068907225));
#39098=CARTESIAN_POINT('Ctrl Pts',(56.9710946830675,-63.9940817395243,-6.93119405118096));
#39099=CARTESIAN_POINT('Ctrl Pts',(59.9539539631079,-65.2913905160755,-6.77530520065924));
#39100=CARTESIAN_POINT('Ctrl Pts',(64.1406165000123,-63.8687885246491,-6.58044413750709));
#39101=CARTESIAN_POINT('Ctrl Pts',(65.5156180778851,-58.6999281298572,-6.34661086172451));
#39102=CARTESIAN_POINT('Ctrl Pts',(62.5891828005711,-55.3851255427309,-6.15174979857236));
#39103=CARTESIAN_POINT('Ctrl Pts',(59.355989914448,-55.0288625677164,-5.99586094805064));
#39104=CARTESIAN_POINT('Ctrl Pts',(57.0945965090759,-55.9080455925754,-5.87894431015935));
#39105=CARTESIAN_POINT('Ctrl Pts',(55.5106832521958,-57.7595027657436,-5.76202767226806));
#39106=CARTESIAN_POINT('Ctrl Pts',(54.9847329820121,-60.1328728166025,-5.64511103437677));
#39107=CARTESIAN_POINT('Ctrl Pts',(55.6366256234011,-62.4772243633749,-5.52819439648548));
#39108=CARTESIAN_POINT('Ctrl Pts',(57.3148511228692,-64.2381789526224,-5.41127775859419));
#39109=CARTESIAN_POINT('Ctrl Pts',(59.6240698767575,-65.0032608100402,-5.2943611207029));
#39110=CARTESIAN_POINT('Ctrl Pts',(62.0217839996138,-64.5919108116637,-5.17744448281161));
#39111=CARTESIAN_POINT('Ctrl Pts',(63.9441442752001,-63.1011555930607,-5.06052784492032));
#39112=CARTESIAN_POINT('Ctrl Pts',(64.9393052902734,-60.8813057068506,-4.94361120702903));
#39113=CARTESIAN_POINT('Ctrl Pts',(64.773278560353,-58.4542925242534,-4.82669456913774));
#39114=CARTESIAN_POINT('Ctrl Pts',(63.4851123401503,-56.3906479031218,-4.70977793124645));
#39115=CARTESIAN_POINT('Ctrl Pts',(61.3776322670752,-55.1755267000177,-4.59286129335516));
#39116=CARTESIAN_POINT('Ctrl Pts',(58.9462872844852,-55.0945835715325,-4.47594465546388));
#39117=CARTESIAN_POINT('Ctrl Pts',(56.7626579210171,-56.1668505486894,-4.35902801757258));
#39118=CARTESIAN_POINT('Ctrl Pts',(55.3400921568247,-58.1402480364103,-4.2421113796813));
#39119=CARTESIAN_POINT('Ctrl Pts',(55.0130188642902,-60.5508528732823,-4.12519474179001));
#39120=CARTESIAN_POINT('Ctrl Pts',(55.858330000942,-62.8319581176111,-4.00827810389872));
#39121=CARTESIAN_POINT('Ctrl Pts',(57.6773011674899,-64.4473015857632,-3.89136146600743));
#39122=CARTESIAN_POINT('Ctrl Pts',(60.0423146482087,-65.0171332941376,-3.77444482811614));
#39123=CARTESIAN_POINT('Ctrl Pts',(62.3973771359187,-64.4074933457197,-3.65752819022485));
#39124=CARTESIAN_POINT('Ctrl Pts',(64.1888499302879,-62.7616987696534,-3.54061155233356));
#39125=CARTESIAN_POINT('Ctrl Pts',(64.9955552648861,-60.4666632924791,-3.42369491444227));
#39126=CARTESIAN_POINT('Ctrl Pts',(64.6278944432215,-58.0619126645643,-3.30677827655098));
#39127=CARTESIAN_POINT('Ctrl Pts',(63.1721974855759,-56.1128044982296,-3.18986163865969));
#39128=CARTESIAN_POINT('Ctrl Pts',(60.9709154626384,-55.0775028549942,-3.0729450007684));
#39129=CARTESIAN_POINT('Ctrl Pts',(58.5410852642163,-55.1995431026464,-2.95602836287711));
#39130=CARTESIAN_POINT('Ctrl Pts',(57.1504834941422,-56.0332526982856,-2.87808393761625));
#39131=CARTESIAN_POINT('Ctrl Pts',(56.5937019680036,-56.5893186660636,-2.83911172498582));
#39132=CARTESIAN_POINT('Ctrl Pts',(56.1445283027442,-56.6630644309996,-10.4826648250425));
#39133=CARTESIAN_POINT('Ctrl Pts',(55.5997855089079,-57.2924563927238,-10.4436926124121));
#39134=CARTESIAN_POINT('Ctrl Pts',(54.8249542647996,-58.8225602616346,-10.3657481871512));
#39135=CARTESIAN_POINT('Ctrl Pts',(54.8793645068411,-61.3955252373669,-10.24883154926));
#39136=CARTESIAN_POINT('Ctrl Pts',(56.1376808706685,-63.6400957825572,-10.1319149113687));
#39137=CARTESIAN_POINT('Ctrl Pts',(58.3039662602388,-65.0290948315175,-10.0149982734774));
#39138=CARTESIAN_POINT('Ctrl Pts',(60.8689858390013,-65.2357346738561,-9.89808163558608));
#39139=CARTESIAN_POINT('Ctrl Pts',(63.2297107943118,-64.2115472768226,-9.78116499769479));
#39140=CARTESIAN_POINT('Ctrl Pts',(64.8311694688852,-62.1972553928581,-9.6642483598035));
#39141=CARTESIAN_POINT('Ctrl Pts',(65.2968723961542,-59.6664207440172,-9.54733172191222));
#39142=CARTESIAN_POINT('Ctrl Pts',(64.5173398889406,-57.2140033571025,-9.43041508402093));
#39143=CARTESIAN_POINT('Ctrl Pts',(62.675830507843,-55.416544576301,-9.31349844612964));
#39144=CARTESIAN_POINT('Ctrl Pts',(60.2052631333967,-54.6966046481226,-9.19658180823834));
#39145=CARTESIAN_POINT('Ctrl Pts',(57.6864406075043,-55.2234346241344,-9.07966517034706));
#39146=CARTESIAN_POINT('Ctrl Pts',(55.7115103085732,-56.8731820153015,-8.96274853245577));
#39147=CARTESIAN_POINT('Ctrl Pts',(54.7447564371768,-59.2580098897298,-8.84583189456448));
#39148=CARTESIAN_POINT('Ctrl Pts',(55.0134521540628,-61.8172711292634,-8.72891525667319));
#39149=CARTESIAN_POINT('Ctrl Pts',(56.4544300397442,-63.9493126239243,-8.6119986187819));
#39150=CARTESIAN_POINT('Ctrl Pts',(58.7289322008878,-65.1529132302293,-8.4950819808906));
#39151=CARTESIAN_POINT('Ctrl Pts',(61.3022482555275,-65.145123605987,-8.37816534299932));
#39152=CARTESIAN_POINT('Ctrl Pts',(63.5694203198369,-63.9277667461252,-8.26124870510802));
#39153=CARTESIAN_POINT('Ctrl Pts',(64.9974608516679,-61.7870475945203,-8.14433206721675));
#39154=CARTESIAN_POINT('Ctrl Pts',(65.2506543952345,-59.2261870397036,-8.02741542932544));
#39155=CARTESIAN_POINT('Ctrl Pts',(64.2694756589632,-56.8472981310306,-7.91049879143416));
#39156=CARTESIAN_POINT('Ctrl Pts',(62.2845938482857,-55.2094519237375,-7.79358215354287));
#39157=CARTESIAN_POINT('Ctrl Pts',(59.7626220066562,-54.6980752792535,-7.67666551565158));
#39158=CARTESIAN_POINT('Ctrl Pts',(57.2964708372155,-55.4325509730806,-7.55974887776029));
#39159=CARTESIAN_POINT('Ctrl Pts',(55.4658552325379,-57.2420179723235,-7.442832239869));
#39160=CARTESIAN_POINT('Ctrl Pts',(54.701239676989,-59.6971936126827,-7.32591560197771));
#39161=CARTESIAN_POINT('Ctrl Pts',(55.1821426669066,-62.2293180577881,-7.20899896408642));
#39162=CARTESIAN_POINT('Ctrl Pts',(56.7959916580377,-64.2249822536134,-7.09208232619513));
#39163=CARTESIAN_POINT('Ctrl Pts',(59.9512920111792,-65.5972893108641,-6.93619347567341));
#39164=CARTESIAN_POINT('Ctrl Pts',(64.3799882857817,-64.0924457548965,-6.74133241252127));
#39165=CARTESIAN_POINT('Ctrl Pts',(65.8344796167214,-58.6247701128846,-6.50749913673868));
#39166=CARTESIAN_POINT('Ctrl Pts',(62.7388651753224,-55.1183365899423,-6.31263807358654));
#39167=CARTESIAN_POINT('Ctrl Pts',(59.3187592643186,-54.7414778160817,-6.15674922306481));
#39168=CARTESIAN_POINT('Ctrl Pts',(56.9266332065095,-55.6714869946495,-6.03983258517353));
#39169=CARTESIAN_POINT('Ctrl Pts',(55.2511528738565,-57.6299781348164,-5.92291594728223));
#39170=CARTESIAN_POINT('Ctrl Pts',(54.6947970697628,-60.1405542822466,-5.80599930939095));
#39171=CARTESIAN_POINT('Ctrl Pts',(55.3843760570615,-62.6204343466251,-5.68908267149966));
#39172=CARTESIAN_POINT('Ctrl Pts',(57.159620885591,-64.483190888477,-5.57216603360837));
#39173=CARTESIAN_POINT('Ctrl Pts',(59.6023371070298,-65.292502635446,-5.45524939571708));
#39174=CARTESIAN_POINT('Ctrl Pts',(62.1386646734039,-64.8573722208712,-5.33833275782579));
#39175=CARTESIAN_POINT('Ctrl Pts',(64.1721578713598,-63.2804354544672,-5.2214161199345));
#39176=CARTESIAN_POINT('Ctrl Pts',(65.2248498046685,-60.9322545742129,-5.10449948204321));
#39177=CARTESIAN_POINT('Ctrl Pts',(65.0492249593888,-58.3649341500245,-4.98758284415192));
#39178=CARTESIAN_POINT('Ctrl Pts',(63.6865889957319,-56.1819888648126,-4.87066620626063));
#39179=CARTESIAN_POINT('Ctrl Pts',(61.4572741020296,-54.8966206991336,-4.75374956836934));
#39180=CARTESIAN_POINT('Ctrl Pts',(58.885371453618,-54.8109981947122,-4.63683293047805));
#39181=CARTESIAN_POINT('Ctrl Pts',(56.5755050285457,-55.9452536369063,-4.51991629258676));
#39182=CARTESIAN_POINT('Ctrl Pts',(55.0706997941323,-58.0327345420765,-4.40299965469547));
#39183=CARTESIAN_POINT('Ctrl Pts',(54.7247181776535,-60.582698043192,-4.28608301680418));
#39184=CARTESIAN_POINT('Ctrl Pts',(55.6188973116942,-62.9956754944399,-4.16916637891289));
#39185=CARTESIAN_POINT('Ctrl Pts',(57.5430244076546,-64.704403039722,-4.0522497410216));
#39186=CARTESIAN_POINT('Ctrl Pts',(60.0447608860831,-65.3071770970488,-3.93533310313031));
#39187=CARTESIAN_POINT('Ctrl Pts',(62.5359710979979,-64.6622934589222,-3.81841646523902));
#39188=CARTESIAN_POINT('Ctrl Pts',(64.4310101226481,-62.9213544069835,-3.70149982734774));
#39189=CARTESIAN_POINT('Ctrl Pts',(65.2843516276165,-60.4936414068911,-3.58458318945645));
#39190=CARTESIAN_POINT('Ctrl Pts',(64.8954360900324,-57.949870550435,-3.46766655156515));
#39191=CARTESIAN_POINT('Ctrl Pts',(63.355584325901,-55.888083148428,-3.35074991367387));
#39192=CARTESIAN_POINT('Ctrl Pts',(61.0270447294087,-54.7929300306235,-3.23383327578258));
#39193=CARTESIAN_POINT('Ctrl Pts',(58.4567444358424,-54.9220255059251,-3.11691663789129));
#39194=CARTESIAN_POINT('Ctrl Pts',(56.9857510552447,-55.8039324061735,-3.03897221263043));
#39195=CARTESIAN_POINT('Ctrl Pts',(56.3967816198431,-56.3921449163111,-3.));
#39196=CARTESIAN_POINT('Ctrl Pts',(56.7766472160421,-57.2101674189746,-10.));
#39197=CARTESIAN_POINT('Ctrl Pts',(56.6836917113314,-57.2986365151465,-10.));
#39198=CARTESIAN_POINT('Ctrl Pts',(56.5950268358409,-57.39120230356,-10.));
#39199=CARTESIAN_POINT('Ctrl Pts',(56.5107709219868,-57.4874461178782,-10.));
#39200=CARTESIAN_POINT('Ctrl Pts',(56.4249560467001,-57.5854707020888,-10.));
#39201=CARTESIAN_POINT('Ctrl Pts',(56.3437142744234,-57.68731109176,-10.));
#39202=CARTESIAN_POINT('Ctrl Pts',(56.2671935602913,-57.792573893156,-10.));
#39203=CARTESIAN_POINT('Ctrl Pts',(56.1895733429177,-57.899349184244,-10.));
#39204=CARTESIAN_POINT('Ctrl Pts',(56.1168102542361,-58.00964645597,-10.));
#39205=CARTESIAN_POINT('Ctrl Pts',(56.049090461305,-58.1230979076824,-10.));
#39206=CARTESIAN_POINT('Ctrl Pts',(55.9815185974621,-58.2363015327393,-10.));
#39207=CARTESIAN_POINT('Ctrl Pts',(55.9189675098551,-58.3526462165835,-10.));
#39208=CARTESIAN_POINT('Ctrl Pts',(55.8616615643608,-58.4717999961111,-10.));
#39209=CARTESIAN_POINT('Ctrl Pts',(55.8501070017569,-58.4958248995163,-10.));
#39210=CARTESIAN_POINT('Ctrl Pts',(55.8387658201931,-58.5199640956874,-10.));
#39211=CARTESIAN_POINT('Ctrl Pts',(55.8276400825626,-58.5442149922488,-10.));
#39212=CARTESIAN_POINT('Ctrl Pts',(55.8174346017263,-58.5664599946337,-10.));
#39213=CARTESIAN_POINT('Ctrl Pts',(55.8074085198422,-58.5888034819082,-10.));
#39214=CARTESIAN_POINT('Ctrl Pts',(55.7975753646996,-58.6112157671766,-10.));
#39215=CARTESIAN_POINT('Ctrl Pts',(55.7403628737432,-58.7416177235827,-10.));
#39216=CARTESIAN_POINT('Ctrl Pts',(55.6896032280292,-58.8745016319323,-10.));
#39217=CARTESIAN_POINT('Ctrl Pts',(55.645480033527,-59.0093932220121,-10.));
#39218=CARTESIAN_POINT('Ctrl Pts',(55.6039769196502,-59.1362748108742,-10.));
#39219=CARTESIAN_POINT('Ctrl Pts',(55.5683449606977,-59.2649336678103,-10.));
#39220=CARTESIAN_POINT('Ctrl Pts',(55.5385237883193,-59.394948029667,-10.));
#39221=CARTESIAN_POINT('Ctrl Pts',(55.5083231158982,-59.5266169359948,-10.));
#39222=CARTESIAN_POINT('Ctrl Pts',(55.4840818234416,-59.6596767600327,-10.));
#39223=CARTESIAN_POINT('Ctrl Pts',(55.4657842264052,-59.7937146570425,-10.));
#39224=CARTESIAN_POINT('Ctrl Pts',(55.4495747295253,-59.9124563076013,-10.));
#39225=CARTESIAN_POINT('Ctrl Pts',(55.4380303521448,-60.0319662479349,-10.));
#39226=CARTESIAN_POINT('Ctrl Pts',(55.4311726380116,-60.1519668352251,-10.));
#39227=CARTESIAN_POINT('Ctrl Pts',(55.429455990605,-60.1820058092848,-10.));
#39228=CARTESIAN_POINT('Ctrl Pts',(55.4280331714048,-60.2120755524062,-10.));
#39229=CARTESIAN_POINT('Ctrl Pts',(55.4269048277578,-60.2421717447487,-10.));
#39230=CARTESIAN_POINT('Ctrl Pts',(55.4260974676989,-60.2637063753445,-10.));
#39231=CARTESIAN_POINT('Ctrl Pts',(55.4254409115147,-60.2852562780381,-10.));
#39232=CARTESIAN_POINT('Ctrl Pts',(55.4249357122242,-60.3067982825129,-10.));
#39233=CARTESIAN_POINT('Ctrl Pts',(55.4216904579502,-60.4451778950763,-10.));
#39234=CARTESIAN_POINT('Ctrl Pts',(55.4246782307337,-60.5834276345437,-10.));
#39235=CARTESIAN_POINT('Ctrl Pts',(55.4338329237967,-60.7211067790156,-10.));
#39236=CARTESIAN_POINT('Ctrl Pts',(55.4430905973063,-60.8603346657192,-10.));
#39237=CARTESIAN_POINT('Ctrl Pts',(55.4586544983472,-60.9989798220631,-10.));
#39238=CARTESIAN_POINT('Ctrl Pts',(55.4805057616638,-61.1366049558711,-10.));
#39239=CARTESIAN_POINT('Ctrl Pts',(55.4853225147871,-61.1669421626271,-10.));
#39240=CARTESIAN_POINT('Ctrl Pts',(55.4904449729792,-61.1972298498434,-10.));
#39241=CARTESIAN_POINT('Ctrl Pts',(55.4958732691136,-61.2274633933805,-10.));
#39242=CARTESIAN_POINT('Ctrl Pts',(55.5203481559226,-61.3637791981151,-10.));
#39243=CARTESIAN_POINT('Ctrl Pts',(55.5510361995063,-61.498994490849,-10.));
#39244=CARTESIAN_POINT('Ctrl Pts',(55.5877252702061,-61.6327571121263,-10.));
#39245=CARTESIAN_POINT('Ctrl Pts',(55.6089637062398,-61.7101891326575,-10.));
#39246=CARTESIAN_POINT('Ctrl Pts',(55.6322140625153,-61.7871343566708,-10.));
#39247=CARTESIAN_POINT('Ctrl Pts',(55.6574430485543,-61.8635234044139,-10.));
#39248=CARTESIAN_POINT('Ctrl Pts',(55.6711730738632,-61.9050955689553,-10.));
#39249=CARTESIAN_POINT('Ctrl Pts',(55.6854892106993,-61.9465029895356,-10.));
#39250=CARTESIAN_POINT('Ctrl Pts',(55.7003867816747,-61.9877342895387,-10.));
#39251=CARTESIAN_POINT('Ctrl Pts',(55.7064544836587,-62.0045275802867,-10.));
#39252=CARTESIAN_POINT('Ctrl Pts',(55.712618644672,-62.0212916526985,-10.));
#39253=CARTESIAN_POINT('Ctrl Pts',(55.7188789712335,-62.0380257298289,-10.));
#39254=CARTESIAN_POINT('Ctrl Pts',(55.7254264995218,-62.0555275074623,-10.));
#39255=CARTESIAN_POINT('Ctrl Pts',(55.7320759827005,-62.072987796165,-10.));
#39256=CARTESIAN_POINT('Ctrl Pts',(55.7388258750028,-62.090403524095,-10.));
#39257=CARTESIAN_POINT('Ctrl Pts',(55.7901008202184,-62.2227005231443,-10.));
#39258=CARTESIAN_POINT('Ctrl Pts',(55.8471813600148,-62.3524682290589,-10.));
#39259=CARTESIAN_POINT('Ctrl Pts',(55.9097891939914,-62.4793487633564,-10.));
#39260=CARTESIAN_POINT('Ctrl Pts',(55.9730108621089,-62.6074732890015,-10.));
#39261=CARTESIAN_POINT('Ctrl Pts',(56.0418689163077,-62.7326544978742,-10.));
#39262=CARTESIAN_POINT('Ctrl Pts',(56.1161301190731,-62.8545209455919,-10.));
#39263=CARTESIAN_POINT('Ctrl Pts',(56.1904609269085,-62.9765016188041,-10.));
#39264=CARTESIAN_POINT('Ctrl Pts',(56.2702052729959,-63.0951620835971,-10.));
#39265=CARTESIAN_POINT('Ctrl Pts',(56.3551790532359,-63.2101155108968,-10.));
#39266=CARTESIAN_POINT('Ctrl Pts',(56.3877839542042,-63.2542237652606,-10.));
#39267=CARTESIAN_POINT('Ctrl Pts',(56.4211592843168,-63.2977860220108,-10.));
#39268=CARTESIAN_POINT('Ctrl Pts',(56.455296464099,-63.3407794968677,-10.));
#39269=CARTESIAN_POINT('Ctrl Pts',(56.5184577271862,-63.4203268465255,-10.));
#39270=CARTESIAN_POINT('Ctrl Pts',(56.5842264360496,-63.4979275884953,-10.));
#39271=CARTESIAN_POINT('Ctrl Pts',(56.6524865899918,-63.5734972061251,-10.));
#39272=CARTESIAN_POINT('Ctrl Pts',(56.6665323550258,-63.5890470259194,-10.));
#39273=CARTESIAN_POINT('Ctrl Pts',(56.6806836439788,-63.6045108180711,-10.));
#39274=CARTESIAN_POINT('Ctrl Pts',(56.6949394989269,-63.619887800082,-10.));
#39275=CARTESIAN_POINT('Ctrl Pts',(56.7093516420952,-63.6354333613299,-10.));
#39276=CARTESIAN_POINT('Ctrl Pts',(56.7238639886949,-63.6508829927511,-10.));
#39277=CARTESIAN_POINT('Ctrl Pts',(56.7384737638415,-63.6662345726912,-10.));
#39278=CARTESIAN_POINT('Ctrl Pts',(56.8381048611188,-63.7709243943361,-10.));
#39279=CARTESIAN_POINT('Ctrl Pts',(56.9422847936492,-63.8710796498495,-10.));
#39280=CARTESIAN_POINT('Ctrl Pts',(57.0506144927706,-63.9665038599407,-10.));
#39281=CARTESIAN_POINT('Ctrl Pts',(57.1492676399244,-64.0534043010616,-10.));
#39282=CARTESIAN_POINT('Ctrl Pts',(57.2513632043421,-64.1363811929212,-10.));
#39283=CARTESIAN_POINT('Ctrl Pts',(57.3566308873088,-64.2152666810068,-10.));
#39284=CARTESIAN_POINT('Ctrl Pts',(57.4121395415194,-64.2568637519878,-10.));
#39285=CARTESIAN_POINT('Ctrl Pts',(57.4685306830645,-64.2973228450431,-10.));
#39286=CARTESIAN_POINT('Ctrl Pts',(57.5257674980437,-64.336616799743,-10.));
#39287=CARTESIAN_POINT('Ctrl Pts',(57.547470637647,-64.3515163392217,-10.));
#39288=CARTESIAN_POINT('Ctrl Pts',(57.5692953852945,-64.3662483371277,-10.));
#39289=CARTESIAN_POINT('Ctrl Pts',(57.5912397986742,-64.3808112384959,-10.));
#39290=CARTESIAN_POINT('Ctrl Pts',(57.6130039806025,-64.3952545334383,-10.));
#39291=CARTESIAN_POINT('Ctrl Pts',(57.6348798559218,-64.4095274598417,-10.));
#39292=CARTESIAN_POINT('Ctrl Pts',(57.6568590278616,-64.4236248088739,-10.));
#39293=CARTESIAN_POINT('Ctrl Pts',(57.7821905968559,-64.5040119534721,-10.));
#39294=CARTESIAN_POINT('Ctrl Pts',(57.9109399451369,-64.5787341115543,-10.));
#39295=CARTESIAN_POINT('Ctrl Pts',(58.0427132801631,-64.6475637443441,-10.));
#39296=CARTESIAN_POINT('Ctrl Pts',(58.1526798139151,-64.7050029533904,-10.));
#39297=CARTESIAN_POINT('Ctrl Pts',(58.2647532533075,-64.7583381770103,-10.));
#39298=CARTESIAN_POINT('Ctrl Pts',(58.3787241365729,-64.8074172934041,-10.));
#39299=CARTESIAN_POINT('Ctrl Pts',(58.4767840475646,-64.8496446908518,-10.));
#39300=CARTESIAN_POINT('Ctrl Pts',(58.5762489646464,-64.8887211766839,-10.));
#39301=CARTESIAN_POINT('Ctrl Pts',(58.6769607093948,-64.9246350255102,-10.));
#39302=CARTESIAN_POINT('Ctrl Pts',(64.2628730310814,-59.999902186829,-7.57968167058906));
#39303=CARTESIAN_POINT('Ctrl Pts',(64.2624542707466,-60.4879393559667,-7.60701019445077));
#39304=CARTESIAN_POINT('Ctrl Pts',(64.1786779858871,-60.9761189685309,-7.63433871831249));
#39305=CARTESIAN_POINT('Ctrl Pts',(64.0144041626786,-61.4355115568657,-7.6616672421742));
#39306=CARTESIAN_POINT('Ctrl Pts',(63.7801392459165,-62.0906345969544,-7.70063945480464));
#39307=CARTESIAN_POINT('Ctrl Pts',(63.3821699194345,-62.6872146939206,-7.73961166743506));
#39308=CARTESIAN_POINT('Ctrl Pts',(62.8672751264245,-63.1551325221511,-7.77858388006549));
#39309=CARTESIAN_POINT('Ctrl Pts',(62.3523803334146,-63.6230503503815,-7.81755609269592));
#39310=CARTESIAN_POINT('Ctrl Pts',(61.7205600738767,-63.9623059098762,-7.85652830532635));
#39311=CARTESIAN_POINT('Ctrl Pts',(61.0460813901126,-64.1330191040233,-7.89550051795678));
#39312=CARTESIAN_POINT('Ctrl Pts',(60.3716027063484,-64.3037322981704,-7.93447273058721));
#39313=CARTESIAN_POINT('Ctrl Pts',(59.654465598358,-64.3059031269698,-7.97344494321764));
#39314=CARTESIAN_POINT('Ctrl Pts',(58.9789655312245,-64.1392775723992,-8.01241715584807));
#39315=CARTESIAN_POINT('Ctrl Pts',(58.3034654640909,-63.9726520178286,-8.0513893684785));
#39316=CARTESIAN_POINT('Ctrl Pts',(57.6696024378142,-63.637230079888,-8.09036158110893));
#39317=CARTESIAN_POINT('Ctrl Pts',(57.1518835570005,-63.1724382162409,-8.12933379373936));
#39318=CARTESIAN_POINT('Ctrl Pts',(56.6341646761868,-62.7076463525939,-8.16830600636979));
#39319=CARTESIAN_POINT('Ctrl Pts',(56.2325899408361,-62.1134845632405,-8.20727821900022));
#39320=CARTESIAN_POINT('Ctrl Pts',(55.9943622305744,-61.4597935272245,-8.24625043163065));
#39321=CARTESIAN_POINT('Ctrl Pts',(55.7561345203128,-60.8061024912086,-8.28522264426108));
#39322=CARTESIAN_POINT('Ctrl Pts',(55.6812538351402,-60.0928822085302,-8.32419485689151));
#39323=CARTESIAN_POINT('Ctrl Pts',(55.7785219894409,-59.4039676536234,-8.36316706952194));
#39324=CARTESIAN_POINT('Ctrl Pts',(55.8757901437417,-58.7150530987165,-8.40213928215237));
#39325=CARTESIAN_POINT('Ctrl Pts',(56.1452071375158,-58.0504442715813,-8.4411114947828));
#39326=CARTESIAN_POINT('Ctrl Pts',(56.5551044905297,-57.4882623288071,-8.48008370741323));
#39327=CARTESIAN_POINT('Ctrl Pts',(56.9650018435436,-56.9260803860329,-8.51905592004366));
#39328=CARTESIAN_POINT('Ctrl Pts',(57.5153795557971,-56.4663253276198,-8.55802813267409));
#39329=CARTESIAN_POINT('Ctrl Pts',(58.1415437805544,-56.1630387578257,-8.59700034530452));
#39330=CARTESIAN_POINT('Ctrl Pts',(58.7677080053116,-55.8597521880315,-8.63597255793495));
#39331=CARTESIAN_POINT('Ctrl Pts',(59.4696587425724,-55.7129341068562,-8.67494477056538));
#39332=CARTESIAN_POINT('Ctrl Pts',(60.1648855564949,-55.7398422498282,-8.71391698319581));
#39333=CARTESIAN_POINT('Ctrl Pts',(60.8601123704174,-55.7667503928002,-8.75288919582624));
#39334=CARTESIAN_POINT('Ctrl Pts',(61.5486152610015,-55.9673847599195,-8.79186140845667));
#39335=CARTESIAN_POINT('Ctrl Pts',(62.1494645520024,-56.3181617324103,-8.8308336210871));
#39336=CARTESIAN_POINT('Ctrl Pts',(62.7503138430034,-56.668938704901,-8.86980583371753));
#39337=CARTESIAN_POINT('Ctrl Pts',(63.2635095344213,-57.1698582827631,-8.90877804634796));
#39338=CARTESIAN_POINT('Ctrl Pts',(63.6287282560618,-57.7620404787157,-8.94775025897839));
#39339=CARTESIAN_POINT('Ctrl Pts',(63.9939469777023,-58.3542226746683,-8.98672247160882));
#39340=CARTESIAN_POINT('Ctrl Pts',(64.2111887295655,-59.0376674887114,-9.02569468423925));
#39341=CARTESIAN_POINT('Ctrl Pts',(64.2549180718975,-59.7320390461549,-9.06466689686968));
#39342=CARTESIAN_POINT('Ctrl Pts',(64.2605339208635,-59.8212122553767,-9.0696718214428));
#39343=CARTESIAN_POINT('Ctrl Pts',(64.2632881266013,-59.9105656732725,-9.07467674601593));
#39344=CARTESIAN_POINT('Ctrl Pts',(64.2632129993401,-59.9999237120662,-9.07968167058906));
#39345=CARTESIAN_POINT('Ctrl Pts',(61.322884965569,-64.9244061944433,-10.));
#39346=CARTESIAN_POINT('Ctrl Pts',(62.1267766598728,-64.7084499564018,-9.96102778736957));
#39347=CARTESIAN_POINT('Ctrl Pts',(63.6260271020141,-63.8754856296126,-9.88308336210871));
#39348=CARTESIAN_POINT('Ctrl Pts',(65.0229772435633,-61.7140881496855,-9.76616672421742));
#39349=CARTESIAN_POINT('Ctrl Pts',(65.2388166219534,-59.1499371274841,-9.64925008632613));
#39350=CARTESIAN_POINT('Ctrl Pts',(64.2231822374133,-56.7854927040709,-9.53233344843484));
#39351=CARTESIAN_POINT('Ctrl Pts',(62.2146698199313,-55.1767965300925,-9.41541681054356));
#39352=CARTESIAN_POINT('Ctrl Pts',(59.6855379300098,-54.7019554558395,-9.29850017265226));
#39353=CARTESIAN_POINT('Ctrl Pts',(57.2303209690299,-55.4726378662523,-9.18158353476098));
#39354=CARTESIAN_POINT('Ctrl Pts',(55.4262302424911,-57.3076473811431,-9.06466689686968));
#39355=CARTESIAN_POINT('Ctrl Pts',(54.6973796557714,-59.775601760132,-8.9477502589784));
#39356=CARTESIAN_POINT('Ctrl Pts',(55.2151175549311,-62.2963084797734,-8.8308336210871));
#39357=CARTESIAN_POINT('Ctrl Pts',(56.8577277980376,-64.2771790632985,-8.71391698319582));
#39358=CARTESIAN_POINT('Ctrl Pts',(59.2390517062358,-65.2525319290857,-8.59700034530453));
#39359=CARTESIAN_POINT('Ctrl Pts',(61.7992659861865,-64.9930728587382,-8.48008370741324));
#39360=CARTESIAN_POINT('Ctrl Pts',(63.9364928774652,-63.5597974904555,-8.36316706952195));
#39361=CARTESIAN_POINT('Ctrl Pts',(65.1482937026264,-61.2896533828664,-8.24625043163066));
#39362=CARTESIAN_POINT('Ctrl Pts',(65.1497880187566,-58.7163255770949,-8.12933379373937));
#39363=CARTESIAN_POINT('Ctrl Pts',(63.9406234799139,-56.4447764036095,-8.01241715584808));
#39364=CARTESIAN_POINT('Ctrl Pts',(61.8050635175092,-55.0090188089158,-7.89550051795678));
#39365=CARTESIAN_POINT('Ctrl Pts',(59.2451498180026,-54.7465902155457,-7.7785838800655));
#39366=CARTESIAN_POINT('Ctrl Pts',(56.8627001404056,-55.7191702005741,-7.66166724217421));
#39367=CARTESIAN_POINT('Ctrl Pts',(55.217779590162,-57.6981472392852,-7.54475060428292));
#39368=CARTESIAN_POINT('Ctrl Pts',(54.6971392178688,-60.21821824206,-7.42783396639163));
#39369=CARTESIAN_POINT('Ctrl Pts',(55.4230712207726,-62.6870881580822,-7.31091732850034));
#39370=CARTESIAN_POINT('Ctrl Pts',(57.2251428783372,-64.5240383042407,-7.19400069060906));
#39371=CARTESIAN_POINT('Ctrl Pts',(59.6792195378112,-65.2979014573777,-7.07708405271776));
#39372=CARTESIAN_POINT('Ctrl Pts',(62.2094281655486,-64.8252835759928,-6.96016741482648));
#39373=CARTESIAN_POINT('Ctrl Pts',(64.2186727163164,-63.2204586132884,-6.84325077693518));
#39374=CARTESIAN_POINT('Ctrl Pts',(65.2395163218884,-60.8538584389166,-6.7263341390439));
#39375=CARTESIAN_POINT('Ctrl Pts',(65.0214094514788,-58.2965905321897,-6.6094175011526));
#39376=CARTESIAN_POINT('Ctrl Pts',(63.1773262290866,-55.3916806820179,-6.45352865063089));
#39377=CARTESIAN_POINT('Ctrl Pts',(58.6661395049216,-54.1559238915272,-6.25866758747873));
#39378=CARTESIAN_POINT('Ctrl Pts',(54.3971988313774,-57.8690311013926,-6.02483431169616));
#39379=CARTESIAN_POINT('Ctrl Pts',(54.9957837258839,-62.5079530267534,-5.82997324854401));
#39380=CARTESIAN_POINT('Ctrl Pts',(57.6170694121072,-64.7368553395382,-5.67408439802229));
#39381=CARTESIAN_POINT('Ctrl Pts',(60.1194267752203,-65.3072914717773,-5.557167760131));
#39382=CARTESIAN_POINT('Ctrl Pts',(62.6046736799591,-64.6243084010734,-5.44025112223971));
#39383=CARTESIAN_POINT('Ctrl Pts',(64.4724887605417,-62.8568826882213,-5.32333448434842));
#39384=CARTESIAN_POINT('Ctrl Pts',(65.2912291347546,-60.4165983684538,-5.20641784645713));
#39385=CARTESIAN_POINT('Ctrl Pts',(64.8649669487591,-57.8789504458245,-5.08950120856584));
#39386=CARTESIAN_POINT('Ctrl Pts',(63.2955109178121,-55.8396721751708,-4.97258457067455));
#39387=CARTESIAN_POINT('Ctrl Pts',(60.9510823423798,-54.7785639854422,-4.85566793278326));
#39388=CARTESIAN_POINT('Ctrl Pts',(58.3831733906512,-54.9449006048999,-4.73875129489197));
#39389=CARTESIAN_POINT('Ctrl Pts',(56.1953121953125,-56.2996615164319,-4.62183465700068));
#39390=CARTESIAN_POINT('Ctrl Pts',(54.9019142627768,-58.5243188117934,-4.50491801910939));
#39391=CARTESIAN_POINT('Ctrl Pts',(54.8070090534039,-61.0958980757912,-4.3880013812181));
#39392=CARTESIAN_POINT('Ctrl Pts',(55.932923519751,-63.4098412167327,-4.27108474332681));
#39393=CARTESIAN_POINT('Ctrl Pts',(58.0149603071344,-64.9221696503736,-4.15416810543553));
#39394=CARTESIAN_POINT('Ctrl Pts',(60.5636590522025,-65.2773499477182,-4.03725146754423));
#39395=CARTESIAN_POINT('Ctrl Pts',(62.9798472271926,-64.3918839378294,-3.92033482965295));
#39396=CARTESIAN_POINT('Ctrl Pts',(64.6955066967082,-62.4739345776163,-3.80341819176165));
#39397=CARTESIAN_POINT('Ctrl Pts',(65.3073040903922,-59.9743905230445,-3.68650155387037));
#39398=CARTESIAN_POINT('Ctrl Pts',(64.6714138259177,-57.4808672112921,-3.56958491597907));
#39399=CARTESIAN_POINT('Ctrl Pts',(62.9373243124707,-55.5795635648098,-3.45266827808779));
#39400=CARTESIAN_POINT('Ctrl Pts',(60.5127057471208,-54.7174568009332,-3.3357516401965));
#39401=CARTESIAN_POINT('Ctrl Pts',(57.9675484622588,-55.0972147578633,-3.21883500230521));
#39402=CARTESIAN_POINT('Ctrl Pts',(55.9002136741803,-56.629568839814,-3.10191836441392));
#39403=CARTESIAN_POINT('Ctrl Pts',(54.7966592387799,-58.9542608884761,-2.98500172652263));
#39404=CARTESIAN_POINT('Ctrl Pts',(54.9164249969225,-61.5248185706029,-2.86808508863134));
#39405=CARTESIAN_POINT('Ctrl Pts',(56.2311219369973,-63.7368377969517,-2.75116845074005));
#39406=CARTESIAN_POINT('Ctrl Pts',(58.4321698206392,-65.0704408031689,-2.63425181284876));
#39407=CARTESIAN_POINT('Ctrl Pts',(60.1446943002093,-65.1644693350243,-2.5563073875879));
#39408=CARTESIAN_POINT('Ctrl Pts',(60.9621351249183,-65.0074042178956,-2.51733517495747));
#39409=CARTESIAN_POINT('Ctrl Pts',(61.2505876634042,-64.655281295538,-10.1608882750142));
#39410=CARTESIAN_POINT('Ctrl Pts',(62.0105456807492,-64.4511273334331,-10.1219160623837));
#39411=CARTESIAN_POINT('Ctrl Pts',(63.4278602289486,-63.6636855389833,-10.0439716371229));
#39412=CARTESIAN_POINT('Ctrl Pts',(64.7484653147133,-61.6204111088842,-9.9270549992316));
#39413=CARTESIAN_POINT('Ctrl Pts',(64.9525088036914,-59.1963941165292,-9.81013836134031));
#39414=CARTESIAN_POINT('Ctrl Pts',(63.9923800964395,-56.9611695099411,-9.69322172344902));
#39415=CARTESIAN_POINT('Ctrl Pts',(62.093635370728,-55.4403905747315,-9.57630508555773));
#39416=CARTESIAN_POINT('Ctrl Pts',(59.702723671692,-54.9915001534219,-9.45938844766644));
#39417=CARTESIAN_POINT('Ctrl Pts',(57.3816873591647,-55.7200638153805,-9.34247180977515));
#39418=CARTESIAN_POINT('Ctrl Pts',(55.6761924257478,-57.4547877870635,-9.22555517188386));
#39419=CARTESIAN_POINT('Ctrl Pts',(54.9871744264961,-59.7878654019264,-9.10863853399257));
#39420=CARTESIAN_POINT('Ctrl Pts',(55.4766173080904,-62.1708123766754,-8.99172189610128));
#39421=CARTESIAN_POINT('Ctrl Pts',(57.0294568665373,-64.0434259288984,-8.87480525820999));
#39422=CARTESIAN_POINT('Ctrl Pts',(59.2806384731565,-64.9654745522983,-8.7578886203187));
#39423=CARTESIAN_POINT('Ctrl Pts',(61.7009338711017,-64.7201952415646,-8.64097198242741));
#39424=CARTESIAN_POINT('Ctrl Pts',(63.7213586651647,-63.3652501477072,-8.52405534453613));
#39425=CARTESIAN_POINT('Ctrl Pts',(64.8669330740459,-61.2191722278638,-8.40713870664483));
#39426=CARTESIAN_POINT('Ctrl Pts',(64.8683457239484,-58.7864799745289,-8.29022206875354));
#39427=CARTESIAN_POINT('Ctrl Pts',(63.7252635250725,-56.6390737773809,-8.17330543086226));
#39428=CARTESIAN_POINT('Ctrl Pts',(61.7064145601557,-55.281782113861,-8.05638879297096));
#39429=CARTESIAN_POINT('Ctrl Pts',(59.2864033155609,-55.0336955682165,-7.93947215507968));
#39430=CARTESIAN_POINT('Ctrl Pts',(57.0341574642351,-55.9531228522261,-7.82255551718839));
#39431=CARTESIAN_POINT('Ctrl Pts',(55.4791338597982,-57.823946344205,-7.7056388792971));
#39432=CARTESIAN_POINT('Ctrl Pts',(54.9869471288226,-60.2062923448016,-7.58872224140581));
#39433=CARTESIAN_POINT('Ctrl Pts',(55.6732060484796,-62.5402354614648,-7.47180560351452));
#39434=CARTESIAN_POINT('Ctrl Pts',(57.3767922575429,-64.2767940065127,-7.35488896562323));
#39435=CARTESIAN_POINT('Ctrl Pts',(59.6967505874543,-65.0083645796653,-7.23797232773194));
#39436=CARTESIAN_POINT('Ctrl Pts',(62.0886801792508,-64.5615758509794,-7.12105568984065));
#39437=CARTESIAN_POINT('Ctrl Pts',(63.9881170262568,-63.044456560552,-7.00413905194936));
#39438=CARTESIAN_POINT('Ctrl Pts',(64.9531702641583,-60.8071940174658,-6.88722241405807));
#39439=CARTESIAN_POINT('Ctrl Pts',(64.7469832044083,-58.3896839697977,-6.77030577616678));
#39440=CARTESIAN_POINT('Ctrl Pts',(63.0036814145795,-55.6435310415546,-6.61441692564505));
#39441=CARTESIAN_POINT('Ctrl Pts',(58.7390366333706,-54.4753098905259,-6.41955586249292));
#39442=CARTESIAN_POINT('Ctrl Pts',(54.7033988560207,-57.9854911915564,-6.18572258671033));
#39443=CARTESIAN_POINT('Ctrl Pts',(55.2692703445124,-62.3708902869766,-5.99086152355819));
#39444=CARTESIAN_POINT('Ctrl Pts',(57.7472995207219,-64.4779803271924,-5.83497267303646));
#39445=CARTESIAN_POINT('Ctrl Pts',(60.112899954008,-65.0172414181455,-5.71805603514517));
#39446=CARTESIAN_POINT('Ctrl Pts',(62.4623250366666,-64.3715842183384,-5.60113939725388));
#39447=CARTESIAN_POINT('Ctrl Pts',(64.2280617092367,-62.7007505101895,-5.4842227593626));
#39448=CARTESIAN_POINT('Ctrl Pts',(65.0020569077392,-60.3938307515336,-5.3673061214713));
#39449=CARTESIAN_POINT('Ctrl Pts',(64.5990904782641,-57.994868431527,-5.25038948358002));
#39450=CARTESIAN_POINT('Ctrl Pts',(63.1154071636583,-56.0670392446326,-5.13347284568872));
#39451=CARTESIAN_POINT('Ctrl Pts',(60.8991045141632,-55.0639219319788,-5.01655620779744));
#39452=CARTESIAN_POINT('Ctrl Pts',(58.471534967785,-55.2211680491245,-4.89963956990615));
#39453=CARTESIAN_POINT('Ctrl Pts',(56.4032430971049,-56.5018895985567,-4.78272293201486));
#39454=CARTESIAN_POINT('Ctrl Pts',(55.1805309638501,-58.6049666168101,-4.66580629412357));
#39455=CARTESIAN_POINT('Ctrl Pts',(55.0908124417384,-61.0360058883453,-4.54888965623228));
#39456=CARTESIAN_POINT('Ctrl Pts',(56.1551942877113,-63.2234891701099,-4.43197301834099));
#39457=CARTESIAN_POINT('Ctrl Pts',(58.1234451854266,-64.6531669813724,-4.3150563804497));
#39458=CARTESIAN_POINT('Ctrl Pts',(60.532854386736,-64.9889362354679,-4.19813974255841));
#39459=CARTESIAN_POINT('Ctrl Pts',(62.8169948847769,-64.1518620399393,-4.08122310466712));
#39460=CARTESIAN_POINT('Ctrl Pts',(64.4388914389159,-62.338730988227,-3.96430646677583));
#39461=CARTESIAN_POINT('Ctrl Pts',(65.0172533471374,-59.9757901126853,-3.84738982888454));
#39462=CARTESIAN_POINT('Ctrl Pts',(64.4161152733605,-57.6185409389093,-3.73047319099325));
#39463=CARTESIAN_POINT('Ctrl Pts',(62.7767959000222,-55.8211458920516,-3.61355655310196));
#39464=CARTESIAN_POINT('Ctrl Pts',(60.4846857428982,-55.0061543308031,-3.49663991521067));
#39465=CARTESIAN_POINT('Ctrl Pts',(58.0786244566074,-55.3651580449409,-3.37972327731938));
#39466=CARTESIAN_POINT('Ctrl Pts',(56.1242720757222,-56.8137670780251,-3.26280663942809));
#39467=CARTESIAN_POINT('Ctrl Pts',(55.0810282573051,-59.0114118263877,-3.1458900015368));
#39468=CARTESIAN_POINT('Ctrl Pts',(55.1942486683988,-61.4414853467666,-3.02897336364552));
#39469=CARTESIAN_POINT('Ctrl Pts',(56.4370957920453,-63.532614982135,-2.91205672575423));
#39470=CARTESIAN_POINT('Ctrl Pts',(58.5178536821771,-64.7933349319883,-2.79514008786294));
#39471=CARTESIAN_POINT('Ctrl Pts',(60.1367865774548,-64.8822246880949,-2.71719566260207));
#39472=CARTESIAN_POINT('Ctrl Pts',(60.9095532484437,-64.7337433741902,-2.67822344997165));
#39473=CARTESIAN_POINT('Ctrl Pts',(61.1782903612393,-64.3861563966327,-10.3217765500284));
#39474=CARTESIAN_POINT('Ctrl Pts',(61.8943147016256,-64.1938047104644,-10.2828043373979));
#39475=CARTESIAN_POINT('Ctrl Pts',(63.229693355883,-63.451885448354,-10.2048599121371));
#39476=CARTESIAN_POINT('Ctrl Pts',(64.4739533858633,-61.526734068083,-10.0879432742458));
#39477=CARTESIAN_POINT('Ctrl Pts',(64.6662009854295,-59.2428511055743,-9.97102663635449));
#39478=CARTESIAN_POINT('Ctrl Pts',(63.7615779554656,-57.1368463158114,-9.8541099984632));
#39479=CARTESIAN_POINT('Ctrl Pts',(61.9726009215247,-55.7039846193705,-9.73719336057191));
#39480=CARTESIAN_POINT('Ctrl Pts',(59.7199094133741,-55.2810448510043,-9.62027672268062));
#39481=CARTESIAN_POINT('Ctrl Pts',(57.5330537492994,-55.9674897645086,-9.50336008478933));
#39482=CARTESIAN_POINT('Ctrl Pts',(55.9261546090045,-57.6019281929839,-9.38644344689803));
#39483=CARTESIAN_POINT('Ctrl Pts',(55.2769691972207,-59.8001290437208,-9.26952680900675));
#39484=CARTESIAN_POINT('Ctrl Pts',(55.7381170612497,-62.0453162735774,-9.15261017111546));
#39485=CARTESIAN_POINT('Ctrl Pts',(57.201185935037,-63.8096727944984,-9.03569353322417));
#39486=CARTESIAN_POINT('Ctrl Pts',(59.3222252400773,-64.678417175511,-8.91877689533288));
#39487=CARTESIAN_POINT('Ctrl Pts',(61.6026017560169,-64.4473176243909,-8.80186025744159));
#39488=CARTESIAN_POINT('Ctrl Pts',(63.5062244528641,-63.1707028049589,-8.68494361955031));
#39489=CARTESIAN_POINT('Ctrl Pts',(64.5855724454654,-61.148691072861,-8.56802698165901));
#39490=CARTESIAN_POINT('Ctrl Pts',(64.5869034291403,-58.856634371963,-8.45111034376772));
#39491=CARTESIAN_POINT('Ctrl Pts',(63.5099035702312,-56.8333711511524,-8.33419370587643));
#39492=CARTESIAN_POINT('Ctrl Pts',(61.6077656028021,-55.5545454188062,-8.21727706798514));
#39493=CARTESIAN_POINT('Ctrl Pts',(59.3276568131192,-55.3208009208871,-8.10036043009385));
#39494=CARTESIAN_POINT('Ctrl Pts',(57.2056147880647,-56.1870755038781,-7.98344379220256));
#39495=CARTESIAN_POINT('Ctrl Pts',(55.7404881294344,-57.9497454491247,-7.86652715431127));
#39496=CARTESIAN_POINT('Ctrl Pts',(55.2767550397765,-60.1943664475432,-7.74961051641999));
#39497=CARTESIAN_POINT('Ctrl Pts',(55.9233408761866,-62.3933827648474,-7.63269387852869));
#39498=CARTESIAN_POINT('Ctrl Pts',(57.5284416367487,-64.0295497087847,-7.51577724063741));
#39499=CARTESIAN_POINT('Ctrl Pts',(59.7142816370973,-64.7188277019528,-7.39886060274611));
#39500=CARTESIAN_POINT('Ctrl Pts',(61.9679321929529,-64.297868125966,-7.28194396485483));
#39501=CARTESIAN_POINT('Ctrl Pts',(63.7575613361973,-62.8684545078156,-7.16502732696354));
#39502=CARTESIAN_POINT('Ctrl Pts',(64.666824206428,-60.7605295960148,-7.04811068907225));
#39503=CARTESIAN_POINT('Ctrl Pts',(64.4725569573379,-58.4827774074056,-6.93119405118095));
#39504=CARTESIAN_POINT('Ctrl Pts',(62.8300366000722,-55.8953814010913,-6.77530520065924));
#39505=CARTESIAN_POINT('Ctrl Pts',(58.8119337618197,-54.7946958895247,-6.58044413750709));
#39506=CARTESIAN_POINT('Ctrl Pts',(55.009598880664,-58.1019512817202,-6.34661086172451));
#39507=CARTESIAN_POINT('Ctrl Pts',(55.542756963141,-62.2338275471998,-6.15174979857236));
#39508=CARTESIAN_POINT('Ctrl Pts',(57.8775296293365,-64.2191053148466,-5.99586094805064));
#39509=CARTESIAN_POINT('Ctrl Pts',(60.1063731327958,-64.7271913645137,-5.87894431015935));
#39510=CARTESIAN_POINT('Ctrl Pts',(62.319976393374,-64.1188600356034,-5.76202767226806));
#39511=CARTESIAN_POINT('Ctrl Pts',(63.9836346579317,-62.5446183321576,-5.64511103437678));
#39512=CARTESIAN_POINT('Ctrl Pts',(64.7128846807238,-60.3710631346135,-5.52819439648548));
#39513=CARTESIAN_POINT('Ctrl Pts',(64.3332140077691,-58.1107864172294,-5.4112777585942));
#39514=CARTESIAN_POINT('Ctrl Pts',(62.9353034095045,-56.2944063140944,-5.2943611207029));
#39515=CARTESIAN_POINT('Ctrl Pts',(60.8471266859465,-55.3492798785154,-5.17744448281161));
#39516=CARTESIAN_POINT('Ctrl Pts',(58.5598965449188,-55.4974354933491,-5.06052784492033));
#39517=CARTESIAN_POINT('Ctrl Pts',(56.6111739988973,-56.7041176806815,-4.94361120702903));
#39518=CARTESIAN_POINT('Ctrl Pts',(55.4591476649235,-58.6856144218269,-4.82669456913774));
#39519=CARTESIAN_POINT('Ctrl Pts',(55.374615830073,-60.9761137008993,-4.70977793124646));
#39520=CARTESIAN_POINT('Ctrl Pts',(56.3774650556715,-63.0371371234872,-4.59286129335517));
#39521=CARTESIAN_POINT('Ctrl Pts',(58.2319300637188,-64.3841643123711,-4.47594465546388));
#39522=CARTESIAN_POINT('Ctrl Pts',(60.5020497212695,-64.7005225232177,-4.35902801757259));
#39523=CARTESIAN_POINT('Ctrl Pts',(62.6541425423612,-63.9118401420491,-4.2421113796813));
#39524=CARTESIAN_POINT('Ctrl Pts',(64.1822761811237,-62.2035273988379,-4.12519474179001));
#39525=CARTESIAN_POINT('Ctrl Pts',(64.7272026038827,-59.977189702326,-4.00827810389872));
#39526=CARTESIAN_POINT('Ctrl Pts',(64.1608167208033,-57.7562146665265,-3.89136146600743));
#39527=CARTESIAN_POINT('Ctrl Pts',(62.6162674875737,-56.0627282192935,-3.77444482811614));
#39528=CARTESIAN_POINT('Ctrl Pts',(60.4566657386756,-55.294851860673,-3.65752819022485));
#39529=CARTESIAN_POINT('Ctrl Pts',(58.1897004509561,-55.6331013320185,-3.54061155233356));
#39530=CARTESIAN_POINT('Ctrl Pts',(56.348330477264,-56.9979653162363,-3.42369491444227));
#39531=CARTESIAN_POINT('Ctrl Pts',(55.3653972758303,-59.0685627642994,-3.30677827655098));
#39532=CARTESIAN_POINT('Ctrl Pts',(55.4720723398751,-61.3581521229303,-3.18986163865969));
#39533=CARTESIAN_POINT('Ctrl Pts',(56.6430696470934,-63.3283921673183,-3.0729450007684));
#39534=CARTESIAN_POINT('Ctrl Pts',(58.603537543715,-64.5162290608077,-2.95602836287711));
#39535=CARTESIAN_POINT('Ctrl Pts',(60.1288788547004,-64.5999800411654,-2.87808393761625));
#39536=CARTESIAN_POINT('Ctrl Pts',(60.8569713719691,-64.4600825304849,-2.83911172498582));
#39537=CARTESIAN_POINT('Ctrl Pts',(61.1059930590745,-64.1170314977274,-10.4826648250425));
#39538=CARTESIAN_POINT('Ctrl Pts',(61.778083722502,-63.9364820874957,-10.4436926124121));
#39539=CARTESIAN_POINT('Ctrl Pts',(63.0315264828174,-63.2400853577248,-10.3657481871512));
#39540=CARTESIAN_POINT('Ctrl Pts',(64.1994414570133,-61.4330570272817,-10.2488315492599));
#39541=CARTESIAN_POINT('Ctrl Pts',(64.3798931671675,-59.2893080946195,-10.1319149113687));
#39542=CARTESIAN_POINT('Ctrl Pts',(63.5307758144917,-57.3125231216816,-10.0149982734774));
#39543=CARTESIAN_POINT('Ctrl Pts',(61.8515664723214,-55.9675786640095,-9.89808163558608));
#39544=CARTESIAN_POINT('Ctrl Pts',(59.7370951550563,-55.5705895485867,-9.78116499769479));
#39545=CARTESIAN_POINT('Ctrl Pts',(57.6844201394341,-56.2149157136367,-9.6642483598035));
#39546=CARTESIAN_POINT('Ctrl Pts',(56.1761167922612,-57.7490685989043,-9.54733172191221));
#39547=CARTESIAN_POINT('Ctrl Pts',(55.5667639679454,-59.8123926855153,-9.43041508402093));
#39548=CARTESIAN_POINT('Ctrl Pts',(55.9996168144089,-61.9198201704793,-9.31349844612963));
#39549=CARTESIAN_POINT('Ctrl Pts',(57.3729150035368,-63.5759196600984,-9.19658180823834));
#39550=CARTESIAN_POINT('Ctrl Pts',(59.3638120069981,-64.3913597987237,-9.07966517034706));
#39551=CARTESIAN_POINT('Ctrl Pts',(61.5042696409321,-64.1744400072173,-8.96274853245577));
#39552=CARTESIAN_POINT('Ctrl Pts',(63.2910902405636,-62.9761554622106,-8.84583189456448));
#39553=CARTESIAN_POINT('Ctrl Pts',(64.3042118168849,-61.0782099178583,-8.72891525667318));
#39554=CARTESIAN_POINT('Ctrl Pts',(64.3054611343321,-58.926788769397,-8.6119986187819));
#39555=CARTESIAN_POINT('Ctrl Pts',(63.2945436153898,-57.0276685249239,-8.49508198089061));
#39556=CARTESIAN_POINT('Ctrl Pts',(61.5091166454485,-55.8273087237513,-8.37816534299932));
#39557=CARTESIAN_POINT('Ctrl Pts',(59.3689103106776,-55.6079062735578,-8.26124870510803));
#39558=CARTESIAN_POINT('Ctrl Pts',(57.3770721118943,-56.42102815553,-8.14433206721674));
#39559=CARTESIAN_POINT('Ctrl Pts',(56.0018423990706,-58.0755445540445,-8.02741542932545));
#39560=CARTESIAN_POINT('Ctrl Pts',(55.5665629507304,-60.1824405502847,-7.91049879143416));
#39561=CARTESIAN_POINT('Ctrl Pts',(56.1734757038936,-62.2465300682299,-7.79358215354287));
#39562=CARTESIAN_POINT('Ctrl Pts',(57.6800910159544,-63.7823054110567,-7.67666551565158));
#39563=CARTESIAN_POINT('Ctrl Pts',(59.7318126867404,-64.4292908242403,-7.55974887776029));
#39564=CARTESIAN_POINT('Ctrl Pts',(61.847184206655,-64.0341604009526,-7.442832239869));
#39565=CARTESIAN_POINT('Ctrl Pts',(63.5270056461378,-62.6924524550791,-7.32591560197771));
#39566=CARTESIAN_POINT('Ctrl Pts',(64.3804781486979,-60.713865174564,-7.20899896408643));
#39567=CARTESIAN_POINT('Ctrl Pts',(64.1981307102675,-58.5758708450136,-7.09208232619513));
#39568=CARTESIAN_POINT('Ctrl Pts',(62.656391785565,-56.147231760628,-6.93619347567341));
#39569=CARTESIAN_POINT('Ctrl Pts',(58.8848308902688,-55.1140818885234,-6.74133241252126));
#39570=CARTESIAN_POINT('Ctrl Pts',(55.3157989053073,-58.218411371884,-6.50749913673868));
#39571=CARTESIAN_POINT('Ctrl Pts',(55.8162435817696,-62.096764807423,-6.31263807358654));
#39572=CARTESIAN_POINT('Ctrl Pts',(58.0077597379512,-63.9602303025007,-6.15674922306482));
#39573=CARTESIAN_POINT('Ctrl Pts',(60.0998463115835,-64.4371413108819,-6.03983258517352));
#39574=CARTESIAN_POINT('Ctrl Pts',(62.1776277500815,-63.8661358528684,-5.92291594728224));
#39575=CARTESIAN_POINT('Ctrl Pts',(63.7392076066267,-62.3884861541258,-5.80599930939095));
#39576=CARTESIAN_POINT('Ctrl Pts',(64.4237124537083,-60.3482955176934,-5.68908267149966));
#39577=CARTESIAN_POINT('Ctrl Pts',(64.067337537274,-58.2267044029319,-5.57216603360837));
#39578=CARTESIAN_POINT('Ctrl Pts',(62.7551996553507,-56.5217733835562,-5.45524939571708));
#39579=CARTESIAN_POINT('Ctrl Pts',(60.7951488577299,-55.634637825052,-5.33833275782579));
#39580=CARTESIAN_POINT('Ctrl Pts',(58.6482581220525,-55.7737029375737,-5.2214161199345));
#39581=CARTESIAN_POINT('Ctrl Pts',(56.8191049006898,-56.9063457628063,-5.10449948204321));
#39582=CARTESIAN_POINT('Ctrl Pts',(55.7377643659967,-58.7662622268436,-4.98758284415192));
#39583=CARTESIAN_POINT('Ctrl Pts',(55.6584192184076,-60.9162215134532,-4.87066620626063));
#39584=CARTESIAN_POINT('Ctrl Pts',(56.5997358236318,-62.8507850768644,-4.75374956836934));
#39585=CARTESIAN_POINT('Ctrl Pts',(58.340414942011,-64.1151616433698,-4.63683293047805));
#39586=CARTESIAN_POINT('Ctrl Pts',(60.471245055803,-64.4121088109674,-4.51991629258676));
#39587=CARTESIAN_POINT('Ctrl Pts',(62.4912901999455,-63.671818244159,-4.40299965469547));
#39588=CARTESIAN_POINT('Ctrl Pts',(63.9256609233314,-62.0683238094486,-4.28608301680419));
#39589=CARTESIAN_POINT('Ctrl Pts',(64.4371518606279,-59.9785892919668,-4.1691663789129));
#39590=CARTESIAN_POINT('Ctrl Pts',(63.9055181682461,-57.8938883941436,-4.0522497410216));
#39591=CARTESIAN_POINT('Ctrl Pts',(62.4557390751251,-56.3043105465354,-3.93533310313032));
#39592=CARTESIAN_POINT('Ctrl Pts',(60.428645734453,-55.5835493905429,-3.81841646523903));
#39593=CARTESIAN_POINT('Ctrl Pts',(58.3007764453048,-55.9010446190962,-3.70149982734774));
#39594=CARTESIAN_POINT('Ctrl Pts',(56.5723888788058,-57.1821635544474,-3.58458318945645));
#39595=CARTESIAN_POINT('Ctrl Pts',(55.6497662943555,-59.125713702211,-3.46766655156516));
#39596=CARTESIAN_POINT('Ctrl Pts',(55.7498960113514,-61.274818899094,-3.35074991367387));
#39597=CARTESIAN_POINT('Ctrl Pts',(56.8490435021415,-63.1241693525015,-3.23383327578258));
#39598=CARTESIAN_POINT('Ctrl Pts',(58.689221405253,-64.2391231896272,-3.11691663789129));
#39599=CARTESIAN_POINT('Ctrl Pts',(60.1209711319459,-64.3177353942359,-3.03897221263043));
#39600=CARTESIAN_POINT('Ctrl Pts',(60.8043894954946,-64.1864216867795,-3.));
#39601=CARTESIAN_POINT('Ctrl Pts',(64.2626697207193,-59.9999992453659,-8.67031832941094));
#39602=CARTESIAN_POINT('Ctrl Pts',(64.262671834753,-59.6527912162173,-8.65087842586792));
#39603=CARTESIAN_POINT('Ctrl Pts',(64.2207061795405,-59.3055836956379,-8.63143852232491));
#39604=CARTESIAN_POINT('Ctrl Pts',(64.1367666616005,-58.9688389200618,-8.6119986187819));
#39605=CARTESIAN_POINT('Ctrl Pts',(63.968488628018,-58.293748687906,-8.57302640615147));
#39606=CARTESIAN_POINT('Ctrl Pts',(63.6315161217039,-57.660708606415,-8.53405419352104));
#39607=CARTESIAN_POINT('Ctrl Pts',(63.16545870689,-57.1441285988073,-8.49508198089061));
#39608=CARTESIAN_POINT('Ctrl Pts',(62.6994012920761,-56.6275485911997,-8.45610976826018));
#39609=CARTESIAN_POINT('Ctrl Pts',(62.1042589687623,-56.2274286574755,-8.41713755562975));
#39610=CARTESIAN_POINT('Ctrl Pts',(61.4499867513102,-55.9908016155812,-8.37816534299932));
#39611=CARTESIAN_POINT('Ctrl Pts',(60.7957145338582,-55.7541745736868,-8.33919313036889));
#39612=CARTESIAN_POINT('Ctrl Pts',(60.0823124222679,-55.6810404236223,-8.30022091773846));
#39613=CARTESIAN_POINT('Ctrl Pts',(59.3936383333422,-55.7799936622521,-8.26124870510803));
#39614=CARTESIAN_POINT('Ctrl Pts',(58.7049642444165,-55.8789469008819,-8.2222764924776));
#39615=CARTESIAN_POINT('Ctrl Pts',(58.0410181781554,-56.149987528206,-8.18330427984717));
#39616=CARTESIAN_POINT('Ctrl Pts',(57.4798401928875,-56.5612605749537,-8.14433206721674));
#39617=CARTESIAN_POINT('Ctrl Pts',(56.9186622076197,-56.9725336217015,-8.10535985458631));
#39618=CARTESIAN_POINT('Ctrl Pts',(56.4602523033451,-57.524039087873,-8.06638764195588));
#39619=CARTESIAN_POINT('Ctrl Pts',(56.1585007764845,-58.1509411536655,-8.02741542932545));
#39620=CARTESIAN_POINT('Ctrl Pts',(55.8567492496238,-58.7778432194579,-7.98844321669502));
#39621=CARTESIAN_POINT('Ctrl Pts',(55.7116561001771,-59.4801418848713,-7.94947100406459));
#39622=CARTESIAN_POINT('Ctrl Pts',(55.740261650981,-60.1753061372356,-7.91049879143416));
#39623=CARTESIAN_POINT('Ctrl Pts',(55.7688672017848,-60.8704703895998,-7.87152657880373));
#39624=CARTESIAN_POINT('Ctrl Pts',(55.9711714528392,-61.5585002289149,-7.8325543661733));
#39625=CARTESIAN_POINT('Ctrl Pts',(56.3234261303765,-62.1584777057102,-7.79358215354287));
#39626=CARTESIAN_POINT('Ctrl Pts',(56.6756808079139,-62.7584551825055,-7.75460994091244));
#39627=CARTESIAN_POINT('Ctrl Pts',(57.1778859119341,-63.2703802967811,-7.71563772828201));
#39628=CARTESIAN_POINT('Ctrl Pts',(57.7709420757419,-63.6341737561162,-7.67666551565158));
#39629=CARTESIAN_POINT('Ctrl Pts',(58.3639982395497,-63.9979672154512,-7.63769330302115));
#39630=CARTESIAN_POINT('Ctrl Pts',(59.0479054631451,-64.2136290198458,-7.59872109039072));
#39631=CARTESIAN_POINT('Ctrl Pts',(59.7424209949285,-64.2556048514951,-7.55974887776029));
#39632=CARTESIAN_POINT('Ctrl Pts',(60.4369365267119,-64.2975806831444,-7.52077666512986));
#39633=CARTESIAN_POINT('Ctrl Pts',(61.1420603666835,-64.1658705420485,-7.48180445249943));
#39634=CARTESIAN_POINT('Ctrl Pts',(61.774592526583,-63.8763974805216,-7.442832239869));
#39635=CARTESIAN_POINT('Ctrl Pts',(62.4071246864826,-63.5869244189948,-7.40386002723857));
#39636=CARTESIAN_POINT('Ctrl Pts',(62.9670651663102,-63.139688437037,-7.36488781460814));
#39637=CARTESIAN_POINT('Ctrl Pts',(63.3892808233173,-62.5863058993055,-7.32591560197771));
#39638=CARTESIAN_POINT('Ctrl Pts',(63.8114964803245,-62.0329233615741,-7.28694338934728));
#39639=CARTESIAN_POINT('Ctrl Pts',(64.0959873145112,-61.373394268069,-7.24797117671685));
#39640=CARTESIAN_POINT('Ctrl Pts',(64.2078414918661,-60.6872973330581,-7.20899896408642));
#39641=CARTESIAN_POINT('Ctrl Pts',(64.2448472649471,-60.4603094092367,-7.1961054191946));
#39642=CARTESIAN_POINT('Ctrl Pts',(64.2629571388165,-60.2304135094119,-7.18321187430277));
#39643=CARTESIAN_POINT('Ctrl Pts',(64.2625444778277,-60.0004819773136,-7.17031832941094));
#39644=CARTESIAN_POINT('Ctrl Pts',(61.322884965569,-64.9244061944433,-10.));
#39645=CARTESIAN_POINT('Ctrl Pts',(61.4613623246005,-64.8748976721282,-10.));
#39646=CARTESIAN_POINT('Ctrl Pts',(61.5973330124332,-64.8193822244967,-10.));
#39647=CARTESIAN_POINT('Ctrl Pts',(61.7304725875119,-64.7581350229247,-10.));
#39648=CARTESIAN_POINT('Ctrl Pts',(61.8646633567708,-64.6964042483669,-10.));
#39649=CARTESIAN_POINT('Ctrl Pts',(61.9959787853947,-64.6288503940197,-10.));
#39650=CARTESIAN_POINT('Ctrl Pts',(62.124061050615,-64.5557090887474,-10.));
#39651=CARTESIAN_POINT('Ctrl Pts',(62.2511463812403,-64.4831370824129,-10.));
#39652=CARTESIAN_POINT('Ctrl Pts',(62.3750492404002,-64.4050637267884,-10.));
#39653=CARTESIAN_POINT('Ctrl Pts',(62.4953860081466,-64.3216816235178,-10.));
#39654=CARTESIAN_POINT('Ctrl Pts',(62.6141471290516,-64.2393912958542,-10.));
#39655=CARTESIAN_POINT('Ctrl Pts',(62.7294354075239,-64.1519298171547,-10.));
#39656=CARTESIAN_POINT('Ctrl Pts',(62.8408411996036,-64.0594534298754,-10.));
#39657=CARTESIAN_POINT('Ctrl Pts',(62.8725488799996,-64.0331333285837,-10.));
#39658=CARTESIAN_POINT('Ctrl Pts',(62.9039417776373,-64.0064068380026,-10.));
#39659=CARTESIAN_POINT('Ctrl Pts',(62.9350097493468,-63.9792772123792,-10.));
#39660=CARTESIAN_POINT('Ctrl Pts',(62.9507442400537,-63.9655373118076,-10.));
#39661=CARTESIAN_POINT('Ctrl Pts',(62.9663953835516,-63.9516940067249,-10.));
#39662=CARTESIAN_POINT('Ctrl Pts',(62.9819618294733,-63.9377477067006,-10.));
#39663=CARTESIAN_POINT('Ctrl Pts',(62.9973179297238,-63.9239898597024,-10.));
#39664=CARTESIAN_POINT('Ctrl Pts',(63.0125855686787,-63.910137153214,-10.));
#39665=CARTESIAN_POINT('Ctrl Pts',(63.0277587514538,-63.8961948001996,-10.));
#39666=CARTESIAN_POINT('Ctrl Pts',(63.1388322518447,-63.7941314443465,-10.));
#39667=CARTESIAN_POINT('Ctrl Pts',(63.2449332640284,-63.6871911500671,-10.));
#39668=CARTESIAN_POINT('Ctrl Pts',(63.3456717247427,-63.5756161384795,-10.));
#39669=CARTESIAN_POINT('Ctrl Pts',(63.4421342550849,-63.4687770239606,-10.));
#39670=CARTESIAN_POINT('Ctrl Pts',(63.5336799426146,-63.357687351767,-10.));
#39671=CARTESIAN_POINT('Ctrl Pts',(63.6201050981688,-63.2427298910755,-10.));
#39672=CARTESIAN_POINT('Ctrl Pts',(63.7063798474185,-63.1279724916591,-10.));
#39673=CARTESIAN_POINT('Ctrl Pts',(63.7875521734868,-63.0093599943829,-10.));
#39674=CARTESIAN_POINT('Ctrl Pts',(63.8633716796039,-62.8872534540177,-10.));
#39675=CARTESIAN_POINT('Ctrl Pts',(63.9290488265557,-62.7814810795189,-10.));
#39676=CARTESIAN_POINT('Ctrl Pts',(63.9907088369082,-62.673086342403,-10.));
#39677=CARTESIAN_POINT('Ctrl Pts',(64.0481572499681,-62.5622984835444,-10.));
#39678=CARTESIAN_POINT('Ctrl Pts',(64.0632545281217,-62.5331837520463,-10.));
#39679=CARTESIAN_POINT('Ctrl Pts',(64.0780607782463,-62.503903736544,-10.));
#39680=CARTESIAN_POINT('Ctrl Pts',(64.0925721116377,-62.4744625907651,-10.));
#39681=CARTESIAN_POINT('Ctrl Pts',(64.1048378651431,-62.449577362971,-10.));
#39682=CARTESIAN_POINT('Ctrl Pts',(64.1168955806734,-62.4245711361352,-10.));
#39683=CARTESIAN_POINT('Ctrl Pts',(64.1287279154018,-62.3994786971242,-10.));
#39684=CARTESIAN_POINT('Ctrl Pts',(64.1887507438292,-62.2721902797369,-10.));
#39685=CARTESIAN_POINT('Ctrl Pts',(64.2430415183514,-62.1425620239058,-10.));
#39686=CARTESIAN_POINT('Ctrl Pts',(64.2914122654767,-62.0109529642666,-10.));
#39687=CARTESIAN_POINT('Ctrl Pts',(64.3393952507057,-61.8803989426737,-10.));
#39688=CARTESIAN_POINT('Ctrl Pts',(64.3815529444373,-61.7478950157847,-10.));
#39689=CARTESIAN_POINT('Ctrl Pts',(64.4176522968207,-61.6137795372952,-10.));
#39690=CARTESIAN_POINT('Ctrl Pts',(64.4263872805874,-61.5813275277682,-10.));
#39691=CARTESIAN_POINT('Ctrl Pts',(64.434767312545,-61.5487811344807,-10.));
#39692=CARTESIAN_POINT('Ctrl Pts',(64.4427886296526,-61.5161451164515,-10.));
#39693=CARTESIAN_POINT('Ctrl Pts',(64.4762031655552,-61.3801927059519,-10.));
#39694=CARTESIAN_POINT('Ctrl Pts',(64.5033968610052,-61.2426844061195,-10.));
#39695=CARTESIAN_POINT('Ctrl Pts',(64.5243233415044,-61.1040536373285,-10.));
#39696=CARTESIAN_POINT('Ctrl Pts',(64.5357567077351,-61.0283115004466,-10.));
#39697=CARTESIAN_POINT('Ctrl Pts',(64.5453183642338,-60.9522344126642,-10.));
#39698=CARTESIAN_POINT('Ctrl Pts',(64.5529943411578,-60.8758947124787,-10.));
#39699=CARTESIAN_POINT('Ctrl Pts',(64.5578649511831,-60.8274551571315,-10.));
#39700=CARTESIAN_POINT('Ctrl Pts',(64.5619762515211,-60.7789098960979,-10.));
#39701=CARTESIAN_POINT('Ctrl Pts',(64.5653237401983,-60.7302777963119,-10.));
#39702=CARTESIAN_POINT('Ctrl Pts',(64.5666136683959,-60.7115378025806,-10.));
#39703=CARTESIAN_POINT('Ctrl Pts',(64.5677903120768,-60.6927823909094,-10.));
#39704=CARTESIAN_POINT('Ctrl Pts',(64.5688529252364,-60.674020922828,-10.));
#39705=CARTESIAN_POINT('Ctrl Pts',(64.5766121022954,-60.5370251107424,-10.));
#39706=CARTESIAN_POINT('Ctrl Pts',(64.5782806847897,-60.4000015709537,-10.));
#39707=CARTESIAN_POINT('Ctrl Pts',(64.5738795675567,-60.2633559862213,-10.));
#39708=CARTESIAN_POINT('Ctrl Pts',(64.5694908670336,-60.1270959146419,-10.));
#39709=CARTESIAN_POINT('Ctrl Pts',(64.5590665340938,-59.9912108741169,-10.));
#39710=CARTESIAN_POINT('Ctrl Pts',(64.5425762288987,-59.8561105901884,-10.));
#39711=CARTESIAN_POINT('Ctrl Pts',(64.5263562657352,-59.7232251400541,-10.));
#39712=CARTESIAN_POINT('Ctrl Pts',(64.5042673687703,-59.591098245371,-10.));
#39713=CARTESIAN_POINT('Ctrl Pts',(64.4762339973929,-59.4601379044057,-10.));
#39714=CARTESIAN_POINT('Ctrl Pts',(64.4633631459476,-59.4000105985925,-10.));
#39715=CARTESIAN_POINT('Ctrl Pts',(64.4492385854436,-59.3401295138928,-10.));
#39716=CARTESIAN_POINT('Ctrl Pts',(64.4338498151205,-59.2805360376953,-10.));
#39717=CARTESIAN_POINT('Ctrl Pts',(64.4113888497131,-59.1935552731982,-10.));
#39718=CARTESIAN_POINT('Ctrl Pts',(64.386234919835,-59.1071868765827,-10.));
#39719=CARTESIAN_POINT('Ctrl Pts',(64.3584258428979,-59.0215528078984,-10.));
#39720=CARTESIAN_POINT('Ctrl Pts',(64.3510564791945,-58.99885990806,-10.));
#39721=CARTESIAN_POINT('Ctrl Pts',(64.3435006224636,-58.9762186151633,-10.));
#39722=CARTESIAN_POINT('Ctrl Pts',(64.3357588976533,-58.9536312872786,-10.));
#39723=CARTESIAN_POINT('Ctrl Pts',(64.3287506921548,-58.9331840821199,-10.));
#39724=CARTESIAN_POINT('Ctrl Pts',(64.3215927201184,-58.912788626874,-10.));
#39725=CARTESIAN_POINT('Ctrl Pts',(64.3142878414638,-58.89245214144,-10.));
#39726=CARTESIAN_POINT('Ctrl Pts',(64.2688704537925,-58.7660119791177,-10.));
#39727=CARTESIAN_POINT('Ctrl Pts',(64.2177539118103,-58.6417791973703,-10.));
#39728=CARTESIAN_POINT('Ctrl Pts',(64.1611296886114,-58.5201308918513,-10.));
#39729=CARTESIAN_POINT('Ctrl Pts',(64.1136394178399,-58.4181054574767,-10.));
#39730=CARTESIAN_POINT('Ctrl Pts',(64.0622740603448,-58.3178981596683,-10.));
#39731=CARTESIAN_POINT('Ctrl Pts',(64.0071247424474,-58.2197495594681,-10.));
#39732=CARTESIAN_POINT('Ctrl Pts',(63.9749821324795,-58.1625457300211,-10.));
#39733=CARTESIAN_POINT('Ctrl Pts',(63.9415537977568,-58.1060415534713,-10.));
#39734=CARTESIAN_POINT('Ctrl Pts',(63.9068550908843,-58.0502878625428,-10.));
#39735=CARTESIAN_POINT('Ctrl Pts',(63.894935289402,-58.031135191228,-10.));
#39736=CARTESIAN_POINT('Ctrl Pts',(63.8828641530877,-58.0120689321377,-10.));
#39737=CARTESIAN_POINT('Ctrl Pts',(63.8706469244938,-57.9930984434797,-10.));
#39738=CARTESIAN_POINT('Ctrl Pts',(63.7998198660847,-57.8831206446772,-10.));
#39739=CARTESIAN_POINT('Ctrl Pts',(63.7241685364943,-57.776484465394,-10.));
#39740=CARTESIAN_POINT('Ctrl Pts',(63.6438531316869,-57.6735585118278,-10.));
#39741=CARTESIAN_POINT('Ctrl Pts',(63.5707659340086,-57.5798956643011,-10.));
#39742=CARTESIAN_POINT('Ctrl Pts',(63.4938156874143,-57.4893053118143,-10.));
#39743=CARTESIAN_POINT('Ctrl Pts',(63.4130998443829,-57.4020947050989,-10.));
#39744=CARTESIAN_POINT('Ctrl Pts',(63.3520427052235,-57.3361246309421,-10.));
#39745=CARTESIAN_POINT('Ctrl Pts',(63.2888302587009,-57.2720891084511,-10.));
#39746=CARTESIAN_POINT('Ctrl Pts',(63.2235668665311,-57.2100812780842,-10.));
#39747=CARTESIAN_POINT('Origin',(60.,-60.,-6.));
#39748=CARTESIAN_POINT('Origin',(60.,-60.,-2.));
#39749=CARTESIAN_POINT('Origin',(-60.,-60.,-2.));
#39750=CARTESIAN_POINT('Origin',(-60.,60.,-2.));
#39751=CARTESIAN_POINT('Origin',(60.,60.,-2.));
#39752=CARTESIAN_POINT('Origin',(46.,46.,-9.));
#39753=CARTESIAN_POINT('Ctrl Pts',(47.303382040875,49.1291532909119,-9.));
#39754=CARTESIAN_POINT('Ctrl Pts',(47.2095003437181,49.1799520323928,-9.));
#39755=CARTESIAN_POINT('Ctrl Pts',(47.1132613420209,49.2258395436386,-9.));
#39756=CARTESIAN_POINT('Ctrl Pts',(47.0150562309281,49.2669287082647,-9.));
#39757=CARTESIAN_POINT('Ctrl Pts',(46.9145918383911,49.3089631596092,-9.));
#39758=CARTESIAN_POINT('Ctrl Pts',(46.812069257442,49.3459762081224,-9.));
#39759=CARTESIAN_POINT('Ctrl Pts',(46.707872720993,49.3780464210823,-9.));
#39760=CARTESIAN_POINT('Ctrl Pts',(46.6771621977228,49.3874986836522,-9.));
#39761=CARTESIAN_POINT('Ctrl Pts',(46.6463060667852,49.3965212754824,-9.));
#39762=CARTESIAN_POINT('Ctrl Pts',(46.6153137287552,49.4051154780772,-9.));
#39763=CARTESIAN_POINT('Ctrl Pts',(46.5945556568678,49.4108717096692,-9.));
#39764=CARTESIAN_POINT('Ctrl Pts',(46.5737364779143,49.4164357562519,-9.));
#39765=CARTESIAN_POINT('Ctrl Pts',(46.5528589766229,49.4218079179609,-9.));
#39766=CARTESIAN_POINT('Ctrl Pts',(46.5322666250878,49.4271067054389,-9.));
#39767=CARTESIAN_POINT('Ctrl Pts',(46.5116250548014,49.4322168424348,-9.));
#39768=CARTESIAN_POINT('Ctrl Pts',(46.4909426777974,49.4371377247396,-9.));
#39769=CARTESIAN_POINT('Ctrl Pts',(46.381602528281,49.4631526265499,-9.));
#39770=CARTESIAN_POINT('Ctrl Pts',(46.271075774618,49.4838943672931,-9.));
#39771=CARTESIAN_POINT('Ctrl Pts',(46.159777013667,49.4994555398657,-9.));
#39772=CARTESIAN_POINT('Ctrl Pts',(46.0642245606241,49.5128151514089,-9.));
#39773=CARTESIAN_POINT('Ctrl Pts',(45.9681022304316,49.5223556770029,-9.));
#39774=CARTESIAN_POINT('Ctrl Pts',(45.8716585758946,49.5281082647279,-9.));
#39775=CARTESIAN_POINT('Ctrl Pts',(45.8389977514598,49.5300563893468,-9.));
#39776=CARTESIAN_POINT('Ctrl Pts',(45.8062999961371,49.5315698759885,-9.));
#39777=CARTESIAN_POINT('Ctrl Pts',(45.7735747590549,49.5326492595276,-9.));
#39778=CARTESIAN_POINT('Ctrl Pts',(45.7546015622976,49.5332750565604,-9.));
#39779=CARTESIAN_POINT('Ctrl Pts',(45.7356170483531,49.5337549639071,-9.));
#39780=CARTESIAN_POINT('Ctrl Pts',(45.7166296773268,49.534088921975,-9.));
#39781=CARTESIAN_POINT('Ctrl Pts',(45.6016680354385,49.536110916898,-9.));
#39782=CARTESIAN_POINT('Ctrl Pts',(45.4868632273739,49.5327830594677,-9.));
#39783=CARTESIAN_POINT('Ctrl Pts',(45.3726342188022,49.5242075664881,-9.));
#39784=CARTESIAN_POINT('Ctrl Pts',(45.2568059442603,49.5155120121138,-9.));
#39785=CARTESIAN_POINT('Ctrl Pts',(45.1415688620258,49.5014210476731,-9.));
#39786=CARTESIAN_POINT('Ctrl Pts',(45.0273402886265,49.4819915828865,-9.));
#39787=CARTESIAN_POINT('Ctrl Pts',(44.9134534204498,49.4626202397186,-9.));
#39788=CARTESIAN_POINT('Ctrl Pts',(44.8005681218786,49.4379423495987,-9.));
#39789=CARTESIAN_POINT('Ctrl Pts',(44.6890920364815,49.4079635851062,-9.));
#39790=CARTESIAN_POINT('Ctrl Pts',(44.6225621987322,49.3900720137391,-9.));
#39791=CARTESIAN_POINT('Ctrl Pts',(44.5565342440641,49.3702914035182,-9.));
#39792=CARTESIAN_POINT('Ctrl Pts',(44.4910958743778,49.348614160014,-9.));
#39793=CARTESIAN_POINT('Ctrl Pts',(44.4459975185961,49.3336747896629,-9.));
#39794=CARTESIAN_POINT('Ctrl Pts',(44.4011792119794,49.3178344584821,-9.));
#39795=CARTESIAN_POINT('Ctrl Pts',(44.3566702061303,49.3010888272762,-9.));
#39796=CARTESIAN_POINT('Ctrl Pts',(44.3429049139472,49.295909908944,-9.));
#39797=CARTESIAN_POINT('Ctrl Pts',(44.329171756633,49.2906453099285,-9.));
#39798=CARTESIAN_POINT('Ctrl Pts',(44.3154794690321,49.2852981639857,-9.));
#39799=CARTESIAN_POINT('Ctrl Pts',(44.2045205723958,49.2419662218545,-9.));
#39800=CARTESIAN_POINT('Ctrl Pts',(44.0960946986793,49.1931609847136,-9.));
#39801=CARTESIAN_POINT('Ctrl Pts',(43.9906292093804,49.1389421571216,-9.));
#39802=CARTESIAN_POINT('Ctrl Pts',(43.9680094585534,49.1273135535052,-9.));
#39803=CARTESIAN_POINT('Ctrl Pts',(43.9455258739352,49.1154357360948,-9.));
#39804=CARTESIAN_POINT('Ctrl Pts',(43.9231826707197,49.103308981174,-9.));
#39805=CARTESIAN_POINT('Ctrl Pts',(43.8230330597324,49.0489528632912,-9.));
#39806=CARTESIAN_POINT('Ctrl Pts',(43.7257027174543,48.9895994060328,-9.));
#39807=CARTESIAN_POINT('Ctrl Pts',(43.6313319971842,48.925638065059,-9.));
#39808=CARTESIAN_POINT('Ctrl Pts',(43.5349249824448,48.8602965913012,-9.));
#39809=CARTESIAN_POINT('Ctrl Pts',(43.4416061360124,48.7901458503572,-9.));
#39810=CARTESIAN_POINT('Ctrl Pts',(43.3515448917371,48.7155502884153,-9.));
#39811=CARTESIAN_POINT('Ctrl Pts',(43.3010473619187,48.673724399335,-9.));
#39812=CARTESIAN_POINT('Ctrl Pts',(43.2515743796257,48.6305002430066,-9.));
#39813=CARTESIAN_POINT('Ctrl Pts',(43.2031594672964,48.5859360444519,-9.));
#39814=CARTESIAN_POINT('Ctrl Pts',(43.1829715430466,48.5673537808187,-9.));
#39815=CARTESIAN_POINT('Ctrl Pts',(43.1629676207064,48.5485384762816,-9.));
#39816=CARTESIAN_POINT('Ctrl Pts',(43.1431502891677,48.529494156865,-9.));
#39817=CARTESIAN_POINT('Ctrl Pts',(43.1324187548122,48.5191812261005,-9.));
#39818=CARTESIAN_POINT('Ctrl Pts',(43.121743487207,48.5088025745941,-9.));
#39819=CARTESIAN_POINT('Ctrl Pts',(43.1111312671148,48.4983653312045,-9.));
#39820=CARTESIAN_POINT('Ctrl Pts',(43.0256520113981,48.4142954769306,-9.));
#39821=CARTESIAN_POINT('Ctrl Pts',(42.9441414511906,48.3263133292321,-9.));
#39822=CARTESIAN_POINT('Ctrl Pts',(42.8667459989365,48.2348514385974,-9.));
#39823=CARTESIAN_POINT('Ctrl Pts',(42.787931061766,48.1417120750572,-9.));
#39824=CARTESIAN_POINT('Ctrl Pts',(42.7133829724,48.044963650616,-9.));
#39825=CARTESIAN_POINT('Ctrl Pts',(42.6432802370783,47.9450129154862,-9.));
#39826=CARTESIAN_POINT('Ctrl Pts',(42.5726093244938,47.8442520873573,-9.));
#39827=CARTESIAN_POINT('Ctrl Pts',(42.5064555090162,47.7402361868037,-9.));
#39828=CARTESIAN_POINT('Ctrl Pts',(42.4450347854646,47.6333403909136,-9.));
#39829=CARTESIAN_POINT('Ctrl Pts',(42.4087714981893,47.5702282565925,-9.));
#39830=CARTESIAN_POINT('Ctrl Pts',(42.3741587493154,47.5061115052744,-9.));
#39831=CARTESIAN_POINT('Ctrl Pts',(42.3412476747171,47.4410620511533,-9.));
#39832=CARTESIAN_POINT('Ctrl Pts',(42.3239077246593,47.4067892630564,-9.));
#39833=CARTESIAN_POINT('Ctrl Pts',(42.3070402397616,47.3722575030078,-9.));
#39834=CARTESIAN_POINT('Ctrl Pts',(42.2906533294539,47.3374769421819,-9.));
#39835=CARTESIAN_POINT('Ctrl Pts',(42.2831049729279,47.3214558577702,-9.));
#39836=CARTESIAN_POINT('Ctrl Pts',(42.2756578447827,47.3053803342217,-9.));
#39837=CARTESIAN_POINT('Ctrl Pts',(42.2683151293564,47.2892565389712,-9.));
#39838=CARTESIAN_POINT('Ctrl Pts',(42.2158991652036,47.1741568483538,-9.));
#39839=CARTESIAN_POINT('Ctrl Pts',(42.168965298218,47.0569640824966,-9.));
#39840=CARTESIAN_POINT('Ctrl Pts',(42.1276944818575,46.9381059675892,-9.));
#39841=CARTESIAN_POINT('Ctrl Pts',(42.0863438342069,46.8190179421183,-9.));
#39842=CARTESIAN_POINT('Ctrl Pts',(42.0506775878683,46.6982573766557,-8.99999999999999));
#39843=CARTESIAN_POINT('Ctrl Pts',(42.0209156826669,46.5762184848755,-8.99999999999999));
#39844=CARTESIAN_POINT('Ctrl Pts',(41.9916665549266,46.4562822405122,-8.99999999999999));
#39845=CARTESIAN_POINT('Ctrl Pts',(41.9681196436424,46.3351105546335,-8.99999999999999));
#39846=CARTESIAN_POINT('Ctrl Pts',(41.9505275256033,46.2130543478546,-8.99999999999999));
#39847=CARTESIAN_POINT('Ctrl Pts',(41.9396355979066,46.1374848583697,-8.99999999999999));
#39848=CARTESIAN_POINT('Ctrl Pts',(41.9310272093262,46.0615758916198,-8.99999999999999));
#39849=CARTESIAN_POINT('Ctrl Pts',(41.9247720476892,45.9854081088662,-8.99999999999999));
#39850=CARTESIAN_POINT('Ctrl Pts',(41.9193705997876,45.9196358180438,-8.99999999999999));
#39851=CARTESIAN_POINT('Ctrl Pts',(41.915724009091,45.853670483811,-9.));
#39852=CARTESIAN_POINT('Ctrl Pts',(41.913803751014,45.7875629828621,-9.));
#39853=CARTESIAN_POINT('Ctrl Pts',(42.5743852316216,43.7746037524369,-9.));
#39854=CARTESIAN_POINT('Ctrl Pts',(42.6510842818103,43.6758334867864,-9.));
#39855=CARTESIAN_POINT('Ctrl Pts',(42.7325420871954,43.5810568881625,-9.));
#39856=CARTESIAN_POINT('Ctrl Pts',(42.8183507984011,43.4904132403405,-9.));
#39857=CARTESIAN_POINT('Ctrl Pts',(42.905364412483,43.3984967987608,-9.));
#39858=CARTESIAN_POINT('Ctrl Pts',(42.9968527722929,43.3108297865861,-9.));
#39859=CARTESIAN_POINT('Ctrl Pts',(43.0924206985133,43.227601359625,-9.));
#39860=CARTESIAN_POINT('Ctrl Pts',(43.132839147332,43.1924016430629,-9.));
#39861=CARTESIAN_POINT('Ctrl Pts',(43.173987598655,43.1579964196685,-9.));
#39862=CARTESIAN_POINT('Ctrl Pts',(43.2158372090038,43.1244025849901,-9.));
#39863=CARTESIAN_POINT('Ctrl Pts',(43.2398459933853,43.105130072615,-9.));
#39864=CARTESIAN_POINT('Ctrl Pts',(43.2640899712917,43.0861213997981,-9.00000000000001));
#39865=CARTESIAN_POINT('Ctrl Pts',(43.2885383440716,43.0673990171184,-9.00000000000001));
#39866=CARTESIAN_POINT('Ctrl Pts',(43.3879649260166,42.9912588775487,-9.00000000000001));
#39867=CARTESIAN_POINT('Ctrl Pts',(43.4908351416811,42.9197950946123,-9.));
#39868=CARTESIAN_POINT('Ctrl Pts',(43.5967555748348,42.8531796409371,-9.));
#39869=CARTESIAN_POINT('Ctrl Pts',(43.6847791881397,42.7978198509528,-9.));
#39870=CARTESIAN_POINT('Ctrl Pts',(43.7749100890708,42.7458091399839,-9.));
#39871=CARTESIAN_POINT('Ctrl Pts',(43.8669310813763,42.6972722115845,-9.));
#39872=CARTESIAN_POINT('Ctrl Pts',(43.9071902655099,42.6760373054098,-9.));
#39873=CARTESIAN_POINT('Ctrl Pts',(43.947811291,42.6554676190036,-9.));
#39874=CARTESIAN_POINT('Ctrl Pts',(43.9887761666103,42.6355751083769,-9.));
#39875=CARTESIAN_POINT('Ctrl Pts',(44.0111456695219,42.6247124957666,-9.));
#39876=CARTESIAN_POINT('Ctrl Pts',(44.0336177053014,42.6140518249009,-9.00000000000001));
#39877=CARTESIAN_POINT('Ctrl Pts',(44.0561893468518,42.6035951629003,-9.00000000000001));
#39878=CARTESIAN_POINT('Ctrl Pts',(44.0723891995466,42.5960903306215,-9.00000000000001));
#39879=CARTESIAN_POINT('Ctrl Pts',(44.0886318158707,42.588694547595,-9.));
#39880=CARTESIAN_POINT('Ctrl Pts',(44.1049153261628,42.5814085416912,-9.));
#39881=CARTESIAN_POINT('Ctrl Pts',(44.2166366261869,42.5314191943725,-9.));
#39882=CARTESIAN_POINT('Ctrl Pts',(44.3302925187242,42.4865883391233,-9.));
#39883=CARTESIAN_POINT('Ctrl Pts',(44.4455161968859,42.4470741286609,-9.));
#39884=CARTESIAN_POINT('Ctrl Pts',(44.5598765647727,42.4078559773457,-9.));
#39885=CARTESIAN_POINT('Ctrl Pts',(44.6757821335432,42.373874917401,-9.));
#39886=CARTESIAN_POINT('Ctrl Pts',(44.792883255394,42.3453358774941,-9.));
#39887=CARTESIAN_POINT('Ctrl Pts',(44.9068402971432,42.3175630900882,-9.));
#39888=CARTESIAN_POINT('Ctrl Pts',(45.0219302512138,42.2949440193141,-9.));
#39889=CARTESIAN_POINT('Ctrl Pts',(45.1378283160657,42.2777163964233,-9.));
#39890=CARTESIAN_POINT('Ctrl Pts',(45.2059618398419,42.2675887152119,-9.));
#39891=CARTESIAN_POINT('Ctrl Pts',(45.2743745433235,42.2593252243489,-9.00000000000001));
#39892=CARTESIAN_POINT('Ctrl Pts',(45.3429985825323,42.2529824582519,-9.00000000000001));
#39893=CARTESIAN_POINT('Ctrl Pts',(45.3908522461537,42.2485594514057,-9.00000000000001));
#39894=CARTESIAN_POINT('Ctrl Pts',(45.4388086450026,42.2450705638683,-9.00000000000001));
#39895=CARTESIAN_POINT('Ctrl Pts',(45.4868441510479,42.2425367943612,-9.00000000000001));
#39896=CARTESIAN_POINT('Ctrl Pts',(45.5023223922575,42.2417203504673,-9.00000000000001));
#39897=CARTESIAN_POINT('Ctrl Pts',(45.5178054105008,42.2410033048907,-9.00000000000001));
#39898=CARTESIAN_POINT('Ctrl Pts',(45.5332839477313,42.2403864886124,-9.00000000000001));
#39899=CARTESIAN_POINT('Ctrl Pts',(45.6490313924479,42.2357739785926,-9.00000000000001));
#39900=CARTESIAN_POINT('Ctrl Pts',(45.764669155912,42.2367543881879,-9.));
#39901=CARTESIAN_POINT('Ctrl Pts',(45.8798835216575,42.2435111643161,-9.));
#39902=CARTESIAN_POINT('Ctrl Pts',(45.9071533193596,42.24511040862,-9.));
#39903=CARTESIAN_POINT('Ctrl Pts',(45.9343993777372,42.2470334785817,-9.00000000000001));
#39904=CARTESIAN_POINT('Ctrl Pts',(45.9616174822091,42.2492832354607,-9.00000000000001));
#39905=CARTESIAN_POINT('Ctrl Pts',(46.0782918804937,42.2589271484086,-9.00000000000001));
#39906=CARTESIAN_POINT('Ctrl Pts',(46.1944539855328,42.2745701138262,-9.00000000000001));
#39907=CARTESIAN_POINT('Ctrl Pts',(46.3097410037823,42.2959688621477,-9.00000000000001));
#39908=CARTESIAN_POINT('Ctrl Pts',(46.4259783104462,42.3175439961796,-9.00000000000001));
#39909=CARTESIAN_POINT('Ctrl Pts',(46.5413268637747,42.34497071593,-9.));
#39910=CARTESIAN_POINT('Ctrl Pts',(46.6553901598249,42.3780460483423,-9.));
#39911=CARTESIAN_POINT('Ctrl Pts',(46.7119947706127,42.394459885069,-9.));
#39912=CARTESIAN_POINT('Ctrl Pts',(46.7682824036172,42.41226547109,-9.));
#39913=CARTESIAN_POINT('Ctrl Pts',(46.8242014173664,42.4314415738847,-9.));
#39914=CARTESIAN_POINT('Ctrl Pts',(46.8468220071947,42.4391987699927,-9.));
#39915=CARTESIAN_POINT('Ctrl Pts',(46.8693822489463,42.4471802617996,-9.00000000000001));
#39916=CARTESIAN_POINT('Ctrl Pts',(46.8918786073677,42.4553847402839,-9.00000000000001));
#39917=CARTESIAN_POINT('Ctrl Pts',(46.9070987891954,42.4609355788682,-9.00000000000001));
#39918=CARTESIAN_POINT('Ctrl Pts',(46.9222893594991,42.4665884167866,-9.00000000000001));
#39919=CARTESIAN_POINT('Ctrl Pts',(46.9374364480238,42.4723378131064,-9.00000000000001));
#39920=CARTESIAN_POINT('Ctrl Pts',(47.0458970233733,42.5135063077472,-9.00000000000001));
#39921=CARTESIAN_POINT('Ctrl Pts',(47.1523003889298,42.559683022919,-9.));
#39922=CARTESIAN_POINT('Ctrl Pts',(47.2563046800238,42.6106192638709,-9.));
#39923=CARTESIAN_POINT('Ctrl Pts',(47.360207427149,42.661505773528,-9.));
#39924=CARTESIAN_POINT('Ctrl Pts',(47.4617165213352,42.7171431270938,-9.00000000000001));
#39925=CARTESIAN_POINT('Ctrl Pts',(47.5604619593116,42.7773262218468,-9.00000000000001));
#39926=CARTESIAN_POINT('Ctrl Pts',(47.6578154101236,42.8366609321364,-9.00000000000001));
#39927=CARTESIAN_POINT('Ctrl Pts',(47.7524831733156,42.9004147535575,-9.00000000000001));
#39928=CARTESIAN_POINT('Ctrl Pts',(47.8440725207098,42.9684235448621,-9.00000000000001));
#39929=CARTESIAN_POINT('Ctrl Pts',(47.8943346524018,43.0057452085929,-9.00000000000001));
#39930=CARTESIAN_POINT('Ctrl Pts',(47.9436689753247,43.0443487994871,-9.));
#39931=CARTESIAN_POINT('Ctrl Pts',(47.992004612389,43.0842104204041,-9.));
#39932=CARTESIAN_POINT('Ctrl Pts',(48.0190276146188,43.1064958548445,-9.));
#39933=CARTESIAN_POINT('Ctrl Pts',(48.0457383875639,43.1291745351713,-9.));
#39934=CARTESIAN_POINT('Ctrl Pts',(48.0721238936586,43.1522425378067,-9.));
#39935=CARTESIAN_POINT('Ctrl Pts',(48.0885406740473,43.166595202937,-9.));
#39936=CARTESIAN_POINT('Ctrl Pts',(48.1048350306298,43.1811018865408,-9.));
#39937=CARTESIAN_POINT('Ctrl Pts',(48.1209818661767,43.195741480298,-9.));
#39938=CARTESIAN_POINT('Ctrl Pts',(48.203597770096,43.2706455237401,-9.));
#39939=CARTESIAN_POINT('Ctrl Pts',(48.2824577883745,43.3491133390206,-9.00000000000001));
#39940=CARTESIAN_POINT('Ctrl Pts',(48.3572276601944,43.4309575696696,-9.00000000000001));
#39941=CARTESIAN_POINT('Ctrl Pts',(48.4308859028047,43.5115849942012,-9.00000000000001));
#39942=CARTESIAN_POINT('Ctrl Pts',(48.5005752103064,43.595489772052,-9.));
#39943=CARTESIAN_POINT('Ctrl Pts',(48.5659337048761,43.6825193013962,-9.));
#39944=CARTESIAN_POINT('Ctrl Pts',(48.6294063439469,43.767037678708,-9.));
#39945=CARTESIAN_POINT('Ctrl Pts',(48.6887947814722,43.8545036158363,-9.));
#39946=CARTESIAN_POINT('Ctrl Pts',(48.7437218093839,43.9447943433075,-9.));
#39947=CARTESIAN_POINT('Ctrl Pts',(48.7713759357979,43.9902530416283,-9.));
#39948=CARTESIAN_POINT('Ctrl Pts',(48.7978984149478,44.0364279976715,-9.));
#39949=CARTESIAN_POINT('Ctrl Pts',(48.8232361680781,44.0833046267998,-9.));
#39950=CARTESIAN_POINT('Ctrl Pts',(48.8494363766439,44.1317768592706,-9.));
#39951=CARTESIAN_POINT('Ctrl Pts',(48.8743697772796,44.1809994232774,-9.));
#39952=CARTESIAN_POINT('Ctrl Pts',(48.8980277622168,44.2309202005125,-9.));
#39953=CARTESIAN_POINT('Origin',(46.,46.,2.76038497140452));
#39954=CARTESIAN_POINT('Ctrl Pts',(41.9098427756084,46.0018622022123,-0.364615028595478));
#39955=CARTESIAN_POINT('Ctrl Pts',(41.9091327304014,46.1207445798862,-0.370425837919348));
#39956=CARTESIAN_POINT('Ctrl Pts',(41.9672599456507,47.5746593135514,-0.441524166511648));
#39957=CARTESIAN_POINT('Ctrl Pts',(43.7008748484235,50.2221781462026,-0.57791001437238));
#39958=CARTESIAN_POINT('Ctrl Pts',(48.2448533065531,50.250832896341,-0.773772572177673));
#39959=CARTESIAN_POINT('Ctrl Pts',(50.7830589135395,46.4820553202928,-0.969635129982967));
#39960=CARTESIAN_POINT('Ctrl Pts',(49.0478253450961,42.2823235547161,-1.16549768778826));
#39961=CARTESIAN_POINT('Ctrl Pts',(44.589457028671,41.4043184071032,-1.36136024559355));
#39962=CARTESIAN_POINT('Ctrl Pts',(42.1450237582726,43.8716100607599,-1.51106602586263));
#39963=CARTESIAN_POINT('Ctrl Pts',(41.9140059020135,45.6034148009506,-1.59548428686327));
#39964=CARTESIAN_POINT('Ctrl Pts',(41.9171329418229,45.9966889238588,-1.61461502859548));
#39965=CARTESIAN_POINT('Ctrl Pts',(41.9194198683446,45.9961669413359,-0.260384971404518));
#39966=CARTESIAN_POINT('Ctrl Pts',(41.9254629731548,46.896854157291,-0.304165019473208));
#39967=CARTESIAN_POINT('Ctrl Pts',(42.657307638586,49.1524155369128,-0.413232586810329));
#39968=CARTESIAN_POINT('Ctrl Pts',(46.3558078761971,50.7932688919524,-0.58758767341588));
#39969=CARTESIAN_POINT('Ctrl Pts',(50.1895250164382,48.3572314578353,-0.783450231221173));
#39970=CARTESIAN_POINT('Ctrl Pts',(50.281582214734,43.813490556254,-0.979312789026467));
#39971=CARTESIAN_POINT('Ctrl Pts',(46.5474666641534,41.224098161527,-1.17517534683176));
#39972=CARTESIAN_POINT('Ctrl Pts',(42.7307414732583,42.7400789827082,-1.35219940762444));
#39973=CARTESIAN_POINT('Ctrl Pts',(41.9246669057656,45.0485594281921,-1.4639359491487));
#39974=CARTESIAN_POINT('Ctrl Pts',(41.9169756956685,46.0033346419049,-1.51038497140452));
#39975=CARTESIAN_POINT('Ctrl Pts',(48.5732344270147,48.2065515280923,5.55111512312578E-16));
#39976=CARTESIAN_POINT('Ctrl Pts',(49.2973603516437,47.3620909591791,-0.0652875192684306));
#39977=CARTESIAN_POINT('Ctrl Pts',(49.8377925944869,44.9184923727932,-0.195862557805293));
#39978=CARTESIAN_POINT('Ctrl Pts',(47.2195282996038,42.1996736729428,-0.391725115610586));
#39979=CARTESIAN_POINT('Ctrl Pts',(43.5104542156236,42.8839736999474,-0.58758767341588));
#39980=CARTESIAN_POINT('Ctrl Pts',(42.0262713464695,46.3485997621082,-0.783450231221173));
#39981=CARTESIAN_POINT('Ctrl Pts',(44.0921763812591,49.5035809965949,-0.979312789026468));
#39982=CARTESIAN_POINT('Ctrl Pts',(47.8627886158846,49.5273588275085,-1.17517534683176));
#39983=CARTESIAN_POINT('Ctrl Pts',(49.9690021914738,46.4000115108843,-1.37103790463705));
#39984=CARTESIAN_POINT('Ctrl Pts',(48.5290981550892,42.9150566143449,-1.56690046244235));
#39985=CARTESIAN_POINT('Ctrl Pts',(44.8295255723225,42.1864842889787,-1.76276302024764));
#39986=CARTESIAN_POINT('Ctrl Pts',(42.175734997888,44.8650909885955,-1.95862557805293));
#39987=CARTESIAN_POINT('Ctrl Pts',(42.9387745105419,48.5577202457448,-2.15448813585823));
#39988=CARTESIAN_POINT('Ctrl Pts',(46.4369034383315,49.9651124328758,-2.35035069366352));
#39989=CARTESIAN_POINT('Ctrl Pts',(49.5446749708226,47.8298347952992,-2.54621325146882));
#39990=CARTESIAN_POINT('Ctrl Pts',(49.4854159118642,44.0596670739996,-2.74207580927411));
#39991=CARTESIAN_POINT('Ctrl Pts',(46.3120712712219,42.0231137852872,-2.9379383670794));
#39992=CARTESIAN_POINT('Ctrl Pts',(42.8599030363351,43.5397550088008,-3.1338009248847));
#39993=CARTESIAN_POINT('Ctrl Pts',(42.2132908762849,47.2545310563557,-3.32966348268999));
#39994=CARTESIAN_POINT('Ctrl Pts',(44.9499580211573,49.8484315832432,-3.52552604049528));
#39995=CARTESIAN_POINT('Ctrl Pts',(48.6247973634805,49.0039062645874,-3.72138859830058));
#39996=CARTESIAN_POINT('Ctrl Pts',(49.9544810003903,45.4755059401351,-3.91725115610587));
#39997=CARTESIAN_POINT('Ctrl Pts',(47.7509876224225,42.415720949153,-4.11311371391117));
#39998=CARTESIAN_POINT('Ctrl Pts',(43.9830540035483,42.5583517256725,-4.30897627171646));
#39999=CARTESIAN_POINT('Ctrl Pts',(42.01718422667,45.7759631591032,-4.50483882952175));
#40000=CARTESIAN_POINT('Ctrl Pts',(43.6098074945965,49.193742909423,-4.70070138732704));
#40001=CARTESIAN_POINT('Ctrl Pts',(47.3379760358727,49.7580359388642,-4.89656394513234));
#40002=CARTESIAN_POINT('Ctrl Pts',(49.8707143391289,46.9646680784839,-5.09242650293763));
#40003=CARTESIAN_POINT('Ctrl Pts',(48.945117923424,43.3094063135909,-5.28828906074292));
#40004=CARTESIAN_POINT('Ctrl Pts',(45.3881716774698,42.0580867456233,-5.48415161854822));
#40005=CARTESIAN_POINT('Ctrl Pts',(42.3778705394672,44.3287153991906,-5.68001417635351));
#40006=CARTESIAN_POINT('Ctrl Pts',(42.6038031037161,48.0925726868875,-5.87587673415881));
#40007=CARTESIAN_POINT('Ctrl Pts',(45.864107183199,49.9867966215158,-6.07173929196409));
#40008=CARTESIAN_POINT('Ctrl Pts',(49.2458264323451,48.3189707046506,-6.26760184976939));
#40009=CARTESIAN_POINT('Ctrl Pts',(49.7275240173135,44.5792336070115,-6.46346440757468));
#40010=CARTESIAN_POINT('Ctrl Pts',(46.8788225841872,42.1088964537141,-6.65932696537998));
#40011=CARTESIAN_POINT('Ctrl Pts',(43.2449255924472,43.1151116077546,-6.85518952318527));
#40012=CARTESIAN_POINT('Ctrl Pts',(42.0725845216841,46.6988625619225,-7.05105208099057));
#40013=CARTESIAN_POINT('Ctrl Pts',(44.4092330005664,49.6582092212329,-7.24691463879585));
#40014=CARTESIAN_POINT('Ctrl Pts',(48.1671818964547,49.3490810528002,-7.44277719660116));
#40015=CARTESIAN_POINT('Ctrl Pts',(49.9888141460323,46.0476882843631,-7.63863975440645));
#40016=CARTESIAN_POINT('Ctrl Pts',(48.2466406173425,42.703665807707,-7.83450231221174));
#40017=CARTESIAN_POINT('Ctrl Pts',(44.4970847166944,42.304836504839,-8.03036487001704));
#40018=CARTESIAN_POINT('Ctrl Pts',(42.090520508291,45.2074018487415,-8.22622742782232));
#40019=CARTESIAN_POINT('Ctrl Pts',(43.1765285507875,48.8183115043247,-8.42208998562762));
#40020=CARTESIAN_POINT('Ctrl Pts',(46.7860126959185,49.9107832013404,-8.61795254343292));
#40021=CARTESIAN_POINT('Ctrl Pts',(49.691563339236,47.5099066949763,-8.81381510123821));
#40022=CARTESIAN_POINT('Ctrl Pts',(49.3022537239607,43.7583823233551,-9.0096776590435));
#40023=CARTESIAN_POINT('Ctrl Pts',(45.955486114933,42.0129799022276,-9.20554021684879));
#40024=CARTESIAN_POINT('Ctrl Pts',(43.7634250628647,43.2205019121706,-9.33611525538566));
#40025=CARTESIAN_POINT('Ctrl Pts',(43.1574106092752,44.1533569326372,-9.40140277465409));
#40026=CARTESIAN_POINT('Ctrl Pts',(48.7491609934165,48.3574087643591,0.133800924884696));
#40027=CARTESIAN_POINT('Ctrl Pts',(49.5227938678302,47.4552142218945,0.0685134056162651));
#40028=CARTESIAN_POINT('Ctrl Pts',(50.1001743140156,44.8445519958907,-0.0620616329205973));
#40029=CARTESIAN_POINT('Ctrl Pts',(47.3029048564098,41.9398534424552,-0.257924190725891));
#40030=CARTESIAN_POINT('Ctrl Pts',(43.3402492637749,42.6709376073043,-0.453786748531184));
#40031=CARTESIAN_POINT('Ctrl Pts',(41.7545959676198,46.3724327866287,-0.649649306336477));
#40032=CARTESIAN_POINT('Ctrl Pts',(43.9617425369805,49.7431133797975,-0.845511864141772));
#40033=CARTESIAN_POINT('Ctrl Pts',(47.9901435127741,49.7685168504526,-1.04137442194706));
#40034=CARTESIAN_POINT('Ctrl Pts',(50.2403544321623,46.4273594473539,-1.23723697975236));
#40035=CARTESIAN_POINT('Ctrl Pts',(48.7020072184249,42.7041455944686,-1.43309953755765));
#40036=CARTESIAN_POINT('Ctrl Pts',(44.7495027244386,41.9257623283536,-1.62896209536294));
#40037=CARTESIAN_POINT('Ctrl Pts',(41.9142781310867,44.7874996726008,-1.82482465316824));
#40038=CARTESIAN_POINT('Ctrl Pts',(42.7294850327982,48.7325861405604,-2.02068721097353));
#40039=CARTESIAN_POINT('Ctrl Pts',(46.4667735974386,50.2361987390397,-2.21654976877882));
#40040=CARTESIAN_POINT('Ctrl Pts',(49.7870168616665,47.9549367095438,-2.41241232658412));
#40041=CARTESIAN_POINT('Ctrl Pts',(49.7237063868474,43.9270106375071,-2.60827488438941));
#40042=CARTESIAN_POINT('Ctrl Pts',(46.3334069204898,41.7512225306933,-2.80413744219471));
#40043=CARTESIAN_POINT('Ctrl Pts',(42.6452212836014,43.3715532898804,-3.));
#40044=CARTESIAN_POINT('Ctrl Pts',(41.954401625036,47.3403006772158,-3.19586255780529));
#40045=CARTESIAN_POINT('Ctrl Pts',(44.8781688837292,50.1115406678118,-3.39172511561059));
#40046=CARTESIAN_POINT('Ctrl Pts',(48.8042491782122,49.2092769488025,-3.58758767341588));
#40047=CARTESIAN_POINT('Ctrl Pts',(50.2248404581203,45.4396473964744,-3.78345023122117));
#40048=CARTESIAN_POINT('Ctrl Pts',(47.8706989231075,42.1706714115666,-3.97931278902647));
#40049=CARTESIAN_POINT('Ctrl Pts',(43.8451596943284,42.3230535510061,-4.17517534683176));
#40050=CARTESIAN_POINT('Ctrl Pts',(41.7448875807613,45.7606462366524,-4.37103790463706));
#40051=CARTESIAN_POINT('Ctrl Pts',(43.44639511518,49.4120923214029,-4.56690046244234));
#40052=CARTESIAN_POINT('Ctrl Pts',(47.4294506125564,50.0149648654316,-4.76276302024764));
#40053=CARTESIAN_POINT('Ctrl Pts',(50.1353468483384,47.0306203838718,-4.95862557805293));
#40054=CARTESIAN_POINT('Ctrl Pts',(49.1464693737532,43.1254561441609,-5.15448813585823));
#40055=CARTESIAN_POINT('Ctrl Pts',(45.3463422759663,41.7885865179659,-5.35035069366352));
#40056=CARTESIAN_POINT('Ctrl Pts',(42.1302332498505,44.2144532246239,-5.54621325146881));
#40057=CARTESIAN_POINT('Ctrl Pts',(42.371612343125,48.2356374321302,-5.74207580927411));
#40058=CARTESIAN_POINT('Ctrl Pts',(45.8548164802582,50.2593654295507,-5.9379383670794));
#40059=CARTESIAN_POINT('Ctrl Pts',(49.4677366840439,48.477513800986,-6.1338009248847));
#40060=CARTESIAN_POINT('Ctrl Pts',(49.9823669086808,44.482098829646,-6.32966348268999));
#40061=CARTESIAN_POINT('Ctrl Pts',(46.9389058156602,41.8428699777639,-6.52552604049529));
#40062=CARTESIAN_POINT('Ctrl Pts',(43.0565670132156,42.9178779224082,-6.72138859830057));
#40063=CARTESIAN_POINT('Ctrl Pts',(41.8040754761498,46.7466423093156,-6.91725115610587));
#40064=CARTESIAN_POINT('Ctrl Pts',(44.3004756432042,49.9083132073737,-7.11311371391116));
#40065=CARTESIAN_POINT('Ctrl Pts',(48.3153475147166,49.5780506033531,-7.30897627171646));
#40066=CARTESIAN_POINT('Ctrl Pts',(50.2615208879286,46.0509486309672,-7.50483882952175));
#40067=CARTESIAN_POINT('Ctrl Pts',(48.4002386594014,42.4783024478534,-7.70070138732704));
#40068=CARTESIAN_POINT('Ctrl Pts',(44.394333594368,42.0522060335642,-7.89656394513234));
#40069=CARTESIAN_POINT('Ctrl Pts',(41.8232377080245,45.1532135984121,-8.09242650293763));
#40070=CARTESIAN_POINT('Ctrl Pts',(42.9834938112478,49.0109934694039,-8.28828906074292));
#40071=CARTESIAN_POINT('Ctrl Pts',(46.8397507126687,50.1781551334624,-8.48415161854822));
#40072=CARTESIAN_POINT('Ctrl Pts',(49.9439476755051,47.613135805253,-8.68001417635351));
#40073=CARTESIAN_POINT('Ctrl Pts',(49.5280217896079,43.6051276890717,-8.8758767341588));
#40074=CARTESIAN_POINT('Ctrl Pts',(45.9524427952592,41.7403958155962,-9.0717392919641));
#40075=CARTESIAN_POINT('Ctrl Pts',(43.6105151899593,43.0304735378497,-9.20231433050096));
#40076=CARTESIAN_POINT('Ctrl Pts',(42.963068816724,44.0271058725704,-9.26760184976939));
#40077=CARTESIAN_POINT('Ctrl Pts',(48.9250875598184,48.5082660006259,0.267601849769392));
#40078=CARTESIAN_POINT('Ctrl Pts',(49.7482273840168,47.54833748461,0.202314330500961));
#40079=CARTESIAN_POINT('Ctrl Pts',(50.3625560335442,44.7706116189882,0.0717392919640985));
#40080=CARTESIAN_POINT('Ctrl Pts',(47.3862814132159,41.6800332119675,-0.124123265841195));
#40081=CARTESIAN_POINT('Ctrl Pts',(43.1700443119262,42.4579015146611,-0.319985823646489));
#40082=CARTESIAN_POINT('Ctrl Pts',(41.4829205887701,46.3962658111493,-0.515848381451782));
#40083=CARTESIAN_POINT('Ctrl Pts',(43.831308692702,49.982645763,-0.711710939257075));
#40084=CARTESIAN_POINT('Ctrl Pts',(48.1174984096636,50.0096748733969,-0.90757349706237));
#40085=CARTESIAN_POINT('Ctrl Pts',(50.5117066728509,46.4547073838233,-1.10343605486766));
#40086=CARTESIAN_POINT('Ctrl Pts',(48.8749162817605,42.4932345745924,-1.29929861267296));
#40087=CARTESIAN_POINT('Ctrl Pts',(44.6694798765548,41.6650403677284,-1.49516117047825));
#40088=CARTESIAN_POINT('Ctrl Pts',(41.6528212642855,44.7099083566062,-1.69102372828354));
#40089=CARTESIAN_POINT('Ctrl Pts',(42.5201955550544,48.9074520353761,-1.88688628608884));
#40090=CARTESIAN_POINT('Ctrl Pts',(46.4966437565457,50.5072850452035,-2.08274884389413));
#40091=CARTESIAN_POINT('Ctrl Pts',(50.0293587525104,48.0800386237884,-2.27861140169942));
#40092=CARTESIAN_POINT('Ctrl Pts',(49.9619968618307,43.7943542010146,-2.47447395950472));
#40093=CARTESIAN_POINT('Ctrl Pts',(46.3547425697576,41.4793312760994,-2.67033651731001));
#40094=CARTESIAN_POINT('Ctrl Pts',(42.4305395308676,43.20335157096,-2.86619907511531));
#40095=CARTESIAN_POINT('Ctrl Pts',(41.6955123737871,47.4260702980758,-3.0620616329206));
#40096=CARTESIAN_POINT('Ctrl Pts',(44.8063797463012,50.3746497523805,-3.25792419072589));
#40097=CARTESIAN_POINT('Ctrl Pts',(48.9837009929438,49.4146476330176,-3.45378674853119));
#40098=CARTESIAN_POINT('Ctrl Pts',(50.4951999158503,45.4037888528138,-3.64964930633648));
#40099=CARTESIAN_POINT('Ctrl Pts',(47.9904102237924,41.9256218739801,-3.84551186414177));
#40100=CARTESIAN_POINT('Ctrl Pts',(43.7072653851086,42.0877553763397,-4.04137442194707));
#40101=CARTESIAN_POINT('Ctrl Pts',(41.4725909348526,45.7453293142015,-4.23723697975236));
#40102=CARTESIAN_POINT('Ctrl Pts',(43.2829827357634,49.6304417333827,-4.43309953755765));
#40103=CARTESIAN_POINT('Ctrl Pts',(47.5209251892401,50.271893791999,-4.62896209536295));
#40104=CARTESIAN_POINT('Ctrl Pts',(50.399979357548,47.0965726892597,-4.82482465316823));
#40105=CARTESIAN_POINT('Ctrl Pts',(49.3478208240825,42.9415059747309,-5.02068721097354));
#40106=CARTESIAN_POINT('Ctrl Pts',(45.3045128744628,41.5190862903084,-5.21654976877882));
#40107=CARTESIAN_POINT('Ctrl Pts',(41.8825959602337,44.1001910500571,-5.41241232658413));
#40108=CARTESIAN_POINT('Ctrl Pts',(42.1394215825338,48.3787021773728,-5.60827488438941));
#40109=CARTESIAN_POINT('Ctrl Pts',(45.8455257773174,50.5319342375856,-5.80413744219471));
#40110=CARTESIAN_POINT('Ctrl Pts',(49.6896469357427,48.6360568973213,-5.99999999999999));
#40111=CARTESIAN_POINT('Ctrl Pts',(50.2372098000482,44.3849640522804,-6.1958625578053));
#40112=CARTESIAN_POINT('Ctrl Pts',(46.9989890471331,41.5768435018138,-6.39172511561059));
#40113=CARTESIAN_POINT('Ctrl Pts',(42.8682084339841,42.7206442370619,-6.58758767341588));
#40114=CARTESIAN_POINT('Ctrl Pts',(41.5355664306156,46.7944220567085,-6.78345023122118));
#40115=CARTESIAN_POINT('Ctrl Pts',(44.191718285842,50.1584171935145,-6.97931278902647));
#40116=CARTESIAN_POINT('Ctrl Pts',(48.4635131329785,49.8070201539059,-7.17517534683176));
#40117=CARTESIAN_POINT('Ctrl Pts',(50.5342276298249,46.0542089775713,-7.37103790463706));
#40118=CARTESIAN_POINT('Ctrl Pts',(48.5538367014603,42.2529390879997,-7.56690046244235));
#40119=CARTESIAN_POINT('Ctrl Pts',(44.2915824720416,41.7995755622895,-7.76276302024764));
#40120=CARTESIAN_POINT('Ctrl Pts',(41.5559549077579,45.0990253480827,-7.95862557805293));
#40121=CARTESIAN_POINT('Ctrl Pts',(42.790459071708,49.2036754344831,-8.15448813585823));
#40122=CARTESIAN_POINT('Ctrl Pts',(46.8934887294189,50.4455270655844,-8.35035069366353));
#40123=CARTESIAN_POINT('Ctrl Pts',(50.1963320117741,47.7163649155299,-8.54621325146881));
#40124=CARTESIAN_POINT('Ctrl Pts',(49.7537898552552,43.4518730547882,-8.74207580927411));
#40125=CARTESIAN_POINT('Ctrl Pts',(45.9493994755854,41.4678117289649,-8.93793836707941));
#40126=CARTESIAN_POINT('Ctrl Pts',(43.4576053170538,42.8404451635287,-9.06851340561627));
#40127=CARTESIAN_POINT('Ctrl Pts',(42.7687270241728,43.9008548125037,-9.1338009248847));
#40128=CARTESIAN_POINT('Ctrl Pts',(49.1010141262202,48.6591232368927,0.401402774654088));
#40129=CARTESIAN_POINT('Ctrl Pts',(49.9736609002034,47.6414607473255,0.336115255385657));
#40130=CARTESIAN_POINT('Ctrl Pts',(50.6249377530729,44.6966712420858,0.205540216848794));
#40131=CARTESIAN_POINT('Ctrl Pts',(47.4696579700219,41.4202129814799,0.0096776590435005));
#40132=CARTESIAN_POINT('Ctrl Pts',(42.9998393600774,42.2448654220179,-0.186184898761793));
#40133=CARTESIAN_POINT('Ctrl Pts',(41.2112452099204,46.4200988356699,-0.382047456567087));
#40134=CARTESIAN_POINT('Ctrl Pts',(43.7008748484235,50.2221781462026,-0.57791001437238));
#40135=CARTESIAN_POINT('Ctrl Pts',(48.2448533065531,50.250832896341,-0.773772572177673));
#40136=CARTESIAN_POINT('Ctrl Pts',(50.7830589135395,46.4820553202928,-0.969635129982967));
#40137=CARTESIAN_POINT('Ctrl Pts',(49.0478253450961,42.2823235547161,-1.16549768778826));
#40138=CARTESIAN_POINT('Ctrl Pts',(44.589457028671,41.4043184071032,-1.36136024559355));
#40139=CARTESIAN_POINT('Ctrl Pts',(41.3913643974842,44.6323170406115,-1.55722280339885));
#40140=CARTESIAN_POINT('Ctrl Pts',(42.3109060773107,49.0823179301917,-1.75308536120414));
#40141=CARTESIAN_POINT('Ctrl Pts',(46.5265139156528,50.7783713513675,-1.94894791900943));
#40142=CARTESIAN_POINT('Ctrl Pts',(50.2717006433544,48.205140538033,-2.14481047681473));
#40143=CARTESIAN_POINT('Ctrl Pts',(50.2002873368139,43.661697764522,-2.34067303462002));
#40144=CARTESIAN_POINT('Ctrl Pts',(46.3760782190255,41.2074400215055,-2.53653559242531));
#40145=CARTESIAN_POINT('Ctrl Pts',(42.2158577781337,43.0351498520396,-2.73239815023061));
#40146=CARTESIAN_POINT('Ctrl Pts',(41.4366231225383,47.5118399189359,-2.9282607080359));
#40147=CARTESIAN_POINT('Ctrl Pts',(44.7345906088731,50.6377588369492,-3.1241232658412));
#40148=CARTESIAN_POINT('Ctrl Pts',(49.1631528076755,49.6200183172327,-3.31998582364649));
#40149=CARTESIAN_POINT('Ctrl Pts',(50.7655593735804,45.3679303091532,-3.51584838145178));
#40150=CARTESIAN_POINT('Ctrl Pts',(48.1101215244772,41.6805723363936,-3.71171093925708));
#40151=CARTESIAN_POINT('Ctrl Pts',(43.5693710758889,41.8524572016734,-3.90757349706237));
#40152=CARTESIAN_POINT('Ctrl Pts',(41.2002942889438,45.7300123917506,-4.10343605486766));
#40153=CARTESIAN_POINT('Ctrl Pts',(43.1195703563469,49.8487911453627,-4.29929861267296));
#40154=CARTESIAN_POINT('Ctrl Pts',(47.6123997659237,50.5288227185664,-4.49516117047825));
#40155=CARTESIAN_POINT('Ctrl Pts',(50.6646118667576,47.1625249946476,-4.69102372828354));
#40156=CARTESIAN_POINT('Ctrl Pts',(49.5491722744117,42.7575558053009,-4.88688628608884));
#40157=CARTESIAN_POINT('Ctrl Pts',(45.2626834729594,41.249586062651,-5.08274884389413));
#40158=CARTESIAN_POINT('Ctrl Pts',(41.6349586706169,43.9859288754904,-5.27861140169943));
#40159=CARTESIAN_POINT('Ctrl Pts',(41.9072308219428,48.5217669226154,-5.47447395950471));
#40160=CARTESIAN_POINT('Ctrl Pts',(45.8362350743765,50.8045030456205,-5.67033651731001));
#40161=CARTESIAN_POINT('Ctrl Pts',(49.9115571874415,48.7945999936567,-5.86619907511531));
#40162=CARTESIAN_POINT('Ctrl Pts',(50.4920526914155,44.2878292749147,-6.0620616329206));
#40163=CARTESIAN_POINT('Ctrl Pts',(47.059072278606,41.3108170258638,-6.2579241907259));
#40164=CARTESIAN_POINT('Ctrl Pts',(42.6798498547524,42.5234105517155,-6.45378674853118));
#40165=CARTESIAN_POINT('Ctrl Pts',(41.2670573850813,46.8422018041016,-6.64964930633648));
#40166=CARTESIAN_POINT('Ctrl Pts',(44.0829609284797,50.4085211796553,-6.84551186414177));
#40167=CARTESIAN_POINT('Ctrl Pts',(48.6116787512404,50.0359897044587,-7.04137442194707));
#40168=CARTESIAN_POINT('Ctrl Pts',(50.8069343717212,46.0574693241754,-7.23723697975236));
#40169=CARTESIAN_POINT('Ctrl Pts',(48.7074347435192,42.027575728146,-7.43309953755765));
#40170=CARTESIAN_POINT('Ctrl Pts',(44.1888313497151,41.5469450910147,-7.62896209536295));
#40171=CARTESIAN_POINT('Ctrl Pts',(41.2886721074914,45.0448370977533,-7.82482465316824));
#40172=CARTESIAN_POINT('Ctrl Pts',(42.5974243321682,49.3963573995622,-8.02068721097353));
#40173=CARTESIAN_POINT('Ctrl Pts',(46.9472267461691,50.7128989977065,-8.21654976877883));
#40174=CARTESIAN_POINT('Ctrl Pts',(50.4487163480431,47.8195940258066,-8.41241232658412));
#40175=CARTESIAN_POINT('Ctrl Pts',(49.9795579209025,43.2986184205048,-8.6082748843894));
#40176=CARTESIAN_POINT('Ctrl Pts',(45.9463561559116,41.1952276423334,-8.80413744219472));
#40177=CARTESIAN_POINT('Ctrl Pts',(43.3046954441484,42.6504167892078,-8.93471248073157));
#40178=CARTESIAN_POINT('Ctrl Pts',(42.5743852316216,43.7746037524369,-9.));
#40179=CARTESIAN_POINT('Ctrl Pts',(48.5732344270147,48.2065515280923,5.55111512312578E-16));
#40180=CARTESIAN_POINT('Ctrl Pts',(48.6498724529377,48.1336147846407,5.78603323158961E-16));
#40181=CARTESIAN_POINT('Ctrl Pts',(48.7225777107301,48.0570419129107,6.40347147519076E-16));
#40182=CARTESIAN_POINT('Ctrl Pts',(48.7913526914527,47.9772484866014,6.6266436782314E-16));
#40183=CARTESIAN_POINT('Ctrl Pts',(48.8618448358061,47.895462789728,6.85538801210275E-16));
#40184=CARTESIAN_POINT('Ctrl Pts',(48.928208390305,47.8102933006344,-6.7353910572983E-17));
#40185=CARTESIAN_POINT('Ctrl Pts',(48.9904198866102,47.7221391971955,2.77555756156289E-17));
#40186=CARTESIAN_POINT('Ctrl Pts',(49.0539468746188,47.6321210332761,1.24876197163927E-16));
#40187=CARTESIAN_POINT('Ctrl Pts',(49.1131448017078,47.5389901598639,1.68613647211554E-16));
#40188=CARTESIAN_POINT('Ctrl Pts',(49.1679552588207,47.4431291844734,5.55111512312578E-17));
#40189=CARTESIAN_POINT('Ctrl Pts',(49.2206161206072,47.3510277527091,-5.3155610957163E-17));
#40190=CARTESIAN_POINT('Ctrl Pts',(49.2692269857254,47.256405341668,1.53540688649506E-16));
#40191=CARTESIAN_POINT('Ctrl Pts',(49.3137022105639,47.1595731524251,1.66533453693773E-16));
#40192=CARTESIAN_POINT('Ctrl Pts',(49.3201152987639,47.1456104715737,1.68406940528153E-16));
#40193=CARTESIAN_POINT('Ctrl Pts',(49.326442337575,47.1316018071751,9.73571062393719E-16));
#40194=CARTESIAN_POINT('Ctrl Pts',(49.3326830075834,47.117548056573,9.85322934354826E-16));
#40195=CARTESIAN_POINT('Ctrl Pts',(49.3392332224637,47.1027972227374,9.97657713551053E-16));
#40196=CARTESIAN_POINT('Ctrl Pts',(49.3456847257789,47.088004706165,9.48337458744454E-16));
#40197=CARTESIAN_POINT('Ctrl Pts',(49.3520361876581,47.0731747255739,9.43689570931383E-16));
#40198=CARTESIAN_POINT('Ctrl Pts',(49.3968937084238,46.9684372375794,9.10863628170813E-16));
#40199=CARTESIAN_POINT('Ctrl Pts',(49.4367850985609,46.861787055252,3.49398990348419E-16));
#40200=CARTESIAN_POINT('Ctrl Pts',(49.4716812246059,46.7536536486796,4.44089209850063E-16));
#40201=CARTESIAN_POINT('Ctrl Pts',(49.5070988999261,46.6439041056987,5.40194647054708E-16));
#40202=CARTESIAN_POINT('Ctrl Pts',(49.5373713257785,46.5326259596867,6.64417056314631E-16));
#40203=CARTESIAN_POINT('Ctrl Pts',(49.5624283638924,46.4202317504508,6.93889390390723E-16));
#40204=CARTESIAN_POINT('Ctrl Pts',(49.5887049858113,46.3023670559666,7.2479621090423E-16));
#40205=CARTESIAN_POINT('Ctrl Pts',(49.6092470262998,46.1832742500753,7.37675641547393E-16));
#40206=CARTESIAN_POINT('Ctrl Pts',(49.6239198903984,46.0634004456029,8.88178419700125E-16));
#40207=CARTESIAN_POINT('Ctrl Pts',(49.6349245384724,45.9734950922486,1.00105550331467E-15));
#40208=CARTESIAN_POINT('Ctrl Pts',(49.642626697916,45.8831497171793,8.62982642107592E-16));
#40209=CARTESIAN_POINT('Ctrl Pts',(49.6469468769482,45.792547505348,8.88178419700125E-16));
#40210=CARTESIAN_POINT('Ctrl Pts',(49.647900301194,45.7725524206909,8.93738898807436E-16));
#40211=CARTESIAN_POINT('Ctrl Pts',(49.6486889090152,45.7525424656911,6.35931628352248E-16));
#40212=CARTESIAN_POINT('Ctrl Pts',(49.6493112460234,45.7325433534409,6.38378239159465E-16));
#40213=CARTESIAN_POINT('Ctrl Pts',(49.6529992119657,45.6140287160447,6.5287684234946E-16));
#40214=CARTESIAN_POINT('Ctrl Pts',(49.6508619840611,45.4957189678778,7.3986846148943E-16));
#40215=CARTESIAN_POINT('Ctrl Pts',(49.6428335563179,45.3780417000535,6.38378239159465E-16));
#40216=CARTESIAN_POINT('Ctrl Pts',(49.6348310508051,45.2607443892198,5.37215709001142E-16));
#40217=CARTESIAN_POINT('Ctrl Pts',(49.6209756516749,45.1440745969525,1.03714765940918E-15));
#40218=CARTESIAN_POINT('Ctrl Pts',(49.6011537548333,45.0284382457395,1.19348975147204E-15));
#40219=CARTESIAN_POINT('Ctrl Pts',(49.5986006508385,45.0135440288755,1.21362695746072E-15));
#40220=CARTESIAN_POINT('Ctrl Pts',(49.5959484928759,44.9986669435562,6.39393560469819E-16));
#40221=CARTESIAN_POINT('Ctrl Pts',(49.5931969753943,44.9838078477401,6.38378239159465E-16));
#40222=CARTESIAN_POINT('Ctrl Pts',(49.5723040282194,44.8709790883241,6.02913079779512E-16));
#40223=CARTESIAN_POINT('Ctrl Pts',(49.5456866559789,44.7591873160563,3.64931038818624E-16));
#40224=CARTESIAN_POINT('Ctrl Pts',(49.5136431171323,44.6486943685595,2.77555756156289E-16));
#40225=CARTESIAN_POINT('Ctrl Pts',(49.4934334709872,44.5790072038202,2.22448748379061E-16));
#40226=CARTESIAN_POINT('Ctrl Pts',(49.4710643432933,44.5098366898445,2.79582804221843E-16));
#40227=CARTESIAN_POINT('Ctrl Pts',(49.4466001824985,44.4412500442809,2.22044604925031E-16));
#40228=CARTESIAN_POINT('Ctrl Pts',(49.437958075777,44.4170214138529,2.0171890223469E-16));
#40229=CARTESIAN_POINT('Ctrl Pts',(49.4290544610887,44.3928656610227,1.16258512332692E-15));
#40230=CARTESIAN_POINT('Ctrl Pts',(49.4198919565046,44.3687858124111,1.16573417585641E-15));
#40231=CARTESIAN_POINT('Ctrl Pts',(49.4140177808709,44.3533479745711,1.1677530657209E-15));
#40232=CARTESIAN_POINT('Ctrl Pts',(49.4080385614616,44.3379450507796,4.6560458043002E-16));
#40233=CARTESIAN_POINT('Ctrl Pts',(49.4019587711633,44.3225866875802,4.71844785465692E-16));
#40234=CARTESIAN_POINT('Ctrl Pts',(49.3590836254494,44.2142783368314,5.15851188164403E-16));
#40235=CARTESIAN_POINT('Ctrl Pts',(49.3111615328034,44.1080549532259,2.48937019875304E-16));
#40236=CARTESIAN_POINT('Ctrl Pts',(49.2585466556507,44.0041726189596,3.33066907387547E-16));
#40237=CARTESIAN_POINT('Ctrl Pts',(49.2040876136808,43.8966491824735,4.20145568840418E-16));
#40238=CARTESIAN_POINT('Ctrl Pts',(49.1446009389686,43.7916331003358,8.50083000759442E-16));
#40239=CARTESIAN_POINT('Ctrl Pts',(49.0804234387592,43.6894117471813,8.32667268468867E-16));
#40240=CARTESIAN_POINT('Ctrl Pts',(49.0155503679019,43.5860824952676,8.1506278042816E-16));
#40241=CARTESIAN_POINT('Ctrl Pts',(48.9458838603176,43.4856081197834,5.53746625258472E-16));
#40242=CARTESIAN_POINT('Ctrl Pts',(48.871719760908,43.3882998852588,6.10622663543836E-16));
#40243=CARTESIAN_POINT('Ctrl Pts',(48.8190210220156,43.3191556323909,6.51037035385447E-16));
#40244=CARTESIAN_POINT('Ctrl Pts',(48.764050303434,43.251610267159,-1.27380500588882E-16));
#40245=CARTESIAN_POINT('Ctrl Pts',(48.7068997131453,43.1857830872598,-1.11022302462516E-16));
#40246=CARTESIAN_POINT('Ctrl Pts',(48.6896338669553,43.1658959442308,-1.060803039395E-16));
#40247=CARTESIAN_POINT('Ctrl Pts',(48.6721689865425,43.1461656757307,8.76550187881266E-16));
#40248=CARTESIAN_POINT('Ctrl Pts',(48.6545074240829,43.1265957195894,8.88178419700125E-16));
#40249=CARTESIAN_POINT('Ctrl Pts',(48.6371228895828,43.1073327252489,8.99624258520571E-16));
#40250=CARTESIAN_POINT('Ctrl Pts',(48.6195440978478,43.0882212546125,1.08275417850399E-15));
#40251=CARTESIAN_POINT('Ctrl Pts',(48.6017950003255,43.0692874663464,1.0547118733939E-15));
#40252=CARTESIAN_POINT('Ctrl Pts',(48.5161349724081,42.977909928451,9.19375153564364E-16));
#40253=CARTESIAN_POINT('Ctrl Pts',(48.4264330472783,42.8905783040618,1.12985113368144E-15));
#40254=CARTESIAN_POINT('Ctrl Pts',(48.3330185610229,42.8076088281368,8.88178419700125E-16));
#40255=CARTESIAN_POINT('Ctrl Pts',(48.2522205241438,42.7358451109195,6.79145734945449E-16));
#40256=CARTESIAN_POINT('Ctrl Pts',(48.1686440240513,42.6673447664859,6.67861884923022E-16));
#40257=CARTESIAN_POINT('Ctrl Pts',(48.0824754659943,42.6023283204542,7.7715611723761E-16));
#40258=CARTESIAN_POINT('Ctrl Pts',(48.0430744722317,42.5725992331592,8.27131438431595E-16));
#40259=CARTESIAN_POINT('Ctrl Pts',(48.003131210002,42.5435988074275,1.18894675673887E-15));
#40260=CARTESIAN_POINT('Ctrl Pts',(47.9626620077452,42.5153495000384,1.16573417585641E-15));
#40261=CARTESIAN_POINT('Ctrl Pts',(47.9441427039662,42.5024222003658,1.15511175651322E-15));
#40262=CARTESIAN_POINT('Ctrl Pts',(47.9255113044799,42.4896509007091,3.58310774532543E-16));
#40263=CARTESIAN_POINT('Ctrl Pts',(47.9067756067456,42.4770420458757,3.33066907387547E-16));
#40264=CARTESIAN_POINT('Ctrl Pts',(47.8018201929055,42.4064085634267,1.9165341103939E-16));
#40265=CARTESIAN_POINT('Ctrl Pts',(47.6937577709793,42.3409782246222,1.69127847991709E-16));
#40266=CARTESIAN_POINT('Ctrl Pts',(47.5828994070635,42.2810832344563,1.11022302462516E-16));
#40267=CARTESIAN_POINT('Ctrl Pts',(47.4730677670903,42.2217429667153,5.34549062680856E-17));
#40268=CARTESIAN_POINT('Ctrl Pts',(47.3604911538792,42.1678352915987,7.49804862520293E-17));
#40269=CARTESIAN_POINT('Ctrl Pts',(47.2454366428579,42.1197191971386,1.66533453693773E-16));
#40270=CARTESIAN_POINT('Ctrl Pts',(47.1845208924579,42.0942440725709,2.69415779354553E-16));
#40271=CARTESIAN_POINT('Ctrl Pts',(47.1229099962542,42.0703931037216,1.36788762772911E-16));
#40272=CARTESIAN_POINT('Ctrl Pts',(47.0606640384105,42.0481501283249,1.66533453693773E-16));
#40273=CARTESIAN_POINT('Ctrl Pts',(42.612019924001,45.9972524552388,-2.01601780324957));
#40274=CARTESIAN_POINT('Ctrl Pts',(42.6094250933538,45.6709119514131,-1.99688706151736));
#40275=CARTESIAN_POINT('Ctrl Pts',(42.6528677689476,45.3452478112547,-1.97775631978515));
#40276=CARTESIAN_POINT('Ctrl Pts',(42.7452066790694,45.0340947481843,-1.95862557805294));
#40277=CARTESIAN_POINT('Ctrl Pts',(43.0603318560328,43.9722220887233,-1.8933380587845));
#40278=CARTESIAN_POINT('Ctrl Pts',(43.9449287141776,43.079353188851,-1.82805053951607));
#40279=CARTESIAN_POINT('Ctrl Pts',(45.0038225737112,42.7543474598092,-1.76276302024764));
#40280=CARTESIAN_POINT('Ctrl Pts',(46.0627164332447,42.4293417307674,-1.69747550097921));
#40281=CARTESIAN_POINT('Ctrl Pts',(47.295907294167,42.6721991725562,-1.63218798171078));
#40282=CARTESIAN_POINT('Ctrl Pts',(48.1524867306922,43.3744537095404,-1.56690046244235));
#40283=CARTESIAN_POINT('Ctrl Pts',(49.0090661672174,44.0767082465247,-1.50161294317392));
#40284=CARTESIAN_POINT('Ctrl Pts',(49.4890341793456,45.2383598787045,-1.43632542390549));
#40285=CARTESIAN_POINT('Ctrl Pts',(49.3779825894782,46.3404102475651,-1.37103790463705));
#40286=CARTESIAN_POINT('Ctrl Pts',(49.2669309996107,47.4424606164257,-1.30575038536862));
#40287=CARTESIAN_POINT('Ctrl Pts',(48.5648598077476,48.4849097219671,-1.24046286610019));
#40288=CARTESIAN_POINT('Ctrl Pts',(47.5853888393785,49.0021713029189,-1.17517534683176));
#40289=CARTESIAN_POINT('Ctrl Pts',(46.6059178710094,49.5194328838706,-1.10988782756333));
#40290=CARTESIAN_POINT('Ctrl Pts',(45.3490471261342,49.5115069402328,-1.0446003082949));
#40291=CARTESIAN_POINT('Ctrl Pts',(44.3762942478984,48.981713762666,-0.979312789026468));
#40292=CARTESIAN_POINT('Ctrl Pts',(43.4035413696625,48.4519205850993,-0.914025269758036));
#40293=CARTESIAN_POINT('Ctrl Pts',(42.714906358066,47.4002601736038,-0.848737750489605));
#40294=CARTESIAN_POINT('Ctrl Pts',(42.6179526637934,46.2969922908292,-0.783450231221173));
#40295=CARTESIAN_POINT('Ctrl Pts',(42.6093234581355,46.198797729728,-0.777639421897304));
#40296=CARTESIAN_POINT('Ctrl Pts',(42.60538131527,46.1001943548762,-0.771828612573434));
#40297=CARTESIAN_POINT('Ctrl Pts',(42.6059705137377,46.0015452631454,-0.766017803249565));
#40298=CARTESIAN_POINT('Ctrl Pts',(44.942095577027,42.0543614925016,0.));
#40299=CARTESIAN_POINT('Ctrl Pts',(43.6472519732775,42.4015349025496,-0.0652875192684312));
#40300=CARTESIAN_POINT('Ctrl Pts',(41.4469681313217,44.4642342884812,-0.195862557805293));
#40301=CARTESIAN_POINT('Ctrl Pts',(42.2010812738077,48.9500090171859,-0.391725115610587));
#40302=CARTESIAN_POINT('Ctrl Pts',(46.3558078761971,50.7932688919524,-0.58758767341588));
#40303=CARTESIAN_POINT('Ctrl Pts',(50.1895250164382,48.3572314578353,-0.783450231221173));
#40304=CARTESIAN_POINT('Ctrl Pts',(50.281582214734,43.813490556254,-0.979312789026467));
#40305=CARTESIAN_POINT('Ctrl Pts',(46.5474666641534,41.224098161527,-1.17517534683176));
#40306=CARTESIAN_POINT('Ctrl Pts',(42.3245742788969,42.9014062059293,-1.37103790463705));
#40307=CARTESIAN_POINT('Ctrl Pts',(41.3853558532093,47.3473770059323,-1.56690046244235));
#40308=CARTESIAN_POINT('Ctrl Pts',(44.5692318828111,50.5894261400569,-1.76276302024764));
#40309=CARTESIAN_POINT('Ctrl Pts',(49.0314017551548,49.7310441604199,-1.95862557805294));
#40310=CARTESIAN_POINT('Ctrl Pts',(50.7851513154972,45.5390953919881,-2.15448813585823));
#40311=CARTESIAN_POINT('Ctrl Pts',(48.2635416323089,41.7589579733313,-2.35035069366352));
#40312=CARTESIAN_POINT('Ctrl Pts',(43.7195493508676,41.7680235772757,-2.54621325146881));
#40313=CARTESIAN_POINT('Ctrl Pts',(41.2130497701183,45.558200280547,-2.74207580927411));
#40314=CARTESIAN_POINT('Ctrl Pts',(42.9835077018007,49.7431068173874,-2.9379383670794));
#40315=CARTESIAN_POINT('Ctrl Pts',(47.4490851541316,50.5836916797423,-3.1338009248847));
#40316=CARTESIAN_POINT('Ctrl Pts',(50.619960918391,47.3289236340817,-3.32966348268999));
#40317=CARTESIAN_POINT('Ctrl Pts',(49.6630787639445,42.8868134693702,-3.52552604049528));
#40318=CARTESIAN_POINT('Ctrl Pts',(45.4333763810852,41.2262159220479,-3.72138859830058));
#40319=CARTESIAN_POINT('Ctrl Pts',(41.7099304228444,43.8308112789577,-3.91725115610586));
#40320=CARTESIAN_POINT('Ctrl Pts',(41.8194970071128,48.3734934933536,-4.11311371391117));
#40321=CARTESIAN_POINT('Ctrl Pts',(45.664182571157,50.7955503680233,-4.30897627171645));
#40322=CARTESIAN_POINT('Ctrl Pts',(49.8089081243513,48.9329670248342,-4.50483882952175));
#40323=CARTESIAN_POINT('Ctrl Pts',(50.5505204413009,44.4498902060922,-4.70070138732704));
#40324=CARTESIAN_POINT('Ctrl Pts',(47.226417382704,41.351776998474,-4.89656394513234));
#40325=CARTESIAN_POINT('Ctrl Pts',(42.8065574559861,42.4066726567364,-5.09242650293762));
#40326=CARTESIAN_POINT('Ctrl Pts',(41.2399158926326,46.6720683948219,-5.28828906074293));
#40327=CARTESIAN_POINT('Ctrl Pts',(43.926226788663,50.3369968125737,-5.48415161854822));
#40328=CARTESIAN_POINT('Ctrl Pts',(48.4653744868355,50.126985023971,-5.68001417635351));
#40329=CARTESIAN_POINT('Ctrl Pts',(50.8018046472976,46.229670491242,-5.87587673415881));
#40330=CARTESIAN_POINT('Ctrl Pts',(48.8480067336088,42.1271542042059,-6.07173929196409));
#40331=CARTESIAN_POINT('Ctrl Pts',(44.3496239015183,41.4848769748296,-6.26760184976939));
#40332=CARTESIAN_POINT('Ctrl Pts',(41.3257891865932,44.8766889552318,-6.46346440757468));
#40333=CARTESIAN_POINT('Ctrl Pts',(42.4781816117647,49.2721361120468,-6.65932696537998));
#40334=CARTESIAN_POINT('Ctrl Pts',(46.7771853228611,50.7440554992066,-6.85518952318527));
#40335=CARTESIAN_POINT('Ctrl Pts',(50.3818002707934,47.9773428079219,-7.05105208099057));
#40336=CARTESIAN_POINT('Ctrl Pts',(50.0714520002853,43.4439513347231,-7.24691463879585));
#40337=CARTESIAN_POINT('Ctrl Pts',(46.1234029772789,41.1942889357184,-7.44277719660116));
#40338=CARTESIAN_POINT('Ctrl Pts',(42.0651280613364,43.2383496733801,-7.63863975440644));
#40339=CARTESIAN_POINT('Ctrl Pts',(41.5224490242513,47.7498293223045,-7.83450231221174));
#40340=CARTESIAN_POINT('Ctrl Pts',(44.9804150360981,50.6979233958617,-8.03036487001703));
#40341=CARTESIAN_POINT('Ctrl Pts',(49.3490853663058,49.448562791698,-8.22622742782233));
#40342=CARTESIAN_POINT('Ctrl Pts',(50.7259992165293,45.1181263046889,-8.42208998562762));
#40343=CARTESIAN_POINT('Ctrl Pts',(47.8793454040792,41.5754411676036,-8.61795254343291));
#40344=CARTESIAN_POINT('Ctrl Pts',(43.3557537989775,41.986275053806,-8.81381510123821));
#40345=CARTESIAN_POINT('Ctrl Pts',(41.190215141007,45.9824985745015,-9.0096776590435));
#40346=CARTESIAN_POINT('Ctrl Pts',(43.3312719327635,49.99581856708,-9.2055402168488));
#40347=CARTESIAN_POINT('Ctrl Pts',(46.3331931919405,50.2864153592086,-9.33611525538566));
#40348=CARTESIAN_POINT('Ctrl Pts',(47.5707104172798,49.7709539622022,-9.40140277465409));
#40349=CARTESIAN_POINT('Ctrl Pts',(45.0021125537771,42.2782052438144,0.133800924884696));
#40350=CARTESIAN_POINT('Ctrl Pts',(43.780727947621,42.6056828306607,0.0685134056162645));
#40351=CARTESIAN_POINT('Ctrl Pts',(41.7052704900895,44.5513612661175,-0.0620616329205976));
#40352=CARTESIAN_POINT('Ctrl Pts',(42.4166013263891,48.7826492644973,-0.257924190725891));
#40353=CARTESIAN_POINT('Ctrl Pts',(46.3356222029269,50.5213374193184,-0.453786748531185));
#40354=CARTESIAN_POINT('Ctrl Pts',(49.9518451088349,48.2235011297195,-0.649649306336477));
#40355=CARTESIAN_POINT('Ctrl Pts',(50.0386797231148,43.9375354922609,-0.845511864141771));
#40356=CARTESIAN_POINT('Ctrl Pts',(46.5164078148468,41.4950443674184,-1.04137442194706));
#40357=CARTESIAN_POINT('Ctrl Pts',(42.5330883329644,43.0771954621779,-1.23723697975236));
#40358=CARTESIAN_POINT('Ctrl Pts',(41.6471535964207,47.2709376861956,-1.43309953755765));
#40359=CARTESIAN_POINT('Ctrl Pts',(44.6504021425806,50.3290590634453,-1.62896209536294));
#40360=CARTESIAN_POINT('Ctrl Pts',(48.8594244340393,49.5193747640485,-1.82482465316824));
#40361=CARTESIAN_POINT('Ctrl Pts',(50.5136803687734,45.5652434073875,-2.02068721097353));
#40362=CARTESIAN_POINT('Ctrl Pts',(48.1351265103291,41.9995605411846,-2.21654976877883));
#40363=CARTESIAN_POINT('Ctrl Pts',(43.8489237542792,42.0081118357741,-2.41241232658412));
#40364=CARTESIAN_POINT('Ctrl Pts',(41.484622772756,45.5832644384377,-2.60827488438941));
#40365=CARTESIAN_POINT('Ctrl Pts',(43.1546391804072,49.5307530830105,-2.80413744219471));
#40366=CARTESIAN_POINT('Ctrl Pts',(47.3668757332087,50.3236499302245,-3.));
#40367=CARTESIAN_POINT('Ctrl Pts',(50.3578615443795,47.2535312100429,-3.19586255780529));
#40368=CARTESIAN_POINT('Ctrl Pts',(49.4552651767856,43.0634305999634,-3.39172511561059));
#40369=CARTESIAN_POINT('Ctrl Pts',(45.4655220417176,41.4970419832635,-3.58758767341588));
#40370=CARTESIAN_POINT('Ctrl Pts',(41.9533144190514,43.953873576657,-3.78345023122117));
#40371=CARTESIAN_POINT('Ctrl Pts',(42.0566650777619,48.2388405883145,-3.97931278902647));
#40372=CARTESIAN_POINT('Ctrl Pts',(45.6832341474444,50.5234894628117,-4.17517534683176));
#40373=CARTESIAN_POINT('Ctrl Pts',(49.5928213537715,48.7665740975379,-4.37103790463706));
#40374=CARTESIAN_POINT('Ctrl Pts',(50.292360560696,44.5378309514381,-4.56690046244235));
#40375=CARTESIAN_POINT('Ctrl Pts',(47.1568403377979,41.615479735464,-4.76276302024764));
#40376=CARTESIAN_POINT('Ctrl Pts',(42.9877276664084,42.6105291100537,-4.95862557805293));
#40377=CARTESIAN_POINT('Ctrl Pts',(41.5099647278547,46.6339406468415,-5.15448813585822));
#40378=CARTESIAN_POINT('Ctrl Pts',(44.0438759788044,50.0909505429741,-5.35035069366352));
#40379=CARTESIAN_POINT('Ctrl Pts',(48.3255089942224,49.8928531318523,-5.54621325146881));
#40380=CARTESIAN_POINT('Ctrl Pts',(50.529388924651,46.2166408373019,-5.74207580927411));
#40381=CARTESIAN_POINT('Ctrl Pts',(48.6864337689787,42.3468682833185,-5.9379383670794));
#40382=CARTESIAN_POINT('Ctrl Pts',(44.4432529494554,41.7410286911291,-6.13380092488469));
#40383=CARTESIAN_POINT('Ctrl Pts',(41.5909662627271,44.940416576927,-6.32966348268999));
#40384=CARTESIAN_POINT('Ctrl Pts',(42.6779812228965,49.0865014623609,-6.52552604049528));
#40385=CARTESIAN_POINT('Ctrl Pts',(46.7330940869803,50.4749159981194,-6.72138859830058));
#40386=CARTESIAN_POINT('Ctrl Pts',(50.1332122138151,47.8651643022338,-6.91725115610587));
#40387=CARTESIAN_POINT('Ctrl Pts',(49.8404706046755,43.5889609499442,-7.11311371391116));
#40388=CARTESIAN_POINT('Ctrl Pts',(46.1164020862178,41.4669262770029,-7.30897627171645));
#40389=CARTESIAN_POINT('Ctrl Pts',(42.2883610042459,43.3950234709796,-7.50483882952175));
#40390=CARTESIAN_POINT('Ctrl Pts',(41.7764692050663,47.6505580994295,-7.70070138732704));
#40391=CARTESIAN_POINT('Ctrl Pts',(45.03825807536,50.4314010587771,-7.89656394513233));
#40392=CARTESIAN_POINT('Ctrl Pts',(49.1590852356714,49.2529191131237,-8.09242650293763));
#40393=CARTESIAN_POINT('Ctrl Pts',(50.4578840834986,45.1681567156775,-8.28828906074292));
#40394=CARTESIAN_POINT('Ctrl Pts',(47.7727264818281,41.8264550009959,-8.48415161854822));
#40395=CARTESIAN_POINT('Ctrl Pts',(43.5057670320466,42.213981481292,-8.6800141763535));
#40396=CARTESIAN_POINT('Ctrl Pts',(41.4630835965936,45.9834914644304,-8.8758767341588));
#40397=CARTESIAN_POINT('Ctrl Pts',(43.4826740697482,49.7691280033295,-9.0717392919641));
#40398=CARTESIAN_POINT('Ctrl Pts',(46.3142904937197,50.0432386738974,-9.20231433050096));
#40399=CARTESIAN_POINT('Ctrl Pts',(47.4816009584782,49.5570204051054,-9.26760184976939));
#40400=CARTESIAN_POINT('Ctrl Pts',(45.0621295305271,42.5020489951272,0.267601849769391));
#40401=CARTESIAN_POINT('Ctrl Pts',(43.9142039219644,42.8098307587719,0.20231433050096));
#40402=CARTESIAN_POINT('Ctrl Pts',(41.9635728488572,44.6384882437539,0.0717392919640979));
#40403=CARTESIAN_POINT('Ctrl Pts',(42.6321213789705,48.6152895118088,-0.124123265841195));
#40404=CARTESIAN_POINT('Ctrl Pts',(46.3154365296567,50.2494059466843,-0.319985823646489));
#40405=CARTESIAN_POINT('Ctrl Pts',(49.7141652012317,48.0897708016036,-0.515848381451782));
#40406=CARTESIAN_POINT('Ctrl Pts',(49.7957772314955,44.0615804282678,-0.711710939257076));
#40407=CARTESIAN_POINT('Ctrl Pts',(46.4853489655401,41.7659905733098,-0.90757349706237));
#40408=CARTESIAN_POINT('Ctrl Pts',(42.7416023870319,43.2529847184266,-1.10343605486766));
#40409=CARTESIAN_POINT('Ctrl Pts',(41.9089513396321,47.1944983664588,-1.29929861267296));
#40410=CARTESIAN_POINT('Ctrl Pts',(44.7315724023501,50.0686919868338,-1.49516117047825));
#40411=CARTESIAN_POINT('Ctrl Pts',(48.6874471129237,49.307705367677,-1.69102372828354));
#40412=CARTESIAN_POINT('Ctrl Pts',(50.2422094220497,45.591391422787,-1.88688628608883));
#40413=CARTESIAN_POINT('Ctrl Pts',(48.0067113883493,42.2401631090378,-2.08274884389413));
#40414=CARTESIAN_POINT('Ctrl Pts',(43.9782981576908,42.2482000942726,-2.27861140169942));
#40415=CARTESIAN_POINT('Ctrl Pts',(41.7561957753938,45.6083285963283,-2.47447395950472));
#40416=CARTESIAN_POINT('Ctrl Pts',(43.3257706590138,49.3183993486336,-2.67033651731001));
#40417=CARTESIAN_POINT('Ctrl Pts',(47.2846663122857,50.0636081807067,-2.86619907511531));
#40418=CARTESIAN_POINT('Ctrl Pts',(50.095762170368,47.1781387860041,-3.0620616329206));
#40419=CARTESIAN_POINT('Ctrl Pts',(49.2474515896267,43.2400477305567,-3.25792419072589));
#40420=CARTESIAN_POINT('Ctrl Pts',(45.4976677023501,41.7678680444789,-3.45378674853118));
#40421=CARTESIAN_POINT('Ctrl Pts',(42.1966984152584,44.0769358743563,-3.64964930633648));
#40422=CARTESIAN_POINT('Ctrl Pts',(42.2938331484111,48.1041876832753,-3.84551186414177));
#40423=CARTESIAN_POINT('Ctrl Pts',(45.702285723732,50.2514285576001,-4.04137442194706));
#40424=CARTESIAN_POINT('Ctrl Pts',(49.3767345831917,48.6001811702416,-4.23723697975236));
#40425=CARTESIAN_POINT('Ctrl Pts',(50.034200680091,44.6257716967841,-4.43309953755765));
#40426=CARTESIAN_POINT('Ctrl Pts',(47.0872632928917,41.8791824724537,-4.62896209536295));
#40427=CARTESIAN_POINT('Ctrl Pts',(43.1688978768307,42.8143855633711,-4.82482465316823));
#40428=CARTESIAN_POINT('Ctrl Pts',(41.7800135630769,46.595812898861,-5.02068721097354));
#40429=CARTESIAN_POINT('Ctrl Pts',(44.1615251689457,49.8449042733747,-5.21654976877882));
#40430=CARTESIAN_POINT('Ctrl Pts',(48.1856435016095,49.6587212397334,-5.41241232658412));
#40431=CARTESIAN_POINT('Ctrl Pts',(50.2569732020045,46.2036111833619,-5.60827488438941));
#40432=CARTESIAN_POINT('Ctrl Pts',(48.5248608043486,42.5665823624312,-5.80413744219471));
#40433=CARTESIAN_POINT('Ctrl Pts',(44.5368819973926,41.9971804074285,-6.));
#40434=CARTESIAN_POINT('Ctrl Pts',(41.8561433388609,45.0041441986222,-6.19586255780529));
#40435=CARTESIAN_POINT('Ctrl Pts',(42.8777808340284,48.900866812675,-6.39172511561059));
#40436=CARTESIAN_POINT('Ctrl Pts',(46.6890028510995,50.2057764970322,-6.58758767341588));
#40437=CARTESIAN_POINT('Ctrl Pts',(49.8846241568369,47.7529857965456,-6.78345023122117));
#40438=CARTESIAN_POINT('Ctrl Pts',(49.6094892090656,43.7339705651652,-6.97931278902646));
#40439=CARTESIAN_POINT('Ctrl Pts',(46.1094011951568,41.7395636182874,-7.17517534683176));
#40440=CARTESIAN_POINT('Ctrl Pts',(42.5115939471553,43.5516972685792,-7.37103790463705));
#40441=CARTESIAN_POINT('Ctrl Pts',(42.0304893858815,47.5512868765546,-7.56690046244235));
#40442=CARTESIAN_POINT('Ctrl Pts',(45.0961011146216,50.1648787216924,-7.76276302024763));
#40443=CARTESIAN_POINT('Ctrl Pts',(48.9690851050371,49.0572754345494,-7.95862557805294));
#40444=CARTESIAN_POINT('Ctrl Pts',(50.1897689504678,45.218187126666,-8.15448813585822));
#40445=CARTESIAN_POINT('Ctrl Pts',(47.6661075595772,42.0774688343883,-8.35035069366352));
#40446=CARTESIAN_POINT('Ctrl Pts',(43.6557802651156,42.441687908778,-8.54621325146882));
#40447=CARTESIAN_POINT('Ctrl Pts',(41.7359520521803,45.9844843543592,-8.74207580927411));
#40448=CARTESIAN_POINT('Ctrl Pts',(43.6340762067327,49.542437439579,-8.9379383670794));
#40449=CARTESIAN_POINT('Ctrl Pts',(46.2953877954988,49.8000619885861,-9.06851340561627));
#40450=CARTESIAN_POINT('Ctrl Pts',(47.3924914996766,49.3430868480086,-9.1338009248847));
#40451=CARTESIAN_POINT('Ctrl Pts',(45.1221465072772,42.72589274644,0.401402774654087));
#40452=CARTESIAN_POINT('Ctrl Pts',(44.0476798963078,43.0139786868831,0.336115255385656));
#40453=CARTESIAN_POINT('Ctrl Pts',(42.221875207625,44.7256152213902,0.205540216848794));
#40454=CARTESIAN_POINT('Ctrl Pts',(42.8476414315519,48.4479297591202,0.00967765904350007));
#40455=CARTESIAN_POINT('Ctrl Pts',(46.2952508563866,49.9774744740503,-0.186184898761793));
#40456=CARTESIAN_POINT('Ctrl Pts',(49.4764852936283,47.9560404734877,-0.382047456567087));
#40457=CARTESIAN_POINT('Ctrl Pts',(49.5528747398763,44.1856253642746,-0.57791001437238));
#40458=CARTESIAN_POINT('Ctrl Pts',(46.4542901162335,42.0369367792011,-0.773772572177674));
#40459=CARTESIAN_POINT('Ctrl Pts',(42.9501164410994,43.4287739746753,-0.969635129982967));
#40460=CARTESIAN_POINT('Ctrl Pts',(42.1707490828436,47.118059046722,-1.16549768778826));
#40461=CARTESIAN_POINT('Ctrl Pts',(44.8127426621197,49.8083249102222,-1.36136024559355));
#40462=CARTESIAN_POINT('Ctrl Pts',(48.5154697918081,49.0960359713057,-1.55722280339885));
#40463=CARTESIAN_POINT('Ctrl Pts',(49.970738475326,45.6175394381864,-1.75308536120414));
#40464=CARTESIAN_POINT('Ctrl Pts',(47.8782962663694,42.4807656768911,-1.94894791900943));
#40465=CARTESIAN_POINT('Ctrl Pts',(44.1076725611025,42.4882883527711,-2.14481047681473));
#40466=CARTESIAN_POINT('Ctrl Pts',(42.0277687780314,45.6333927542189,-2.34067303462002));
#40467=CARTESIAN_POINT('Ctrl Pts',(43.4969021376203,49.1060456142567,-2.53653559242531));
#40468=CARTESIAN_POINT('Ctrl Pts',(47.2024568913628,49.8035664311889,-2.73239815023061));
#40469=CARTESIAN_POINT('Ctrl Pts',(49.8336627963565,47.1027463619653,-2.9282607080359));
#40470=CARTESIAN_POINT('Ctrl Pts',(49.0396380024677,43.4166648611499,-3.12412326584119));
#40471=CARTESIAN_POINT('Ctrl Pts',(45.5298133629825,42.0386941056945,-3.31998582364649));
#40472=CARTESIAN_POINT('Ctrl Pts',(42.4400824114655,44.1999981720555,-3.51584838145178));
#40473=CARTESIAN_POINT('Ctrl Pts',(42.5310012190602,47.9695347782363,-3.71171093925708));
#40474=CARTESIAN_POINT('Ctrl Pts',(45.7213373000194,49.9793676523885,-3.90757349706237));
#40475=CARTESIAN_POINT('Ctrl Pts',(49.1606478126119,48.4337882429453,-4.10343605486766));
#40476=CARTESIAN_POINT('Ctrl Pts',(49.776040799486,44.7137124421301,-4.29929861267295));
#40477=CARTESIAN_POINT('Ctrl Pts',(47.0176862479855,42.1428852094436,-4.49516117047825));
#40478=CARTESIAN_POINT('Ctrl Pts',(43.3500680872531,43.0182420166884,-4.69102372828354));
#40479=CARTESIAN_POINT('Ctrl Pts',(42.0500623982989,46.5576851508807,-4.88688628608884));
#40480=CARTESIAN_POINT('Ctrl Pts',(44.279174359087,49.5988580037752,-5.08274884389412));
#40481=CARTESIAN_POINT('Ctrl Pts',(48.0457780089964,49.4245893476147,-5.27861140169943));
#40482=CARTESIAN_POINT('Ctrl Pts',(49.9845574793579,46.1905815294217,-5.47447395950471));
#40483=CARTESIAN_POINT('Ctrl Pts',(48.3632878397186,42.7862964415439,-5.67033651731002));
#40484=CARTESIAN_POINT('Ctrl Pts',(44.6305110453297,42.2533321237279,-5.8661990751153));
#40485=CARTESIAN_POINT('Ctrl Pts',(42.1213204149949,45.0678718203174,-6.06206163292059));
#40486=CARTESIAN_POINT('Ctrl Pts',(43.0775804451602,48.7152321629891,-6.25792419072589));
#40487=CARTESIAN_POINT('Ctrl Pts',(46.6449116152187,49.936636995945,-6.45378674853118));
#40488=CARTESIAN_POINT('Ctrl Pts',(49.6360360998585,47.6408072908576,-6.64964930633648));
#40489=CARTESIAN_POINT('Ctrl Pts',(49.3785078134558,43.8789801803862,-6.84551186414177));
#40490=CARTESIAN_POINT('Ctrl Pts',(46.1024003040958,42.012200959572,-7.04137442194707));
#40491=CARTESIAN_POINT('Ctrl Pts',(42.7348268900648,43.7083710661787,-7.23723697975235));
#40492=CARTESIAN_POINT('Ctrl Pts',(42.2845095666966,47.4520156536797,-7.43309953755766));
#40493=CARTESIAN_POINT('Ctrl Pts',(45.1539441538833,49.8983563846077,-7.62896209536294));
#40494=CARTESIAN_POINT('Ctrl Pts',(48.7790849744028,48.8616317559751,-7.82482465316824));
#40495=CARTESIAN_POINT('Ctrl Pts',(49.921653817437,45.2682175376546,-8.02068721097353));
#40496=CARTESIAN_POINT('Ctrl Pts',(47.5594886373262,42.3284826677807,-8.21654976877883));
#40497=CARTESIAN_POINT('Ctrl Pts',(43.8057934981846,42.6693943362641,-8.41241232658412));
#40498=CARTESIAN_POINT('Ctrl Pts',(42.008820507767,45.985477244288,-8.60827488438941));
#40499=CARTESIAN_POINT('Ctrl Pts',(43.7854783437173,49.3157468758285,-8.80413744219471));
#40500=CARTESIAN_POINT('Ctrl Pts',(46.276485097278,49.5568853032748,-8.93471248073157));
#40501=CARTESIAN_POINT('Ctrl Pts',(47.303382040875,49.1291532909119,-9.));
#40502=CARTESIAN_POINT('Ctrl Pts',(42.6118894404877,46.0027670997301,-1.10898219675043));
#40503=CARTESIAN_POINT('Ctrl Pts',(42.6093009894316,46.3240935072758,-1.12782069376304));
#40504=CARTESIAN_POINT('Ctrl Pts',(42.6514001366817,46.6447561369006,-1.14665919077565));
#40505=CARTESIAN_POINT('Ctrl Pts',(42.7409759057656,46.9515558452975,-1.16549768778826));
#40506=CARTESIAN_POINT('Ctrl Pts',(43.0514136092689,48.0148143345554,-1.23078520705669));
#40507=CARTESIAN_POINT('Ctrl Pts',(43.9320781356943,48.9115696223888,-1.29607272632512));
#40508=CARTESIAN_POINT('Ctrl Pts',(44.9895315871884,49.2412324431528,-1.36136024559355));
#40509=CARTESIAN_POINT('Ctrl Pts',(46.0469850386825,49.5708952639167,-1.42664776486199));
#40510=CARTESIAN_POINT('Ctrl Pts',(47.2812274152453,49.3334656176112,-1.49193528413042));
#40511=CARTESIAN_POINT('Ctrl Pts',(48.140893384113,48.6350013722719,-1.55722280339885));
#40512=CARTESIAN_POINT('Ctrl Pts',(49.0005593529807,47.9365371269326,-1.62251032266728));
#40513=CARTESIAN_POINT('Ctrl Pts',(49.4856489141533,46.7770382825595,-1.68779784193571));
#40514=CARTESIAN_POINT('Ctrl Pts',(49.3794533265802,45.6744932334904,-1.75308536120414));
#40515=CARTESIAN_POINT('Ctrl Pts',(49.2732577390071,44.5719481844213,-1.81837288047257));
#40516=CARTESIAN_POINT('Ctrl Pts',(48.5757770026882,43.5263569306562,-1.883660399741));
#40517=CARTESIAN_POINT('Ctrl Pts',(47.5985993503177,43.004815083087,-1.94894791900943));
#40518=CARTESIAN_POINT('Ctrl Pts',(46.6214216979471,42.4832732355177,-2.01423543827787));
#40519=CARTESIAN_POINT('Ctrl Pts',(45.3645471295248,42.4857807941444,-2.0795229575463));
#40520=CARTESIAN_POINT('Ctrl Pts',(44.3894592148018,43.0112186403657,-2.14481047681473));
#40521=CARTESIAN_POINT('Ctrl Pts',(43.4143713000788,43.536656486587,-2.21009799608316));
#40522=CARTESIAN_POINT('Ctrl Pts',(42.7210700390551,44.585024620403,-2.27538551535159));
#40523=CARTESIAN_POINT('Ctrl Pts',(42.6192749684748,45.6879841639839,-2.34067303462002));
#40524=CARTESIAN_POINT('Ctrl Pts',(42.6097592015399,45.7910884292043,-2.34677608866349));
#40525=CARTESIAN_POINT('Ctrl Pts',(42.6054122782067,45.8946697383908,-2.35287914270696));
#40526=CARTESIAN_POINT('Ctrl Pts',(42.6060554931448,45.9983056788579,-2.35898219675043));
#40527=CARTESIAN_POINT('Ctrl Pts',(44.942095577027,42.0543614925016,0.));
#40528=CARTESIAN_POINT('Ctrl Pts',(44.8266307302754,42.0960014427504,4.42886871984448E-17));
#40529=CARTESIAN_POINT('Ctrl Pts',(44.7135214812892,42.1431495451391,-5.03172530635855E-16));
#40530=CARTESIAN_POINT('Ctrl Pts',(44.6029924719227,42.1954516455847,-3.95516952522712E-16));
#40531=CARTESIAN_POINT('Ctrl Pts',(44.4901067525159,42.2488689363858,-2.85565931943401E-16));
#40532=CARTESIAN_POINT('Ctrl Pts',(44.3799118551348,42.3076629065189,1.44264892563786E-16));
#40533=CARTESIAN_POINT('Ctrl Pts',(44.2726743864217,42.3715030161957,1.66533453693773E-16));
#40534=CARTESIAN_POINT('Ctrl Pts',(44.1607060042205,42.4381595112235,1.89784419924096E-16));
#40535=CARTESIAN_POINT('Ctrl Pts',(44.0519608304487,42.5103177258471,-2.8701074745102E-17));
#40536=CARTESIAN_POINT('Ctrl Pts',(43.946783909642,42.5876437180967,6.93889390390723E-17));
#40537=CARTESIAN_POINT('Ctrl Pts',(43.8547541039362,42.655303961315,1.55217701100225E-16));
#40538=CARTESIAN_POINT('Ctrl Pts',(43.765456599975,42.726921786639,-2.27548279265547E-16));
#40539=CARTESIAN_POINT('Ctrl Pts',(43.6791551681974,42.8022928629544,-2.4980018054066E-16));
#40540=CARTESIAN_POINT('Ctrl Pts',(43.6621958485022,42.8171042299581,-2.54172959760878E-16));
#40541=CARTESIAN_POINT('Ctrl Pts',(43.6453523327829,42.8320605803158,-3.03677325780712E-16));
#40542=CARTESIAN_POINT('Ctrl Pts',(43.6286267795443,42.8471604216388,-2.91433543964104E-16));
#40543=CARTESIAN_POINT('Ctrl Pts',(43.6160043212654,42.858555985923,-2.82193393701082E-16));
#40544=CARTESIAN_POINT('Ctrl Pts',(43.6034490907185,42.8700333172051,-2.10429711059181E-16));
#40545=CARTESIAN_POINT('Ctrl Pts',(43.5909724483507,42.8815818989063,-2.08166817117217E-16));
#40546=CARTESIAN_POINT('Ctrl Pts',(43.5004972697294,42.9653271856134,-1.9175729542341E-16));
#40547=CARTESIAN_POINT('Ctrl Pts',(43.4140102484227,43.05294274113,-3.77380346460283E-16));
#40548=CARTESIAN_POINT('Ctrl Pts',(43.3317690097074,43.1441141207288,-2.77555756156289E-16));
#40549=CARTESIAN_POINT('Ctrl Pts',(43.2498535715234,43.2349243228407,-1.78126623229546E-16));
#40550=CARTESIAN_POINT('Ctrl Pts',(43.1721498672441,43.3292629650551,-1.87918282286947E-16));
#40551=CARTESIAN_POINT('Ctrl Pts',(43.0989549512928,43.4268482158262,-2.91433543964104E-16));
#40552=CARTESIAN_POINT('Ctrl Pts',(43.0268392362533,43.5229946495667,-3.93422555308908E-16));
#40553=CARTESIAN_POINT('Ctrl Pts',(42.9590999801082,43.6222933564817,2.20767809209777E-16));
#40554=CARTESIAN_POINT('Ctrl Pts',(42.8960686068535,43.7244922554337,3.05311331771918E-16));
#40555=CARTESIAN_POINT('Ctrl Pts',(42.8445094854135,43.8080900761696,3.74467206404779E-16));
#40556=CARTESIAN_POINT('Ctrl Pts',(42.7961012115271,43.8936289130541,-5.33629442249871E-16));
#40557=CARTESIAN_POINT('Ctrl Pts',(42.7510518070775,43.980974939088,-4.9960036108132E-16));
#40558=CARTESIAN_POINT('Ctrl Pts',(42.74041777222,44.0015932068954,-4.91567703608139E-16));
#40559=CARTESIAN_POINT('Ctrl Pts',(42.7299710086774,44.0223121796291,-4.88458287812069E-16));
#40560=CARTESIAN_POINT('Ctrl Pts',(42.7197144645543,44.0431301039729,-4.9960036108132E-16));
#40561=CARTESIAN_POINT('Ctrl Pts',(42.7124726338891,44.0578290007056,-5.07467436668099E-16));
#40562=CARTESIAN_POINT('Ctrl Pts',(42.7053263583429,44.0725758823316,1.51950655804844E-16));
#40563=CARTESIAN_POINT('Ctrl Pts',(42.6982817518653,44.0873590202079,1.38777878078145E-16));
#40564=CARTESIAN_POINT('Ctrl Pts',(42.6476425106855,44.1936256919781,4.40870716540678E-17));
#40565=CARTESIAN_POINT('Ctrl Pts',(42.6021758605503,44.3019194279858,-6.69941841300824E-16));
#40566=CARTESIAN_POINT('Ctrl Pts',(42.5621529437021,44.41198419035,-6.38378239159465E-16));
#40567=CARTESIAN_POINT('Ctrl Pts',(42.5229361716051,44.5198320195807,-6.07450393584487E-16));
#40568=CARTESIAN_POINT('Ctrl Pts',(42.4889458186532,44.6293808836332,-3.54776608850978E-16));
#40569=CARTESIAN_POINT('Ctrl Pts',(42.4604858664397,44.7404006911176,-2.22044604925031E-16));
#40570=CARTESIAN_POINT('Ctrl Pts',(42.4550252974187,44.7617018977013,-1.96577511259863E-16));
#40571=CARTESIAN_POINT('Ctrl Pts',(42.4497684749154,44.7830572714539,-1.49720226808031E-16));
#40572=CARTESIAN_POINT('Ctrl Pts',(42.4447177681396,44.8044652044406,-1.66533453693773E-16));
#40573=CARTESIAN_POINT('Ctrl Pts',(42.4175098232356,44.9197888387505,-2.84861175164851E-16));
#40574=CARTESIAN_POINT('Ctrl Pts',(42.3962790783293,45.0366384306533,-9.22849484574937E-16));
#40575=CARTESIAN_POINT('Ctrl Pts',(42.3809409474924,45.1545774247301,-1.0547118733939E-15));
#40576=CARTESIAN_POINT('Ctrl Pts',(42.3724305620896,45.2200160563527,-1.1278759219288E-15));
#40577=CARTESIAN_POINT('Ctrl Pts',(42.3657352040573,45.2857899368098,1.34755129582655E-16));
#40578=CARTESIAN_POINT('Ctrl Pts',(42.3608470177873,45.3518224752913,1.66533453693773E-16));
#40579=CARTESIAN_POINT('Ctrl Pts',(42.3589207553668,45.3778435780852,1.79056174420974E-16));
#40580=CARTESIAN_POINT('Ctrl Pts',(42.3572751729226,45.4039048254304,-5.56858868693118E-16));
#40581=CARTESIAN_POINT('Ctrl Pts',(42.3559099796205,45.4300014357341,-5.55111512312578E-16));
#40582=CARTESIAN_POINT('Ctrl Pts',(42.3550355815509,45.4467161571147,-5.53992341097868E-16));
#40583=CARTESIAN_POINT('Ctrl Pts',(42.3542762567425,45.4634458531474,-4.42970038635353E-16));
#40584=CARTESIAN_POINT('Ctrl Pts',(42.3536323516061,45.4801738313914,-4.44089209850063E-16));
#40585=CARTESIAN_POINT('Ctrl Pts',(42.3490550645524,45.5990869350797,-4.52044990325077E-16));
#40586=CARTESIAN_POINT('Ctrl Pts',(42.3502944925708,45.7181022972958,-2.70567314906092E-16));
#40587=CARTESIAN_POINT('Ctrl Pts',(42.3571975065646,45.8367846513465,-3.88578058618805E-16));
#40588=CARTESIAN_POINT('Ctrl Pts',(42.3639586270055,45.9530274534999,-5.04163055589147E-16));
#40589=CARTESIAN_POINT('Ctrl Pts',(42.3761534299899,46.0689517074927,-3.47685979037171E-16));
#40590=CARTESIAN_POINT('Ctrl Pts',(42.3936903792512,46.1841385916871,-2.77555756156289E-16));
#40591=CARTESIAN_POINT('Ctrl Pts',(42.4110240724559,46.2979904414069,-2.0823835381404E-16));
#40592=CARTESIAN_POINT('Ctrl Pts',(42.4335771976944,46.4111227280688,-2.32655623883673E-16));
#40593=CARTESIAN_POINT('Ctrl Pts',(42.4613062683471,46.5231086200947,-5.55111512312578E-17));
#40594=CARTESIAN_POINT('Ctrl Pts',(42.4793959719044,46.5961652188794,6.00531616599059E-17));
#40595=CARTESIAN_POINT('Ctrl Pts',(42.4996894082884,46.6687334385816,-3.21939151686953E-16));
#40596=CARTESIAN_POINT('Ctrl Pts',(42.5221838062526,46.7406870735208,-2.77555756156289E-16));
#40597=CARTESIAN_POINT('Ctrl Pts',(42.5314101376854,46.7701996697149,-2.59351405102697E-16));
#40598=CARTESIAN_POINT('Ctrl Pts',(42.5410068236004,46.7996087909298,-9.55235496976607E-16));
#40599=CARTESIAN_POINT('Ctrl Pts',(42.5509740049686,46.8289053625447,-9.99200722162641E-16));
#40600=CARTESIAN_POINT('Ctrl Pts',(42.5570607607216,46.8467961853593,-1.02604939456517E-15));
#40601=CARTESIAN_POINT('Ctrl Pts',(42.5632829918888,46.8646370330611,-8.8363779498305E-16));
#40602=CARTESIAN_POINT('Ctrl Pts',(42.5696388615209,46.8824218237155,-8.32667268468867E-16));
#40603=CARTESIAN_POINT('Ctrl Pts',(42.6078192628296,46.9892569987086,-5.2648176280675E-16));
#40604=CARTESIAN_POINT('Ctrl Pts',(42.6508353549956,47.0941210422799,-1.56418195276785E-15));
#40605=CARTESIAN_POINT('Ctrl Pts',(42.6986278307943,47.1966030771671,-1.38777878078145E-15));
#40606=CARTESIAN_POINT('Ctrl Pts',(42.737019496892,47.2789268320815,-1.24607422239025E-15));
#40607=CARTESIAN_POINT('Ctrl Pts',(42.7784942288083,47.3597131960483,-4.31564916260592E-16));
#40608=CARTESIAN_POINT('Ctrl Pts',(42.8230399677098,47.4387323947075,-2.22044604925031E-16));
#40609=CARTESIAN_POINT('Ctrl Pts',(42.845116479876,47.4778936779992,-1.18208013225659E-16));
#40610=CARTESIAN_POINT('Ctrl Pts',(42.8679475116497,47.5166206644653,-1.64609701332461E-15));
#40611=CARTESIAN_POINT('Ctrl Pts',(42.8915329771438,47.5548836868594,-1.88737914186277E-15));
#40612=CARTESIAN_POINT('Ctrl Pts',(42.9049283273751,47.5766151462621,-2.02441517437781E-15));
#40613=CARTESIAN_POINT('Ctrl Pts',(42.9185688329768,47.598199463855,-2.01487937691598E-16));
#40614=CARTESIAN_POINT('Ctrl Pts',(42.9324408350102,47.6196104178753,-2.77555756156289E-16));
#40615=CARTESIAN_POINT('Ctrl Pts',(42.990991151139,47.7099808001382,-5.9861934940153E-16));
#40616=CARTESIAN_POINT('Ctrl Pts',(43.053708488674,47.7973421754918,-3.6468209649014E-17));
#40617=CARTESIAN_POINT('Ctrl Pts',(43.1205609304308,47.8813134312875,-1.11022302462516E-16));
#40618=CARTESIAN_POINT('Ctrl Pts',(43.1787978512499,47.9544630013906,-1.75968334137956E-16));
#40619=CARTESIAN_POINT('Ctrl Pts',(43.2401733961615,48.0250397128339,-9.64438377216789E-17));
#40620=CARTESIAN_POINT('Ctrl Pts',(43.3046859799344,48.0927658552249,5.55111512312578E-16));
#40621=CARTESIAN_POINT('Ctrl Pts',(43.342705354392,48.1326790848235,9.39711714460504E-16));
#40622=CARTESIAN_POINT('Ctrl Pts',(43.3818146654666,48.1716017370957,-1.4559310714997E-16));
#40623=CARTESIAN_POINT('Ctrl Pts',(43.4219648396841,48.2095124983745,-1.11022302462516E-16));
#40624=CARTESIAN_POINT('Origin',(46.,46.,-5.));
#40625=CARTESIAN_POINT('Origin',(-46.,46.,-9.));
#40626=CARTESIAN_POINT('Ctrl Pts',(-44.696617959125,49.1291532909119,-9.));
#40627=CARTESIAN_POINT('Ctrl Pts',(-44.7904996223388,49.1799520140265,-9.));
#40628=CARTESIAN_POINT('Ctrl Pts',(-44.8867385915556,49.2258395047784,-9.));
#40629=CARTESIAN_POINT('Ctrl Pts',(-44.9849436714741,49.2669286477321,-9.));
#40630=CARTESIAN_POINT('Ctrl Pts',(-45.0854080385689,49.3089630796041,-9.));
#40631=CARTESIAN_POINT('Ctrl Pts',(-45.1879305957063,49.3459761067654,-9.));
#40632=CARTESIAN_POINT('Ctrl Pts',(-45.2921271097238,49.3780462975193,-9.));
#40633=CARTESIAN_POINT('Ctrl Pts',(-45.3228377156123,49.3874985810078,-9.));
#40634=CARTESIAN_POINT('Ctrl Pts',(-45.3536939301342,49.3965211911857,-8.99999999999999));
#40635=CARTESIAN_POINT('Ctrl Pts',(-45.3846863526263,49.4051154095944,-8.99999999999999));
#40636=CARTESIAN_POINT('Ctrl Pts',(-45.4054444996056,49.4108716569141,-8.99999999999999));
#40637=CARTESIAN_POINT('Ctrl Pts',(-45.4262637541538,49.4164357177448,-9.));
#40638=CARTESIAN_POINT('Ctrl Pts',(-45.4471413315095,49.4218078922329,-9.));
#40639=CARTESIAN_POINT('Ctrl Pts',(-45.4677336090854,49.4271066539791,-9.));
#40640=CARTESIAN_POINT('Ctrl Pts',(-45.4883751049533,49.4322167664951,-9.));
#40641=CARTESIAN_POINT('Ctrl Pts',(-45.5090574073606,49.4371376256381,-9.));
#40642=CARTESIAN_POINT('Ctrl Pts',(-45.6183975459561,49.4631524962317,-9.));
#40643=CARTESIAN_POINT('Ctrl Pts',(-45.7289242899367,49.4838942050191,-9.));
#40644=CARTESIAN_POINT('Ctrl Pts',(-45.8402230421101,49.4994553459788,-9.));
#40645=CARTESIAN_POINT('Ctrl Pts',(-45.9357755114348,49.5128149337116,-9.));
#40646=CARTESIAN_POINT('Ctrl Pts',(-46.0318978588596,49.5223554338441,-9.));
#40647=CARTESIAN_POINT('Ctrl Pts',(-46.1283415311861,49.528107995161,-9.));
#40648=CARTESIAN_POINT('Ctrl Pts',(-46.1610023378608,49.530056109418,-9.));
#40649=CARTESIAN_POINT('Ctrl Pts',(-46.1937000754335,49.5315695862222,-9.));
#40650=CARTESIAN_POINT('Ctrl Pts',(-46.2264252947816,49.532648960474,-9.));
#40651=CARTESIAN_POINT('Ctrl Pts',(-46.2453984913202,49.5332747524542,-9.));
#40652=CARTESIAN_POINT('Ctrl Pts',(-46.2643830050267,49.5337546547774,-9.));
#40653=CARTESIAN_POINT('Ctrl Pts',(-46.2833703759129,49.5340886078599,-9.));
#40654=CARTESIAN_POINT('Ctrl Pts',(-46.3983320105817,49.5361105724853,-9.));
#40655=CARTESIAN_POINT('Ctrl Pts',(-46.5131368120173,49.5327826867357,-9.));
#40656=CARTESIAN_POINT('Ctrl Pts',(-46.6273658142106,49.5242071685151,-9.));
#40657=CARTESIAN_POINT('Ctrl Pts',(-46.743194097363,49.5155115874144,-9.));
#40658=CARTESIAN_POINT('Ctrl Pts',(-46.8584311883117,49.5014205980068,-9.));
#40659=CARTESIAN_POINT('Ctrl Pts',(-46.9726597700209,49.4819911111919,-9.));
#40660=CARTESIAN_POINT('Ctrl Pts',(-47.0865466693785,49.4626197421671,-9.));
#40661=CARTESIAN_POINT('Ctrl Pts',(-47.1994319983269,49.4379418269772,-9.));
#40662=CARTESIAN_POINT('Ctrl Pts',(-47.3109081125593,49.4079630393852,-9.));
#40663=CARTESIAN_POINT('Ctrl Pts',(-47.377437977202,49.3900714516277,-9.));
#40664=CARTESIAN_POINT('Ctrl Pts',(-47.4434659580683,49.3702908251682,-9.));
#40665=CARTESIAN_POINT('Ctrl Pts',(-47.5089043530615,49.3486135658251,-9.));
#40666=CARTESIAN_POINT('Ctrl Pts',(-47.5540027434167,49.3336741788828,-9.));
#40667=CARTESIAN_POINT('Ctrl Pts',(-47.5988210839709,49.3178338306162,-9.));
#40668=CARTESIAN_POINT('Ctrl Pts',(-47.6433301230227,49.3010881819055,-9.));
#40669=CARTESIAN_POINT('Ctrl Pts',(-47.6570954003034,49.2959092676296,-9.));
#40670=CARTESIAN_POINT('Ctrl Pts',(-47.6708285427968,49.2906446729309,-9.));
#40671=CARTESIAN_POINT('Ctrl Pts',(-47.6845208156298,49.2852975315791,-9.));
#40672=CARTESIAN_POINT('Ctrl Pts',(-47.7954797276198,49.24196557392,-9.));
#40673=CARTESIAN_POINT('Ctrl Pts',(-47.9039056143507,49.1931603257822,-9.));
#40674=CARTESIAN_POINT('Ctrl Pts',(-48.0093711136693,49.1389414929264,-9.));
#40675=CARTESIAN_POINT('Ctrl Pts',(-48.0319908991973,49.1273128714464,-9.));
#40676=CARTESIAN_POINT('Ctrl Pts',(-48.0544745179869,49.1154350357187,-9.));
#40677=CARTESIAN_POINT('Ctrl Pts',(-48.0768177548194,49.1033082620402,-9.));
#40678=CARTESIAN_POINT('Ctrl Pts',(-48.1769673925503,49.0489521273469,-9.));
#40679=CARTESIAN_POINT('Ctrl Pts',(-48.2742977574197,48.9895986568041,-9.));
#40680=CARTESIAN_POINT('Ctrl Pts',(-48.3686684964881,48.9256373054214,-9.));
#40681=CARTESIAN_POINT('Ctrl Pts',(-48.4650755230169,48.8602958260555,-9.));
#40682=CARTESIAN_POINT('Ctrl Pts',(-48.5583943777551,48.7901450832442,-9.));
#40683=CARTESIAN_POINT('Ctrl Pts',(-48.6484556272283,48.7155495224137,-9.));
#40684=CARTESIAN_POINT('Ctrl Pts',(-48.6989531510327,48.6737236413519,-9.));
#40685=CARTESIAN_POINT('Ctrl Pts',(-48.7484261266963,48.6304994944732,-9.));
#40686=CARTESIAN_POINT('Ctrl Pts',(-48.7968410318596,48.585935306637,-9.));
#40687=CARTESIAN_POINT('Ctrl Pts',(-48.8170290143165,48.5673529911454,-9.));
#40688=CARTESIAN_POINT('Ctrl Pts',(-48.8370329936549,48.5485376335577,-9.));
#40689=CARTESIAN_POINT('Ctrl Pts',(-48.8568503809651,48.5294932599232,-9.));
#40690=CARTESIAN_POINT('Ctrl Pts',(-48.8675819585321,48.5191802872961,-9.));
#40691=CARTESIAN_POINT('Ctrl Pts',(-48.878257268696,48.5088015935768,-9.));
#40692=CARTESIAN_POINT('Ctrl Pts',(-48.8888695308225,48.4983643075092,-9.));
#40693=CARTESIAN_POINT('Ctrl Pts',(-48.9743487820228,48.4142944469096,-9.));
#40694=CARTESIAN_POINT('Ctrl Pts',(-49.0558593342174,48.3263122954055,-9.));
#40695=CARTESIAN_POINT('Ctrl Pts',(-49.1332547753371,48.2348504026783,-9.));
#40696=CARTESIAN_POINT('Ctrl Pts',(-49.2120696940868,48.1417110453766,-9.));
#40697=CARTESIAN_POINT('Ctrl Pts',(-49.2866177625613,48.0449626295991,-9.00000000000001));
#40698=CARTESIAN_POINT('Ctrl Pts',(-49.3567204749084,47.9450119046275,-9.00000000000001));
#40699=CARTESIAN_POINT('Ctrl Pts',(-49.4273913584228,47.8442510951645,-9.00000000000001));
#40700=CARTESIAN_POINT('Ctrl Pts',(-49.4935451434678,47.7402352153407,-9.));
#40701=CARTESIAN_POINT('Ctrl Pts',(-49.5549658356322,47.6333394412306,-9.));
#40702=CARTESIAN_POINT('Ctrl Pts',(-49.5912290899789,47.5702273448256,-9.));
#40703=CARTESIAN_POINT('Ctrl Pts',(-49.6258418069011,47.506110632588,-9.));
#40704=CARTESIAN_POINT('Ctrl Pts',(-49.6587528506667,47.4410612184224,-9.));
#40705=CARTESIAN_POINT('Ctrl Pts',(-49.6760927446588,47.4067885300837,-9.));
#40706=CARTESIAN_POINT('Ctrl Pts',(-49.6929601759713,47.3722568712257,-9.));
#40707=CARTESIAN_POINT('Ctrl Pts',(-49.7093470352523,47.3374764129113,-9.));
#40708=CARTESIAN_POINT('Ctrl Pts',(-49.7168953641755,47.3214553844182,-9.));
#40709=CARTESIAN_POINT('Ctrl Pts',(-49.7243424653822,47.3053799171024,-9.));
#40710=CARTESIAN_POINT('Ctrl Pts',(-49.7316851545068,47.2892561784676,-9.));
#40711=CARTESIAN_POINT('Ctrl Pts',(-49.7841011013623,47.1741565176969,-9.));
#40712=CARTESIAN_POINT('Ctrl Pts',(-49.8310349508625,47.0569637809862,-9.));
#40713=CARTESIAN_POINT('Ctrl Pts',(-49.8723057500299,46.938105693547,-9.));
#40714=CARTESIAN_POINT('Ctrl Pts',(-49.9136563789374,46.8190176999652,-9.));
#40715=CARTESIAN_POINT('Ctrl Pts',(-49.9493226072422,46.6982571648312,-9.));
#40716=CARTESIAN_POINT('Ctrl Pts',(-49.9790844956097,46.5762183008083,-9.));
#40717=CARTESIAN_POINT('Ctrl Pts',(-50.0083336073707,46.4562820814085,-9.));
#40718=CARTESIAN_POINT('Ctrl Pts',(-50.0318805036137,46.335110417964,-9.));
#40719=CARTESIAN_POINT('Ctrl Pts',(-50.049472608,46.2130542301493,-9.));
#40720=CARTESIAN_POINT('Ctrl Pts',(-50.060364521469,46.1374847924716,-9.));
#40721=CARTESIAN_POINT('Ctrl Pts',(-50.0689728987746,46.0615758765585,-9.));
#40722=CARTESIAN_POINT('Ctrl Pts',(-50.0752280523108,45.9854081433151,-9.));
#40723=CARTESIAN_POINT('Ctrl Pts',(-50.0806294959961,45.9196358614081,-9.));
#40724=CARTESIAN_POINT('Ctrl Pts',(-50.0842760830383,45.8536705349028,-9.));
#40725=CARTESIAN_POINT('Ctrl Pts',(-50.0861963379778,45.7875630405759,-9.));
#40726=CARTESIAN_POINT('Ctrl Pts',(-49.4256147683784,43.7746037524369,-9.));
#40727=CARTESIAN_POINT('Ctrl Pts',(-49.3489156851343,43.6758334442189,-9.));
#40728=CARTESIAN_POINT('Ctrl Pts',(-49.2674578564169,43.5810567995784,-9.));
#40729=CARTESIAN_POINT('Ctrl Pts',(-49.181649129582,43.490413103789,-9.));
#40730=CARTESIAN_POINT('Ctrl Pts',(-49.0946355246868,43.3984966400144,-9.));
#40731=CARTESIAN_POINT('Ctrl Pts',(-49.0031471845609,43.3108296011929,-9.00000000000001));
#40732=CARTESIAN_POINT('Ctrl Pts',(-48.9075792861019,43.2276011445689,-9.));
#40733=CARTESIAN_POINT('Ctrl Pts',(-48.8671606571012,43.1924012483188,-9.));
#40734=CARTESIAN_POINT('Ctrl Pts',(-48.8260120201089,43.157995852241,-9.));
#40735=CARTESIAN_POINT('Ctrl Pts',(-48.7841622188313,43.124401852238,-9.));
#40736=CARTESIAN_POINT('Ctrl Pts',(-48.7601537028534,43.1051295483988,-9.));
#40737=CARTESIAN_POINT('Ctrl Pts',(-48.7359099990676,43.0861210782675,-9.));
#40738=CARTESIAN_POINT('Ctrl Pts',(-48.711461905359,43.0673988919303,-9.));
#40739=CARTESIAN_POINT('Ctrl Pts',(-48.6120353794127,42.9912587246101,-9.));
#40740=CARTESIAN_POINT('Ctrl Pts',(-48.5091652266986,42.9197949105889,-9.));
#40741=CARTESIAN_POINT('Ctrl Pts',(-48.403244860894,42.8531794238142,-9.));
#40742=CARTESIAN_POINT('Ctrl Pts',(-48.3152213037729,42.7978196064578,-9.));
#40743=CARTESIAN_POINT('Ctrl Pts',(-48.2250904620759,42.7458088667081,-9.));
#40744=CARTESIAN_POINT('Ctrl Pts',(-48.1330695305898,42.6972719088762,-9.));
#40745=CARTESIAN_POINT('Ctrl Pts',(-48.0928103730647,42.6760369898247,-9.));
#40746=CARTESIAN_POINT('Ctrl Pts',(-48.0521893744864,42.655467290417,-9.));
#40747=CARTESIAN_POINT('Ctrl Pts',(-48.0112245259672,42.6355747667283,-9.));
#40748=CARTESIAN_POINT('Ctrl Pts',(-47.988854995164,42.6247121262574,-9.));
#40749=CARTESIAN_POINT('Ctrl Pts',(-47.9663829311551,42.6140514282838,-9.));
#40750=CARTESIAN_POINT('Ctrl Pts',(-47.943811261034,42.6035947399501,-9.));
#40751=CARTESIAN_POINT('Ctrl Pts',(-47.9276114508231,42.5960899179529,-9.));
#40752=CARTESIAN_POINT('Ctrl Pts',(-47.9113688772611,42.5886941448197,-9.));
#40753=CARTESIAN_POINT('Ctrl Pts',(-47.8950854098512,42.5814081483561,-9.));
#40754=CARTESIAN_POINT('Ctrl Pts',(-47.783364187915,42.5314187691019,-9.));
#40755=CARTESIAN_POINT('Ctrl Pts',(-47.6697083738472,42.4865878815946,-9.));
#40756=CARTESIAN_POINT('Ctrl Pts',(-47.5544847720591,42.4470736397854,-9.));
#40757=CARTESIAN_POINT('Ctrl Pts',(-47.4401244943331,42.4078554622826,-9.));
#40758=CARTESIAN_POINT('Ctrl Pts',(-47.3242190140508,42.373874375732,-9.));
#40759=CARTESIAN_POINT('Ctrl Pts',(-47.2071179764348,42.3453353099349,-9.));
#40760=CARTESIAN_POINT('Ctrl Pts',(-47.0931610163015,42.3175624972469,-9.));
#40761=CARTESIAN_POINT('Ctrl Pts',(-46.9780711398153,42.2949434018992,-9.));
#40762=CARTESIAN_POINT('Ctrl Pts',(-46.8621731460597,42.2777157561986,-9.));
#40763=CARTESIAN_POINT('Ctrl Pts',(-46.7940396442691,42.2675880586332,-9.));
#40764=CARTESIAN_POINT('Ctrl Pts',(-46.7256269603666,42.2593245531098,-9.));
#40765=CARTESIAN_POINT('Ctrl Pts',(-46.6570029378699,42.252981774315,-9.));
#40766=CARTESIAN_POINT('Ctrl Pts',(-46.6091492630523,42.2485587565022,-9.));
#40767=CARTESIAN_POINT('Ctrl Pts',(-46.5611928515148,42.2450698598449,-9.));
#40768=CARTESIAN_POINT('Ctrl Pts',(-46.5131573311611,42.2425360831896,-9.));
#40769=CARTESIAN_POINT('Ctrl Pts',(-46.4976790891648,42.2417196371941,-9.));
#40770=CARTESIAN_POINT('Ctrl Pts',(-46.48219606998,42.2410025896726,-9.));
#40771=CARTESIAN_POINT('Ctrl Pts',(-46.4667175316418,42.2403857716101,-9.));
#40772=CARTESIAN_POINT('Ctrl Pts',(-46.3509701417906,42.2357732507639,-9.));
#40773=CARTESIAN_POINT('Ctrl Pts',(-46.2353324238638,42.2367536523897,-9.));
#40774=CARTESIAN_POINT('Ctrl Pts',(-46.1201180919468,42.243510424435,-9.));
#40775=CARTESIAN_POINT('Ctrl Pts',(-46.0928482837347,42.2451096688584,-9.));
#40776=CARTESIAN_POINT('Ctrl Pts',(-46.0656022142227,42.2470327395972,-9.));
#40777=CARTESIAN_POINT('Ctrl Pts',(-46.0383840979687,42.2492824979304,-9.));
#40778=CARTESIAN_POINT('Ctrl Pts',(-45.9217097098913,42.2589264120937,-9.));
#40779=CARTESIAN_POINT('Ctrl Pts',(-45.8055476026248,42.2745693849197,-9.));
#40780=CARTESIAN_POINT('Ctrl Pts',(-45.6902605716738,42.2959681457642,-9.));
#40781=CARTESIAN_POINT('Ctrl Pts',(-45.5740232449465,42.3175432937693,-9.));
#40782=CARTESIAN_POINT('Ctrl Pts',(-45.4586746610144,42.344970033424,-9.));
#40783=CARTESIAN_POINT('Ctrl Pts',(-45.3446113258486,42.3780453905501,-9.));
#40784=CARTESIAN_POINT('Ctrl Pts',(-45.2880066971767,42.3944592390983,-9.));
#40785=CARTESIAN_POINT('Ctrl Pts',(-45.2317190441744,42.4122648380503,-9.));
#40786=CARTESIAN_POINT('Ctrl Pts',(-45.1758000085569,42.4314409547508,-9.));
#40787=CARTESIAN_POINT('Ctrl Pts',(-45.1531794291222,42.4391981498863,-9.));
#40788=CARTESIAN_POINT('Ctrl Pts',(-45.1306191973553,42.4471796404986,-9.));
#40789=CARTESIAN_POINT('Ctrl Pts',(-45.108122848517,42.4553841175605,-9.));
#40790=CARTESIAN_POINT('Ctrl Pts',(-45.0929026543741,42.4609349620386,-9.));
#40791=CARTESIAN_POINT('Ctrl Pts',(-45.077712071619,42.4665878060077,-9.));
#40792=CARTESIAN_POINT('Ctrl Pts',(-45.0625649705552,42.4723372085153,-9.));
#40793=CARTESIAN_POINT('Ctrl Pts',(-44.9541043446988,42.5135057325545,-9.));
#40794=CARTESIAN_POINT('Ctrl Pts',(-44.8477009223801,42.5596824806258,-9.));
#40795=CARTESIAN_POINT('Ctrl Pts',(-44.7436965702623,42.6106187568676,-9.));
#40796=CARTESIAN_POINT('Ctrl Pts',(-44.63979376496,42.6615053004152,-9.));
#40797=CARTESIAN_POINT('Ctrl Pts',(-44.5382846082116,42.7171426900045,-9.));
#40798=CARTESIAN_POINT('Ctrl Pts',(-44.4395391052149,42.7773258218427,-9.));
#40799=CARTESIAN_POINT('Ctrl Pts',(-44.3421856021374,42.8366605614795,-9.));
#40800=CARTESIAN_POINT('Ctrl Pts',(-44.2475177836353,42.9004144122074,-9.));
#40801=CARTESIAN_POINT('Ctrl Pts',(-44.1559283796025,42.9684232317984,-9.));
#40802=CARTESIAN_POINT('Ctrl Pts',(-44.1056662078478,43.0057449177206,-9.));
#40803=CARTESIAN_POINT('Ctrl Pts',(-44.0563318447938,43.0443485309563,-9.));
#40804=CARTESIAN_POINT('Ctrl Pts',(-44.007996167856,43.0842101741848,-9.));
#40805=CARTESIAN_POINT('Ctrl Pts',(-43.9809731477155,43.1064956174855,-9.));
#40806=CARTESIAN_POINT('Ctrl Pts',(-43.9542623568393,43.1291743065356,-9.));
#40807=CARTESIAN_POINT('Ctrl Pts',(-43.9278768328444,43.1522423177272,-9.));
#40808=CARTESIAN_POINT('Ctrl Pts',(-43.9114600205802,43.1665950063119,-9.));
#40809=CARTESIAN_POINT('Ctrl Pts',(-43.8951656324309,43.1811017137048,-9.));
#40810=CARTESIAN_POINT('Ctrl Pts',(-43.8790187657196,43.195741331518,-9.));
#40811=CARTESIAN_POINT('Ctrl Pts',(-43.7964028050777,43.2706454049021,-9.));
#40812=CARTESIAN_POINT('Ctrl Pts',(-43.7175427311938,43.3491132482605,-9.));
#40813=CARTESIAN_POINT('Ctrl Pts',(-43.642772806583,43.4309575041822,-9.));
#40814=CARTESIAN_POINT('Ctrl Pts',(-43.5691145212186,43.5115849434834,-9.));
#40815=CARTESIAN_POINT('Ctrl Pts',(-43.4994251726958,43.5954897325599,-9.));
#40816=CARTESIAN_POINT('Ctrl Pts',(-43.4340666403476,43.6825192687086,-9.));
#40817=CARTESIAN_POINT('Ctrl Pts',(-43.3705939763842,43.7670376369213,-9.));
#40818=CARTESIAN_POINT('Ctrl Pts',(-43.3112055155065,43.854503559686,-9.));
#40819=CARTESIAN_POINT('Ctrl Pts',(-43.2562784669833,43.9447942667368,-9.));
#40820=CARTESIAN_POINT('Ctrl Pts',(-43.2286242788146,43.9902530392324,-9.));
#40821=CARTESIAN_POINT('Ctrl Pts',(-43.2021017428087,44.036428070575,-9.));
#40822=CARTESIAN_POINT('Ctrl Pts',(-43.176763938175,44.0833047759387,-9.));
#40823=CARTESIAN_POINT('Ctrl Pts',(-43.1505637145409,44.1317770165891,-9.00000000000001));
#40824=CARTESIAN_POINT('Ctrl Pts',(-43.1256303008689,44.1809995875891,-9.));
#40825=CARTESIAN_POINT('Ctrl Pts',(-43.1019723047815,44.2309203707047,-9.));
#40826=CARTESIAN_POINT('Origin',(-46.,46.,2.76038497140452));
#40827=CARTESIAN_POINT('Ctrl Pts',(-50.0901569545599,46.0018621213198,-0.364615028595479));
#40828=CARTESIAN_POINT('Ctrl Pts',(-50.0908670066917,46.1207444808691,-0.370425837919348));
#40829=CARTESIAN_POINT('Ctrl Pts',(-50.0327398704972,47.5746590118461,-0.441524166511649));
#40830=CARTESIAN_POINT('Ctrl Pts',(-48.2991248954935,50.2221780497669,-0.577910014372381));
#40831=CARTESIAN_POINT('Ctrl Pts',(-43.7551468972239,50.2508324710758,-0.773772572177673));
#40832=CARTESIAN_POINT('Ctrl Pts',(-41.216941413185,46.4820553508686,-0.969635129982968));
#40833=CARTESIAN_POINT('Ctrl Pts',(-42.9521748839983,42.2823237877054,-1.16549768778826));
#40834=CARTESIAN_POINT('Ctrl Pts',(-47.4105428653624,41.4043187587238,-1.36136024559355));
#40835=CARTESIAN_POINT('Ctrl Pts',(-49.8549759634627,43.8716102112686,-1.51106602586263));
#40836=CARTESIAN_POINT('Ctrl Pts',(-50.0859938031716,45.6034148261523,-1.59548428686327));
#40837=CARTESIAN_POINT('Ctrl Pts',(-50.0828667635534,45.9966889209644,-1.61461502859548));
#40838=CARTESIAN_POINT('Ctrl Pts',(-50.0805800719598,45.9961676961768,-0.260384971404518));
#40839=CARTESIAN_POINT('Ctrl Pts',(-50.074537021219,46.8968546972385,-0.304165019473208));
#40840=CARTESIAN_POINT('Ctrl Pts',(-49.3426925538961,49.1524151445276,-0.413232586810328));
#40841=CARTESIAN_POINT('Ctrl Pts',(-45.6441921094362,50.7932694144525,-0.587587673415879));
#40842=CARTESIAN_POINT('Ctrl Pts',(-41.8104748163565,48.3572313450219,-0.783450231221174));
#40843=CARTESIAN_POINT('Ctrl Pts',(-41.7184176569125,43.8134905867626,-0.979312789026467));
#40844=CARTESIAN_POINT('Ctrl Pts',(-45.4525333012251,41.2240979371497,-1.17517534683176));
#40845=CARTESIAN_POINT('Ctrl Pts',(-49.2692586484769,42.740078891428,-1.35219940762444));
#40846=CARTESIAN_POINT('Ctrl Pts',(-50.0753332382032,45.0485594015793,-1.4639359491487));
#40847=CARTESIAN_POINT('Ctrl Pts',(-50.0830244466748,46.0033346430494,-1.51038497140452));
#40848=CARTESIAN_POINT('Ctrl Pts',(-43.4267655729853,48.2065515280923,0.));
#40849=CARTESIAN_POINT('Ctrl Pts',(-42.7026396483563,47.3620909591791,-0.0652875192684312));
#40850=CARTESIAN_POINT('Ctrl Pts',(-42.1622053861818,44.918494548316,-0.195862557805293));
#40851=CARTESIAN_POINT('Ctrl Pts',(-44.780472506665,42.1996731612585,-0.391725115610587));
#40852=CARTESIAN_POINT('Ctrl Pts',(-48.4895452540558,42.8839744308764,-0.58758767341588));
#40853=CARTESIAN_POINT('Ctrl Pts',(-49.9737285271075,46.3485994374708,-0.783450231221174));
#40854=CARTESIAN_POINT('Ctrl Pts',(-47.9078234062422,49.5035809165722,-0.979312789026467));
#40855=CARTESIAN_POINT('Ctrl Pts',(-44.1372115532105,49.5273584746216,-1.17517534683176));
#40856=CARTESIAN_POINT('Ctrl Pts',(-42.0309980796435,46.4000115362563,-1.37103790463705));
#40857=CARTESIAN_POINT('Ctrl Pts',(-43.4709020350142,42.9150568076804,-1.56690046244235));
#40858=CARTESIAN_POINT('Ctrl Pts',(-47.170474339746,42.186484580755,-1.76276302024764));
#40859=CARTESIAN_POINT('Ctrl Pts',(-49.8242647271257,44.8650910620353,-1.95862557805294));
#40860=CARTESIAN_POINT('Ctrl Pts',(-49.0612252674608,48.5577200654077,-2.15448813585823));
#40861=CARTESIAN_POINT('Ctrl Pts',(-45.5630965935586,49.9651121437844,-2.35035069366352));
#40862=CARTESIAN_POINT('Ctrl Pts',(-42.4553252853163,47.8298346642785,-2.54621325146881));
#40863=CARTESIAN_POINT('Ctrl Pts',(-42.5145843401837,44.0596672136162,-2.74207580927411));
#40864=CARTESIAN_POINT('Ctrl Pts',(-45.6879287513146,42.0231140731554,-2.9379383670794));
#40865=CARTESIAN_POINT('Ctrl Pts',(-49.1400967366528,43.5397551864917,-3.1338009248847));
#40866=CARTESIAN_POINT('Ctrl Pts',(-49.7867088499387,47.2545309657486,-3.32966348268999));
#40867=CARTESIAN_POINT('Ctrl Pts',(-47.0500419029285,49.848431304961,-3.52552604049528));
#40868=CARTESIAN_POINT('Ctrl Pts',(-43.3752028262867,49.0039060474354,-3.72138859830057));
#40869=CARTESIAN_POINT('Ctrl Pts',(-42.0455192855114,45.4755059780424,-3.91725115610587));
#40870=CARTESIAN_POINT('Ctrl Pts',(-44.2490125041704,42.4157212082961,-4.11311371391116));
#40871=CARTESIAN_POINT('Ctrl Pts',(-48.0169458506302,42.5583519744937,-4.30897627171646));
#40872=CARTESIAN_POINT('Ctrl Pts',(-49.9828154853804,45.7759631753024,-4.50483882952175));
#40873=CARTESIAN_POINT('Ctrl Pts',(-48.3901923325963,49.1937426785204,-4.70070138732704));
#40874=CARTESIAN_POINT('Ctrl Pts',(-44.662024060862,49.7580356671663,-4.89656394513234));
#40875=CARTESIAN_POINT('Ctrl Pts',(-42.1292859407132,46.9646680087392,-5.09242650293763));
#40876=CARTESIAN_POINT('Ctrl Pts',(-43.0548822895087,43.3094065081176,-5.28828906074292));
#40877=CARTESIAN_POINT('Ctrl Pts',(-46.6118282782839,42.0580870306127,-5.48415161854822));
#40878=CARTESIAN_POINT('Ctrl Pts',(-49.6221291986836,44.3287155200276,-5.68001417635351));
#40879=CARTESIAN_POINT('Ctrl Pts',(-49.3961966506987,48.0925725355867,-5.87587673415881));
#40880=CARTESIAN_POINT('Ctrl Pts',(-46.1358928070669,49.9867963332999,-6.0717392919641));
#40881=CARTESIAN_POINT('Ctrl Pts',(-42.7541738021461,48.3189705369532,-6.2676018497694));
#40882=CARTESIAN_POINT('Ctrl Pts',(-42.2724762525193,44.5792337098036,-6.46346440757469));
#40883=CARTESIAN_POINT('Ctrl Pts',(-45.1211774786945,42.1088967349022,-6.65932696537998));
#40884=CARTESIAN_POINT('Ctrl Pts',(-48.7550742096251,43.1151118165565,-6.85518952318527));
#40885=CARTESIAN_POINT('Ctrl Pts',(-49.9274151919628,46.6988625110037,-7.05105208099057));
#40886=CARTESIAN_POINT('Ctrl Pts',(-47.5907668890102,49.658208957394,-7.24691463879586));
#40887=CARTESIAN_POINT('Ctrl Pts',(-43.8328182515428,49.3490808096796,-7.44277719660115));
#40888=CARTESIAN_POINT('Ctrl Pts',(-42.0111861586986,46.0476882822715,-7.63863975440645));
#40889=CARTESIAN_POINT('Ctrl Pts',(-43.7533595145448,42.7036660446114,-7.83450231221174));
#40890=CARTESIAN_POINT('Ctrl Pts',(-47.5029152312013,42.3048367721094,-8.03036487001704));
#40891=CARTESIAN_POINT('Ctrl Pts',(-49.9094791054614,45.2074019114722,-8.22622742782233));
#40892=CARTESIAN_POINT('Ctrl Pts',(-48.8234714323549,48.8183112778844,-8.42208998562762));
#40893=CARTESIAN_POINT('Ctrl Pts',(-45.2139870282641,49.9107829885096,-8.61795254343291));
#40894=CARTESIAN_POINT('Ctrl Pts',(-42.3084375115684,47.5099063922733,-8.81381510123821));
#40895=CARTESIAN_POINT('Ctrl Pts',(-42.6977455577746,43.7583829526296,-9.00967765904351));
#40896=CARTESIAN_POINT('Ctrl Pts',(-46.0445165417033,42.0129785782631,-9.20554021684879));
#40897=CARTESIAN_POINT('Ctrl Pts',(-48.2365749371353,43.2205019121706,-9.33611525538566));
#40898=CARTESIAN_POINT('Ctrl Pts',(-48.8425893907247,44.1533569326372,-9.40140277465409));
#40899=CARTESIAN_POINT('Ctrl Pts',(-43.2508390065835,48.3574087643591,0.133800924884696));
#40900=CARTESIAN_POINT('Ctrl Pts',(-42.4772061321698,47.4552142218946,0.0685134056162645));
#40901=CARTESIAN_POINT('Ctrl Pts',(-41.8998235285957,44.8445543201494,-0.0620616329205977));
#40902=CARTESIAN_POINT('Ctrl Pts',(-44.6970960049819,41.9398528957881,-0.257924190725891));
#40903=CARTESIAN_POINT('Ctrl Pts',(-48.6597501696476,42.6709383882054,-0.453786748531184));
#40904=CARTESIAN_POINT('Ctrl Pts',(-50.245403897314,46.3724324397966,-0.649649306336479));
#40905=CARTESIAN_POINT('Ctrl Pts',(-48.0382572359926,49.7431132943038,-0.845511864141771));
#40906=CARTESIAN_POINT('Ctrl Pts',(-44.0098566678816,49.7685164734396,-1.04137442194707));
#40907=CARTESIAN_POINT('Ctrl Pts',(-41.7596458574907,46.4273594744604,-1.23723697975236));
#40908=CARTESIAN_POINT('Ctrl Pts',(-43.2979929846756,42.7041458010221,-1.43309953755765));
#40909=CARTESIAN_POINT('Ctrl Pts',(-47.2504971816181,41.9257626400779,-1.62896209536295));
#40910=CARTESIAN_POINT('Ctrl Pts',(-50.0857215751267,44.7874997510615,-1.82482465316824));
#40911=CARTESIAN_POINT('Ctrl Pts',(-49.2705147300271,48.732585947894,-2.02068721097353));
#40912=CARTESIAN_POINT('Ctrl Pts',(-45.5332264366317,50.2361984301837,-2.21654976877883));
#40913=CARTESIAN_POINT('Ctrl Pts',(-42.2129834119841,47.9549365695654,-2.41241232658412));
#40914=CARTESIAN_POINT('Ctrl Pts',(-42.2762938824324,43.927010786669,-2.60827488438942));
#40915=CARTESIAN_POINT('Ctrl Pts',(-45.6665931035876,41.7512228382424,-2.80413744219471));
#40916=CARTESIAN_POINT('Ctrl Pts',(-49.3547784738662,43.3715534797197,-3.));
#40917=CARTESIAN_POINT('Ctrl Pts',(-50.0455980824701,47.3403005804141,-3.1958625578053));
#40918=CARTESIAN_POINT('Ctrl Pts',(-47.1218310351665,50.111540370504,-3.39172511561058));
#40919=CARTESIAN_POINT('Ctrl Pts',(-43.195751024529,49.2092767168044,-3.58758767341588));
#40920=CARTESIAN_POINT('Ctrl Pts',(-41.7751598473278,45.4396474369734,-3.78345023122118));
#40921=CARTESIAN_POINT('Ctrl Pts',(-44.1293012121405,42.1706716884267,-3.97931278902647));
#40922=CARTESIAN_POINT('Ctrl Pts',(-48.1548401498805,42.3230538168387,-4.17517534683176));
#40923=CARTESIAN_POINT('Ctrl Pts',(-50.2551121116026,45.7606462539591,-4.37103790463705));
#40924=CARTESIAN_POINT('Ctrl Pts',(-48.5536047001984,49.4120920747139,-4.56690046244235));
#40925=CARTESIAN_POINT('Ctrl Pts',(-44.5705494907919,50.0149645751583,-4.76276302024764));
#40926=CARTESIAN_POINT('Ctrl Pts',(-41.8646534506358,47.0306203093587,-4.95862557805294));
#40927=CARTESIAN_POINT('Ctrl Pts',(-42.8535308537372,43.125456351987,-5.15448813585823));
#40928=CARTESIAN_POINT('Ctrl Pts',(-46.6536576767624,41.7885868224394,-5.35035069366352));
#40929=CARTESIAN_POINT('Ctrl Pts',(-49.8697664703983,44.2144533537222,-5.54621325146882));
#40930=CARTESIAN_POINT('Ctrl Pts',(-49.6283873944997,48.2356372704853,-5.74207580927411));
#40931=CARTESIAN_POINT('Ctrl Pts',(-46.1451835093422,50.2593651216301,-5.9379383670794));
#40932=CARTESIAN_POINT('Ctrl Pts',(-42.532263566479,48.4775136218234,-6.1338009248847));
#40933=CARTESIAN_POINT('Ctrl Pts',(-42.0176333795999,44.4820989394656,-6.32966348268999));
#40934=CARTESIAN_POINT('Ctrl Pts',(-45.0610942515207,41.8428702781764,-6.52552604049528));
#40935=CARTESIAN_POINT('Ctrl Pts',(-48.9434327753248,42.9178781454855,-6.72138859830058));
#40936=CARTESIAN_POINT('Ctrl Pts',(-50.1959242179196,46.7466422549156,-6.91725115610587));
#40937=CARTESIAN_POINT('Ctrl Pts',(-47.6995242388231,49.9083129254967,-7.11311371391117));
#40938=CARTESIAN_POINT('Ctrl Pts',(-43.6846526433991,49.5780503436108,-7.30897627171646));
#40939=CARTESIAN_POINT('Ctrl Pts',(-41.7384794376362,46.0509486287325,-7.50483882952175));
#40940=CARTESIAN_POINT('Ctrl Pts',(-43.5997614815028,42.4783027009544,-7.70070138732705));
#40941=CARTESIAN_POINT('Ctrl Pts',(-47.6056663499655,42.0522063191074,-7.89656394513234));
#40942=CARTESIAN_POINT('Ctrl Pts',(-50.176761879321,45.1532136654315,-8.09242650293763));
#40943=CARTESIAN_POINT('Ctrl Pts',(-49.0165061707422,49.0109932274824,-8.28828906074293));
#40944=CARTESIAN_POINT('Ctrl Pts',(-45.1602489926568,50.1781549060808,-8.48415161854822));
#40945=CARTESIAN_POINT('Ctrl Pts',(-42.056053233467,47.6131354818549,-8.68001417635352));
#40946=CARTESIAN_POINT('Ctrl Pts',(-42.4719774430211,43.6051283613683,-8.8758767341588));
#40947=CARTESIAN_POINT('Ctrl Pts',(-46.0475600430057,41.7403944011151,-9.0717392919641));
#40948=CARTESIAN_POINT('Ctrl Pts',(-48.3894848100407,43.0304735378497,-9.20231433050096));
#40949=CARTESIAN_POINT('Ctrl Pts',(-49.036931183276,44.0271058725704,-9.2676018497694));
#40950=CARTESIAN_POINT('Ctrl Pts',(-43.0749124401816,48.5082660006259,0.267601849769391));
#40951=CARTESIAN_POINT('Ctrl Pts',(-42.2517726159832,47.54833748461,0.20231433050096));
#40952=CARTESIAN_POINT('Ctrl Pts',(-41.6374416710097,44.7706140919828,0.0717392919640979));
#40953=CARTESIAN_POINT('Ctrl Pts',(-44.6137195032988,41.6800326303177,-0.124123265841196));
#40954=CARTESIAN_POINT('Ctrl Pts',(-48.8299550852394,42.4579023455342,-0.319985823646489));
#40955=CARTESIAN_POINT('Ctrl Pts',(-50.5170792675203,46.3962654421224,-0.515848381451782));
#40956=CARTESIAN_POINT('Ctrl Pts',(-48.1686910657431,49.9826456720353,-0.711710939257076));
#40957=CARTESIAN_POINT('Ctrl Pts',(-43.8825017825528,50.0096744722577,-0.907573497062369));
#40958=CARTESIAN_POINT('Ctrl Pts',(-41.4882936353378,46.4547074126645,-1.10343605486766));
#40959=CARTESIAN_POINT('Ctrl Pts',(-43.1250839343369,42.4932347943637,-1.29929861267296));
#40960=CARTESIAN_POINT('Ctrl Pts',(-47.3305200234903,41.6650406994009,-1.49516117047825));
#40961=CARTESIAN_POINT('Ctrl Pts',(-50.3471784231277,44.7099084400878,-1.69102372828354));
#40962=CARTESIAN_POINT('Ctrl Pts',(-49.4798041925933,48.9074518303804,-1.88688628608884));
#40963=CARTESIAN_POINT('Ctrl Pts',(-45.5033562797049,50.507284716583,-2.08274884389413));
#40964=CARTESIAN_POINT('Ctrl Pts',(-41.9706415386519,48.0800384748524,-2.27861140169942));
#40965=CARTESIAN_POINT('Ctrl Pts',(-42.0380034246811,43.7943543597217,-2.47447395950472));
#40966=CARTESIAN_POINT('Ctrl Pts',(-45.6452574558605,41.4793316033294,-2.67033651731001));
#40967=CARTESIAN_POINT('Ctrl Pts',(-49.5694602110796,43.2033517729476,-2.8661990751153));
#40968=CARTESIAN_POINT('Ctrl Pts',(-50.3044873150015,47.4260701950796,-3.0620616329206));
#40969=CARTESIAN_POINT('Ctrl Pts',(-47.1936201674044,50.3746494360471,-3.25792419072589));
#40970=CARTESIAN_POINT('Ctrl Pts',(-43.0162992227714,49.4146473861733,-3.45378674853119));
#40971=CARTESIAN_POINT('Ctrl Pts',(-41.5048004091442,45.4037888959043,-3.64964930633648));
#40972=CARTESIAN_POINT('Ctrl Pts',(-44.0095899201106,41.9256221685573,-3.84551186414177));
#40973=CARTESIAN_POINT('Ctrl Pts',(-48.2927344491307,42.0877556591837,-4.04137442194706));
#40974=CARTESIAN_POINT('Ctrl Pts',(-50.5274087378249,45.7453293326157,-4.23723697975236));
#40975=CARTESIAN_POINT('Ctrl Pts',(-48.7170170678005,49.6304414709075,-4.43309953755765));
#40976=CARTESIAN_POINT('Ctrl Pts',(-44.4790749207218,50.2718934831503,-4.62896209536295));
#40977=CARTESIAN_POINT('Ctrl Pts',(-41.6000209605584,47.0965726099784,-4.82482465316824));
#40978=CARTESIAN_POINT('Ctrl Pts',(-42.6521794179657,42.9415061958563,-5.02068721097354));
#40979=CARTESIAN_POINT('Ctrl Pts',(-46.6954870752408,41.5190866142661,-5.21654976877883));
#40980=CARTESIAN_POINT('Ctrl Pts',(-50.117403742113,44.1001911874169,-5.41241232658411));
#40981=CARTESIAN_POINT('Ctrl Pts',(-49.8605781383007,48.3787020053837,-5.60827488438942));
#40982=CARTESIAN_POINT('Ctrl Pts',(-46.1544742116175,50.5319339099603,-5.8041374421947));
#40983=CARTESIAN_POINT('Ctrl Pts',(-42.3103533308119,48.6360567066936,-6.00000000000001));
#40984=CARTESIAN_POINT('Ctrl Pts',(-41.7627905066804,44.3849641691278,-6.19586255780529));
#40985=CARTESIAN_POINT('Ctrl Pts',(-45.0010110243469,41.5768438214505,-6.39172511561059));
#40986=CARTESIAN_POINT('Ctrl Pts',(-49.1317913410244,42.7206444744145,-6.58758767341588));
#40987=CARTESIAN_POINT('Ctrl Pts',(-50.4644332438766,46.7944219988274,-6.78345023122118));
#40988=CARTESIAN_POINT('Ctrl Pts',(-47.8082815886359,50.1584168935994,-6.97931278902647));
#40989=CARTESIAN_POINT('Ctrl Pts',(-43.5364870352555,49.807019877542,-7.17517534683176));
#40990=CARTESIAN_POINT('Ctrl Pts',(-41.4657727165736,46.0542089751936,-7.37103790463705));
#40991=CARTESIAN_POINT('Ctrl Pts',(-43.4461634484607,42.2529393572974,-7.56690046244235));
#40992=CARTESIAN_POINT('Ctrl Pts',(-47.7084174687297,41.7995758661054,-7.76276302024764));
#40993=CARTESIAN_POINT('Ctrl Pts',(-50.4440446531807,45.0990254193909,-7.95862557805294));
#40994=CARTESIAN_POINT('Ctrl Pts',(-49.2095409091294,49.2036751770803,-8.15448813585823));
#40995=CARTESIAN_POINT('Ctrl Pts',(-45.1065109570496,50.4455268236521,-8.35035069366353));
#40996=CARTESIAN_POINT('Ctrl Pts',(-41.8036689553657,47.7163645714366,-8.54621325146882));
#40997=CARTESIAN_POINT('Ctrl Pts',(-42.2462093282676,43.451873770107,-8.74207580927411));
#40998=CARTESIAN_POINT('Ctrl Pts',(-46.0506035443081,41.4678102239671,-8.93793836707941));
#40999=CARTESIAN_POINT('Ctrl Pts',(-48.5423946829461,42.8404451635287,-9.06851340561627));
#41000=CARTESIAN_POINT('Ctrl Pts',(-49.2312729758272,43.9008548125037,-9.1338009248847));
#41001=CARTESIAN_POINT('Ctrl Pts',(-42.8989858737798,48.6591232368927,0.401402774654087));
#41002=CARTESIAN_POINT('Ctrl Pts',(-42.0263390997967,47.6414607473255,0.336115255385656));
#41003=CARTESIAN_POINT('Ctrl Pts',(-41.3750598134236,44.6966738638162,0.205540216848794));
#41004=CARTESIAN_POINT('Ctrl Pts',(-44.5303430016157,41.4202123648473,0.00967765904350021));
#41005=CARTESIAN_POINT('Ctrl Pts',(-49.0001600008312,42.2448663028631,-0.186184898761794));
#41006=CARTESIAN_POINT('Ctrl Pts',(-50.7887546377267,46.4200984444482,-0.382047456567086));
#41007=CARTESIAN_POINT('Ctrl Pts',(-48.2991248954935,50.2221780497669,-0.577910014372381));
#41008=CARTESIAN_POINT('Ctrl Pts',(-43.7551468972239,50.2508324710758,-0.773772572177673));
#41009=CARTESIAN_POINT('Ctrl Pts',(-41.216941413185,46.4820553508686,-0.969635129982968));
#41010=CARTESIAN_POINT('Ctrl Pts',(-42.9521748839983,42.2823237877054,-1.16549768778826));
#41011=CARTESIAN_POINT('Ctrl Pts',(-47.4105428653624,41.4043187587238,-1.36136024559355));
#41012=CARTESIAN_POINT('Ctrl Pts',(-50.6086352711288,44.632317129114,-1.55722280339885));
#41013=CARTESIAN_POINT('Ctrl Pts',(-49.6890936551595,49.0823177128668,-1.75308536120414));
#41014=CARTESIAN_POINT('Ctrl Pts',(-45.4734861227781,50.7783710029823,-1.94894791900944));
#41015=CARTESIAN_POINT('Ctrl Pts',(-41.7282996653196,48.2051403801394,-2.14481047681473));
#41016=CARTESIAN_POINT('Ctrl Pts',(-41.7997129669298,43.6616979327745,-2.34067303462002));
#41017=CARTESIAN_POINT('Ctrl Pts',(-45.6239218081334,41.2074403684165,-2.53653559242531));
#41018=CARTESIAN_POINT('Ctrl Pts',(-49.784141948293,43.0351500661756,-2.73239815023061));
#41019=CARTESIAN_POINT('Ctrl Pts',(-50.5633765475329,47.511839809745,-2.9282607080359));
#41020=CARTESIAN_POINT('Ctrl Pts',(-47.2654092996424,50.6377585015902,-3.1241232658412));
#41021=CARTESIAN_POINT('Ctrl Pts',(-42.8368474210137,49.6200180555421,-3.31998582364649));
#41022=CARTESIAN_POINT('Ctrl Pts',(-41.2344409709606,45.3679303548353,-3.51584838145178));
#41023=CARTESIAN_POINT('Ctrl Pts',(-43.8898786280806,41.6805726486878,-3.71171093925708));
#41024=CARTESIAN_POINT('Ctrl Pts',(-48.430628748381,41.8524575015287,-3.90757349706237));
#41025=CARTESIAN_POINT('Ctrl Pts',(-50.7997053640471,45.7300124112724,-4.10343605486767));
#41026=CARTESIAN_POINT('Ctrl Pts',(-48.8804294354025,49.848790867101,-4.29929861267296));
#41027=CARTESIAN_POINT('Ctrl Pts',(-44.3876003506517,50.5288223911423,-4.49516117047825));
#41028=CARTESIAN_POINT('Ctrl Pts',(-41.3353884704811,47.1625249105979,-4.69102372828355));
#41029=CARTESIAN_POINT('Ctrl Pts',(-42.4508279821942,42.7575560397258,-4.88688628608884));
#41030=CARTESIAN_POINT('Ctrl Pts',(-46.7373164737192,41.2495864060927,-5.08274884389414));
#41031=CARTESIAN_POINT('Ctrl Pts',(-50.3650410138277,43.9859290211115,-5.27861140169942));
#41032=CARTESIAN_POINT('Ctrl Pts',(-50.0927688821017,48.5217667402822,-5.47447395950472));
#41033=CARTESIAN_POINT('Ctrl Pts',(-46.1637649138928,50.8045026982905,-5.67033651731001));
#41034=CARTESIAN_POINT('Ctrl Pts',(-42.0884430951448,48.7945997915639,-5.86619907511531));
#41035=CARTESIAN_POINT('Ctrl Pts',(-41.507947633761,44.2878293987898,-6.0620616329206));
#41036=CARTESIAN_POINT('Ctrl Pts',(-44.940927797173,41.3108173647246,-6.25792419072589));
#41037=CARTESIAN_POINT('Ctrl Pts',(-49.3201499067242,42.5234108033435,-6.45378674853119));
#41038=CARTESIAN_POINT('Ctrl Pts',(-50.7329422698335,46.8422017427392,-6.64964930633648));
#41039=CARTESIAN_POINT('Ctrl Pts',(-47.9170389384488,50.4085208617021,-6.84551186414178));
#41040=CARTESIAN_POINT('Ctrl Pts',(-43.3883214271118,50.0359894114731,-7.04137442194707));
#41041=CARTESIAN_POINT('Ctrl Pts',(-41.1930659955112,46.0574693216547,-7.23723697975236));
#41042=CARTESIAN_POINT('Ctrl Pts',(-43.2925654154187,42.0275760136403,-7.43309953755766));
#41043=CARTESIAN_POINT('Ctrl Pts',(-47.8111685874939,41.5469454131034,-7.62896209536294));
#41044=CARTESIAN_POINT('Ctrl Pts',(-50.7113274270403,45.0448371733502,-7.82482465316825));
#41045=CARTESIAN_POINT('Ctrl Pts',(-49.4025756475167,49.3963571266783,-8.02068721097353));
#41046=CARTESIAN_POINT('Ctrl Pts',(-45.0527729214423,50.7128987412233,-8.21654976877883));
#41047=CARTESIAN_POINT('Ctrl Pts',(-41.5512846772643,47.8195936610183,-8.41241232658412));
#41048=CARTESIAN_POINT('Ctrl Pts',(-42.0204412135141,43.2986191788456,-8.60827488438942));
#41049=CARTESIAN_POINT('Ctrl Pts',(-46.0536470456105,41.195226046819,-8.80413744219471));
#41050=CARTESIAN_POINT('Ctrl Pts',(-48.6953045558515,42.6504167892078,-8.93471248073157));
#41051=CARTESIAN_POINT('Ctrl Pts',(-49.4256147683784,43.7746037524369,-9.));
#41052=CARTESIAN_POINT('Ctrl Pts',(-43.4267655729853,48.2065515280923,0.));
#41053=CARTESIAN_POINT('Ctrl Pts',(-43.350127485791,48.1336147263286,-7.04754888835137E-18));
#41054=CARTESIAN_POINT('Ctrl Pts',(-43.2774221639843,48.0570418002056,-2.0037929668525E-16));
#41055=CARTESIAN_POINT('Ctrl Pts',(-43.2086471182341,47.9772483225893,-1.80411241501588E-16));
#41056=CARTESIAN_POINT('Ctrl Pts',(-43.1381549137597,47.8954625807044,-1.59944628740986E-16));
#41057=CARTESIAN_POINT('Ctrl Pts',(-43.0717912973076,47.8102930504676,-2.80029045420587E-16));
#41058=CARTESIAN_POINT('Ctrl Pts',(-43.0095797390392,47.722138908728,-3.05311331771918E-16));
#41059=CARTESIAN_POINT('Ctrl Pts',(-42.9460526993407,47.632120722112,-3.31128219395583E-16));
#41060=CARTESIAN_POINT('Ctrl Pts',(-42.8868547189701,47.5389898301017,-7.05663083191702E-16));
#41061=CARTESIAN_POINT('Ctrl Pts',(-42.8320442088995,47.443128838907,-7.21644966006352E-16));
#41062=CARTESIAN_POINT('Ctrl Pts',(-42.7793833374229,47.3510274639989,-7.37000048011074E-16));
#41063=CARTESIAN_POINT('Ctrl Pts',(-42.7307724565797,47.256405116335,-2.18211742452875E-16));
#41064=CARTESIAN_POINT('Ctrl Pts',(-42.6862972115001,47.1595729951209,-1.2490009027033E-16));
#41065=CARTESIAN_POINT('Ctrl Pts',(-42.6798840800015,47.1456102361632,-1.11444967207507E-16));
#41066=CARTESIAN_POINT('Ctrl Pts',(-42.6735569988815,47.1316014931762,-5.23608940400973E-16));
#41067=CARTESIAN_POINT('Ctrl Pts',(-42.6673162875643,47.1175476635147,-5.27355936696949E-16));
#41068=CARTESIAN_POINT('Ctrl Pts',(-42.6607661644965,47.102797051096,-5.31288707438301E-16));
#41069=CARTESIAN_POINT('Ctrl Pts',(-42.6543147503395,47.0880047578612,7.95783905053014E-17));
#41070=CARTESIAN_POINT('Ctrl Pts',(-42.6479633745278,47.0731750014718,6.93889390390723E-17));
#41071=CARTESIAN_POINT('Ctrl Pts',(-42.6031057839847,46.9684375147142,-2.57566442362801E-18));
#41072=CARTESIAN_POINT('Ctrl Pts',(-42.5632143269563,46.8617873344586,-4.68138119745799E-16));
#41073=CARTESIAN_POINT('Ctrl Pts',(-42.5283181388421,46.7536539294655,-3.60822483003176E-16));
#41074=CARTESIAN_POINT('Ctrl Pts',(-42.4929004096067,46.643904416229,-2.51902959975767E-16));
#41075=CARTESIAN_POINT('Ctrl Pts',(-42.4626279321656,46.5326263002381,-1.62036195599726E-16));
#41076=CARTESIAN_POINT('Ctrl Pts',(-42.4375708467752,46.4202321196064,-2.08166817117217E-16));
#41077=CARTESIAN_POINT('Ctrl Pts',(-42.4112941893324,46.302367518157,-2.56542696448442E-16));
#41078=CARTESIAN_POINT('Ctrl Pts',(-42.3907521119287,46.183274805057,1.09214840709062E-16));
#41079=CARTESIAN_POINT('Ctrl Pts',(-42.3760792116234,46.0634010904814,1.38777878078145E-16));
#41080=CARTESIAN_POINT('Ctrl Pts',(-42.3650745363945,45.9734958045497,1.60950156104956E-16));
#41081=CARTESIAN_POINT('Ctrl Pts',(-42.3573723501925,45.8831504952769,2.7624515033776E-16));
#41082=CARTESIAN_POINT('Ctrl Pts',(-42.3530521456739,45.7925483464972,4.16333634234434E-16));
#41083=CARTESIAN_POINT('Ctrl Pts',(-42.3520987176639,45.7725533147698,4.47249829025506E-16));
#41084=CARTESIAN_POINT('Ctrl Pts',(-42.3513101054994,45.7525434126973,-6.43493868513383E-16));
#41085=CARTESIAN_POINT('Ctrl Pts',(-42.3506877635742,45.7325443531856,-6.38378239159465E-16));
#41086=CARTESIAN_POINT('Ctrl Pts',(-42.3469997598448,45.6140297503959,-6.08062974556997E-16));
#41087=CARTESIAN_POINT('Ctrl Pts',(-42.3491369571258,45.495720031201,-1.89016809378538E-16));
#41088=CARTESIAN_POINT('Ctrl Pts',(-42.3571653633738,45.3780427848328,-1.94289029309402E-16));
#41089=CARTESIAN_POINT('Ctrl Pts',(-42.365167844959,45.2607455320572,-1.99544224625444E-16));
#41090=CARTESIAN_POINT('Ctrl Pts',(-42.3790232255707,45.1440757899907,5.28835535732368E-17));
#41091=CARTESIAN_POINT('Ctrl Pts',(-42.3988451111656,45.0284394788713,5.55111512312578E-17));
#41092=CARTESIAN_POINT('Ctrl Pts',(-42.4013982106115,45.0135452852572,5.58495911890846E-17));
#41093=CARTESIAN_POINT('Ctrl Pts',(-42.4040503639055,44.9986682229785,-4.58137967173707E-16));
#41094=CARTESIAN_POINT('Ctrl Pts',(-42.4068018766013,44.9838091499857,-4.71844785465692E-16));
#41095=CARTESIAN_POINT('Ctrl Pts',(-42.4276948097905,44.8709804431543,-6.0624956633226E-16));
#41096=CARTESIAN_POINT('Ctrl Pts',(-42.4543121735532,44.7591887131703,-8.63511011112326E-16));
#41097=CARTESIAN_POINT('Ctrl Pts',(-42.4863557082657,44.6486957988342,-9.71445146547012E-16));
#41098=CARTESIAN_POINT('Ctrl Pts',(-42.5065653594726,44.5790086285643,-1.03951851142446E-15));
#41099=CARTESIAN_POINT('Ctrl Pts',(-42.528934495595,44.509838105819,-9.38420932093488E-16));
#41100=CARTESIAN_POINT('Ctrl Pts',(-42.5533986678225,44.441251448601,-9.99200722162641E-16));
#41101=CARTESIAN_POINT('Ctrl Pts',(-42.5620407794544,44.4170228116121,-1.02067153776408E-15));
#41102=CARTESIAN_POINT('Ctrl Pts',(-42.5709443994809,44.3928670518755,-3.880055035361E-16));
#41103=CARTESIAN_POINT('Ctrl Pts',(-42.5801069098143,44.3687871960285,-3.88578058618805E-16));
#41104=CARTESIAN_POINT('Ctrl Pts',(-42.5859810783122,44.3533493819905,-3.88945128876595E-16));
#41105=CARTESIAN_POINT('Ctrl Pts',(-42.5919602903931,44.3379464816701,-9.54382670255255E-18));
#41106=CARTESIAN_POINT('Ctrl Pts',(-42.5980400731475,44.3225881416726,0.));
#41107=CARTESIAN_POINT('Ctrl Pts',(-42.6409152181459,44.2142798219628,6.73038774974722E-17));
#41108=CARTESIAN_POINT('Ctrl Pts',(-42.6888373119785,44.1080564604858,-3.4716028785113E-16));
#41109=CARTESIAN_POINT('Ctrl Pts',(-42.741452191163,44.0041741405836,-3.88578058618805E-16));
#41110=CARTESIAN_POINT('Ctrl Pts',(-42.7959112494356,43.8966506909297,-4.31447543956746E-16));
#41111=CARTESIAN_POINT('Ctrl Pts',(-42.8553979439767,43.791634588613,-3.1798967153709E-16));
#41112=CARTESIAN_POINT('Ctrl Pts',(-42.9195754661052,43.6894132096538,-5.55111512312578E-16));
#41113=CARTESIAN_POINT('Ctrl Pts',(-42.9844485692458,43.5860839155262,-7.94803372069007E-16));
#41114=CARTESIAN_POINT('Ctrl Pts',(-43.0541151127463,43.4856094929693,-7.88000339611239E-16));
#41115=CARTESIAN_POINT('Ctrl Pts',(-43.1282792501117,43.3883012080013,-7.21644966006352E-16));
#41116=CARTESIAN_POINT('Ctrl Pts',(-43.1809780311253,43.3191568994108,-6.74494855091483E-16));
#41117=CARTESIAN_POINT('Ctrl Pts',(-43.2359487941652,43.2516114776716,-8.53408132386238E-17));
#41118=CARTESIAN_POINT('Ctrl Pts',(-43.2930994306075,43.1857842411025,-5.55111512312578E-17));
#41119=CARTESIAN_POINT('Ctrl Pts',(-43.3103646730886,43.1658977923772,-4.64995919600553E-17));
#41120=CARTESIAN_POINT('Ctrl Pts',(-43.327828935708,43.1461682069428,-1.02592134112036E-16));
#41121=CARTESIAN_POINT('Ctrl Pts',(-43.345489866523,43.1265989222763,-1.11022302462516E-16));
#41122=CARTESIAN_POINT('Ctrl Pts',(-43.3628751859287,43.1073350302407,-1.19320912029112E-16));
#41123=CARTESIAN_POINT('Ctrl Pts',(-43.3804547805861,43.0882226751835,2.41217254613375E-16));
#41124=CARTESIAN_POINT('Ctrl Pts',(-43.3982046967558,43.0692880183209,2.22044604925031E-16));
#41125=CARTESIAN_POINT('Ctrl Pts',(-43.4838647831345,42.9779104407086,1.295184874654E-16));
#41126=CARTESIAN_POINT('Ctrl Pts',(-43.5735667660932,42.8905787756105,1.54127168466576E-16));
#41127=CARTESIAN_POINT('Ctrl Pts',(-43.6669813080034,42.8076092595666,-1.11022302462516E-16));
#41128=CARTESIAN_POINT('Ctrl Pts',(-43.7477793817384,42.7358455176695,-3.40360969278814E-16));
#41129=CARTESIAN_POINT('Ctrl Pts',(-43.8313559162862,42.6673451480848,-3.95274884398571E-16));
#41130=CARTESIAN_POINT('Ctrl Pts',(-43.9175245054789,42.602328677346,-1.66533453693773E-16));
#41131=CARTESIAN_POINT('Ctrl Pts',(-43.9569254786932,42.5725996049999,-6.19404103510884E-17));
#41132=CARTESIAN_POINT('Ctrl Pts',(-43.9968687187229,42.5435991930232,-9.45628619310071E-17));
#41133=CARTESIAN_POINT('Ctrl Pts',(-44.0373378970811,42.5153498982221,-5.55111512312578E-17));
#41134=CARTESIAN_POINT('Ctrl Pts',(-44.0558572039848,42.5024225944947,-3.76404989249141E-17));
#41135=CARTESIAN_POINT('Ctrl Pts',(-44.074488606412,42.4896512907743,7.87308458251505E-18));
#41136=CARTESIAN_POINT('Ctrl Pts',(-44.0932243068781,42.4770424318878,0.));
#41137=CARTESIAN_POINT('Ctrl Pts',(-44.1981797728502,42.4064089019487,-4.41042096338891E-17));
#41138=CARTESIAN_POINT('Ctrl Pts',(-44.3062422429739,42.3409785193577,4.59490679880944E-16));
#41139=CARTESIAN_POINT('Ctrl Pts',(-44.4171006494925,42.2810834907564,4.44089209850063E-16));
#41140=CARTESIAN_POINT('Ctrl Pts',(-44.5269323221333,42.2217431900906,4.28830383138215E-16));
#41141=CARTESIAN_POINT('Ctrl Pts',(-44.6395089620466,42.1678354863558,-2.86547826934204E-16));
#41142=CARTESIAN_POINT('Ctrl Pts',(-44.7545634922447,42.1197193691043,-2.22044604925031E-16));
#41143=CARTESIAN_POINT('Ctrl Pts',(-44.815479257569,42.0942442304743,-1.87893293127013E-16));
#41144=CARTESIAN_POINT('Ctrl Pts',(-44.8770901666956,42.0703932494507,-2.5515543336404E-16));
#41145=CARTESIAN_POINT('Ctrl Pts',(-44.9393361356002,42.0481502636203,-2.77555756156289E-16));
#41146=CARTESIAN_POINT('Ctrl Pts',(-49.387979831519,45.997252452837,-2.01601780324957));
#41147=CARTESIAN_POINT('Ctrl Pts',(-49.3905746620075,45.6709119723256,-1.99688706151736));
#41148=CARTESIAN_POINT('Ctrl Pts',(-49.347131989526,45.3452478557311,-1.97775631978515));
#41149=CARTESIAN_POINT('Ctrl Pts',(-49.2547930859516,45.0340948157173,-1.95862557805294));
#41150=CARTESIAN_POINT('Ctrl Pts',(-48.9396679313325,43.9722222349419,-1.8933380587845));
#41151=CARTESIAN_POINT('Ctrl Pts',(-48.0550711355392,43.0793534078484,-1.82805053951607));
#41152=CARTESIAN_POINT('Ctrl Pts',(-46.9961773535207,42.7543476987893,-1.76276302024764));
#41153=CARTESIAN_POINT('Ctrl Pts',(-45.9372835715021,42.4293419897301,-1.69747550097921));
#41154=CARTESIAN_POINT('Ctrl Pts',(-44.7040928032581,42.6721993987052,-1.63218798171078));
#41155=CARTESIAN_POINT('Ctrl Pts',(-43.8475134265744,43.3744538912888,-1.56690046244235));
#41156=CARTESIAN_POINT('Ctrl Pts',(-42.9909340498907,44.0767083838724,-1.50161294317392));
#41157=CARTESIAN_POINT('Ctrl Pts',(-42.5109660647671,45.2383599600643,-1.43632542390549));
#41158=CARTESIAN_POINT('Ctrl Pts',(-42.6220176511331,46.3404102378879,-1.37103790463705));
#41159=CARTESIAN_POINT('Ctrl Pts',(-42.7330692374992,47.4424605157114,-1.30575038536862));
#41160=CARTESIAN_POINT('Ctrl Pts',(-43.4351403953548,48.4849094951665,-1.24046286610019));
#41161=CARTESIAN_POINT('Ctrl Pts',(-44.4146112831213,49.0021710585525,-1.17517534683176));
#41162=CARTESIAN_POINT('Ctrl Pts',(-45.3940821708877,49.5194326219384,-1.10988782756333));
#41163=CARTESIAN_POINT('Ctrl Pts',(-46.6509527885649,49.5115067692553,-1.0446003082949));
#41164=CARTESIAN_POINT('Ctrl Pts',(-47.6237056175478,48.9817135963969,-0.979312789026467));
#41165=CARTESIAN_POINT('Ctrl Pts',(-48.5964584465306,48.4519204235384,-0.914025269758036));
#41166=CARTESIAN_POINT('Ctrl Pts',(-49.2850934868191,47.4002599305046,-0.848737750489605));
#41167=CARTESIAN_POINT('Ctrl Pts',(-49.3820471281213,46.2969921828887,-0.783450231221174));
#41168=CARTESIAN_POINT('Ctrl Pts',(-49.3906763290647,46.198797633817,-0.777639421897305));
#41169=CARTESIAN_POINT('Ctrl Pts',(-49.3946184665688,46.1001942727114,-0.771828612573436));
#41170=CARTESIAN_POINT('Ctrl Pts',(-49.3940292623548,46.0015451960205,-0.766017803249567));
#41171=CARTESIAN_POINT('Ctrl Pts',(-47.0579044229729,42.0543614925016,5.55111512312578E-16));
#41172=CARTESIAN_POINT('Ctrl Pts',(-48.3527480267224,42.4015349025495,-0.0652875192684306));
#41173=CARTESIAN_POINT('Ctrl Pts',(-50.5530316149402,44.4642359903368,-0.195862557805293));
#41174=CARTESIAN_POINT('Ctrl Pts',(-49.7989189441901,48.9500085119455,-0.391725115610587));
#41175=CARTESIAN_POINT('Ctrl Pts',(-45.6441921094362,50.7932694144525,-0.587587673415879));
#41176=CARTESIAN_POINT('Ctrl Pts',(-41.8104748163565,48.3572313450219,-0.783450231221174));
#41177=CARTESIAN_POINT('Ctrl Pts',(-41.7184176569125,43.8134905867626,-0.979312789026467));
#41178=CARTESIAN_POINT('Ctrl Pts',(-45.4525333012251,41.2240979371497,-1.17517534683176));
#41179=CARTESIAN_POINT('Ctrl Pts',(-49.6754258594775,42.9014061288129,-1.37103790463705));
#41180=CARTESIAN_POINT('Ctrl Pts',(-50.6146443015424,47.3473770364547,-1.56690046244235));
#41181=CARTESIAN_POINT('Ctrl Pts',(-47.4307681707597,50.5894263088653,-1.76276302024764));
#41182=CARTESIAN_POINT('Ctrl Pts',(-42.968598137007,49.7310442859955,-1.95862557805294));
#41183=CARTESIAN_POINT('Ctrl Pts',(-41.2148485187469,45.539095378305,-2.15448813585823));
#41184=CARTESIAN_POINT('Ctrl Pts',(-43.7364582880855,41.758957824139,-2.35035069366352));
#41185=CARTESIAN_POINT('Ctrl Pts',(-48.2804507290339,41.7680234302945,-2.54621325146882));
#41186=CARTESIAN_POINT('Ctrl Pts',(-50.7869503966815,45.5582002648003,-2.74207580927411));
#41187=CARTESIAN_POINT('Ctrl Pts',(-49.0164924035275,49.7431069481348,-2.9379383670794));
#41188=CARTESIAN_POINT('Ctrl Pts',(-44.5509147952652,50.5836918395513,-3.13380092488469));
#41189=CARTESIAN_POINT('Ctrl Pts',(-41.380038920474,47.3289236804855,-3.32966348268999));
#41190=CARTESIAN_POINT('Ctrl Pts',(-42.3369211082577,42.8868133607463,-3.52552604049528));
#41191=CARTESIAN_POINT('Ctrl Pts',(-46.5666236386886,41.2262157555308,-3.72138859830058));
#41192=CARTESIAN_POINT('Ctrl Pts',(-50.2900697268067,43.8308112032815,-3.91725115610587));
#41193=CARTESIAN_POINT('Ctrl Pts',(-50.1805031387222,48.3734935761537,-4.11311371391116));
#41194=CARTESIAN_POINT('Ctrl Pts',(-46.3358174405565,50.7955505353102,-4.30897627171646));
#41195=CARTESIAN_POINT('Ctrl Pts',(-42.1910917427793,48.9329671271487,-4.50483882952175));
#41196=CARTESIAN_POINT('Ctrl Pts',(-41.4494793999576,44.4498901520179,-4.70070138732704));
#41197=CARTESIAN_POINT('Ctrl Pts',(-44.7735825745146,41.351776836325,-4.89656394513234));
#41198=CARTESIAN_POINT('Ctrl Pts',(-49.1934426554123,42.406672531387,-5.09242650293763));
#41199=CARTESIAN_POINT('Ctrl Pts',(-50.7600842734221,46.6720684182653,-5.28828906074293));
#41200=CARTESIAN_POINT('Ctrl Pts',(-48.0737732836718,50.3369969638681,-5.48415161854822));
#41201=CARTESIAN_POINT('Ctrl Pts',(-43.5346254271756,50.1269851679324,-5.68001417635351));
#41202=CARTESIAN_POINT('Ctrl Pts',(-41.19819518517,46.2296704992633,-5.87587673415881));
#41203=CARTESIAN_POINT('Ctrl Pts',(-43.1519931670912,42.1271540690863,-6.07173929196409));
#41204=CARTESIAN_POINT('Ctrl Pts',(-47.650376155957,41.4848768173615,-6.2676018497694));
#41205=CARTESIAN_POINT('Ctrl Pts',(-50.6742109766474,44.8766889159707,-6.46346440757468));
#41206=CARTESIAN_POINT('Ctrl Pts',(-49.5218185107369,49.2721362263424,-6.65932696537998));
#41207=CARTESIAN_POINT('Ctrl Pts',(-45.2228146507001,50.7440556643996,-6.85518952318527));
#41208=CARTESIAN_POINT('Ctrl Pts',(-41.6181995750799,47.9773428774946,-7.05105208099057));
#41209=CARTESIAN_POINT('Ctrl Pts',(-41.9285478600743,43.4439512443748,-7.24691463879586));
#41210=CARTESIAN_POINT('Ctrl Pts',(-45.8765970139655,41.1942887704259,-7.44277719660115));
#41211=CARTESIAN_POINT('Ctrl Pts',(-49.934872084144,43.2383495723774,-7.63863975440645));
#41212=CARTESIAN_POINT('Ctrl Pts',(-50.4775511169527,47.7498293925976,-7.83450231221174));
#41213=CARTESIAN_POINT('Ctrl Pts',(-47.0195850264259,50.6979235414129,-8.03036487001704));
#41214=CARTESIAN_POINT('Ctrl Pts',(-42.6509144693004,49.448562948282,-8.22622742782232));
#41215=CARTESIAN_POINT('Ctrl Pts',(-41.274000700432,45.1181262021708,-8.42208998562762));
#41216=CARTESIAN_POINT('Ctrl Pts',(-44.1206543946181,41.5754411548869,-8.61795254343291));
#41217=CARTESIAN_POINT('Ctrl Pts',(-48.6442465086048,41.9862746311881,-8.81381510123821));
#41218=CARTESIAN_POINT('Ctrl Pts',(-50.8097847232332,45.9824991077558,-9.0096776590435));
#41219=CARTESIAN_POINT('Ctrl Pts',(-48.6687289051654,49.9958170642257,-9.2055402168488));
#41220=CARTESIAN_POINT('Ctrl Pts',(-45.6668068080595,50.2864153592086,-9.33611525538566));
#41221=CARTESIAN_POINT('Ctrl Pts',(-44.4292895827202,49.7709539622022,-9.40140277465409));
#41222=CARTESIAN_POINT('Ctrl Pts',(-46.9978874462229,42.2782052438144,0.133800924884696));
#41223=CARTESIAN_POINT('Ctrl Pts',(-48.219272052379,42.6056828306607,0.0685134056162651));
#41224=CARTESIAN_POINT('Ctrl Pts',(-50.2947292705676,44.5513628714236,-0.062061632920597));
#41225=CARTESIAN_POINT('Ctrl Pts',(-49.5833988792412,48.7826487879202,-0.257924190725891));
#41226=CARTESIAN_POINT('Ctrl Pts',(-45.6643777835214,50.521337912176,-0.453786748531184));
#41227=CARTESIAN_POINT('Ctrl Pts',(-42.0481547334457,48.2235010233062,-0.649649306336478));
#41228=CARTESIAN_POINT('Ctrl Pts',(-41.9613201558135,43.9375355210387,-0.845511864141771));
#41229=CARTESIAN_POINT('Ctrl Pts',(-45.4835921524958,41.4950441557703,-1.04137442194707));
#41230=CARTESIAN_POINT('Ctrl Pts',(-49.4669117975598,43.0771953894366,-1.23723697975236));
#41231=CARTESIAN_POINT('Ctrl Pts',(-50.3528465495515,47.2709377149863,-1.43309953755765));
#41232=CARTESIAN_POINT('Ctrl Pts',(-47.349597907951,50.3290592226769,-1.62896209536294));
#41233=CARTESIAN_POINT('Ctrl Pts',(-43.1405754642404,49.5193748824999,-1.82482465316824));
#41234=CARTESIAN_POINT('Ctrl Pts',(-41.4863194748743,45.5652433944807,-2.02068721097353));
#41235=CARTESIAN_POINT('Ctrl Pts',(-43.8648734145815,41.9995604004562,-2.21654976877883));
#41236=CARTESIAN_POINT('Ctrl Pts',(-48.1510763210893,42.0081116971315,-2.41241232658412));
#41237=CARTESIAN_POINT('Ctrl Pts',(-50.5153773845809,45.5832644235843,-2.60827488438941));
#41238=CARTESIAN_POINT('Ctrl Pts',(-48.8453609189455,49.5307532063404,-2.80413744219471));
#41239=CARTESIAN_POINT('Ctrl Pts',(-44.6331242190589,50.3236500809672,-3.));
#41240=CARTESIAN_POINT('Ctrl Pts',(-41.642138303627,47.2535312538142,-3.19586255780529));
#41241=CARTESIAN_POINT('Ctrl Pts',(-42.5447347026668,43.063430497502,-3.39172511561059));
#41242=CARTESIAN_POINT('Ctrl Pts',(-46.5344779769343,41.4970418261931,-3.58758767341588));
#41243=CARTESIAN_POINT('Ctrl Pts',(-50.0466857221096,43.9538735052741,-3.78345023122118));
#41244=CARTESIAN_POINT('Ctrl Pts',(-49.9433350597996,48.2388406664172,-3.97931278902647));
#41245=CARTESIAN_POINT('Ctrl Pts',(-46.3167658636045,50.523489620608,-4.17517534683176));
#41246=CARTESIAN_POINT('Ctrl Pts',(-42.407178520897,48.7665741940479,-4.37103790463706));
#41247=CARTESIAN_POINT('Ctrl Pts',(-41.7076392895683,44.5378309004316,-4.56690046244235));
#41248=CARTESIAN_POINT('Ctrl Pts',(-44.8431596218478,41.6154795825139,-4.76276302024764));
#41249=CARTESIAN_POINT('Ctrl Pts',(-49.0122724386701,42.6105289918156,-4.95862557805293));
#41250=CARTESIAN_POINT('Ctrl Pts',(-50.4900354287793,46.6339406689548,-5.15448813585823));
#41251=CARTESIAN_POINT('Ctrl Pts',(-47.9561240894267,50.0909506856854,-5.35035069366352));
#41252=CARTESIAN_POINT('Ctrl Pts',(-43.6744909246669,49.8928532676464,-5.54621325146882));
#41253=CARTESIAN_POINT('Ctrl Pts',(-41.470610917321,46.2166408448682,-5.74207580927411));
#41254=CARTESIAN_POINT('Ctrl Pts',(-43.3135661373547,42.3468681558645,-5.9379383670794));
#41255=CARTESIAN_POINT('Ctrl Pts',(-47.5567471047592,41.7410285425945,-6.13380092488469));
#41256=CARTESIAN_POINT('Ctrl Pts',(-50.4090338912526,44.9404165398932,-6.32966348268999));
#41257=CARTESIAN_POINT('Ctrl Pts',(-49.3220188926554,49.0865015701723,-6.52552604049528));
#41258=CARTESIAN_POINT('Ctrl Pts',(-45.2669058880808,50.4749161539406,-6.72138859830057));
#41259=CARTESIAN_POINT('Ctrl Pts',(-41.8667876408021,47.8651643678596,-6.91725115610587));
#41260=CARTESIAN_POINT('Ctrl Pts',(-42.1595292636062,43.5889608647215,-7.11311371391116));
#41261=CARTESIAN_POINT('Ctrl Pts',(-45.8835979055232,41.4669261210878,-7.30897627171646));
#41262=CARTESIAN_POINT('Ctrl Pts',(-49.7116391329811,43.395023375707,-7.50483882952176));
#41263=CARTESIAN_POINT('Ctrl Pts',(-50.2235309281268,47.6505581657348,-7.70070138732704));
#41264=CARTESIAN_POINT('Ctrl Pts',(-46.961741983617,50.4314011960709,-7.89656394513235));
#41265=CARTESIAN_POINT('Ctrl Pts',(-42.8409146092611,49.2529192608244,-8.09242650293762));
#41266=CARTESIAN_POINT('Ctrl Pts',(-41.5421158381738,45.1681566189754,-8.28828906074293));
#41267=CARTESIAN_POINT('Ctrl Pts',(-44.2272733282894,41.8264549890007,-8.48415161854821));
#41268=CARTESIAN_POINT('Ctrl Pts',(-48.4942332580861,42.2139810826501,-8.68001417635352));
#41269=CARTESIAN_POINT('Ctrl Pts',(-50.5369162753484,45.9834919674321,-8.8758767341588));
#41270=CARTESIAN_POINT('Ctrl Pts',(-48.5173267206434,49.769126585735,-9.0717392919641));
#41271=CARTESIAN_POINT('Ctrl Pts',(-45.6857095062803,50.0432386738974,-9.20231433050096));
#41272=CARTESIAN_POINT('Ctrl Pts',(-44.5183990415218,49.5570204051054,-9.26760184976939));
#41273=CARTESIAN_POINT('Ctrl Pts',(-46.9378704694728,42.5020489951272,0.267601849769392));
#41274=CARTESIAN_POINT('Ctrl Pts',(-48.0857960780355,42.8098307587719,0.202314330500961));
#41275=CARTESIAN_POINT('Ctrl Pts',(-50.0364269261949,44.6384897525104,0.0717392919640985));
#41276=CARTESIAN_POINT('Ctrl Pts',(-49.3678788142924,48.6152890638949,-0.124123265841195));
#41277=CARTESIAN_POINT('Ctrl Pts',(-45.6845634576067,50.2494064098995,-0.319985823646489));
#41278=CARTESIAN_POINT('Ctrl Pts',(-42.2858346505349,48.0897707015904,-0.515848381451782));
#41279=CARTESIAN_POINT('Ctrl Pts',(-42.2042226547145,44.0615804553148,-0.711710939257076));
#41280=CARTESIAN_POINT('Ctrl Pts',(-45.5146510037666,41.765990374391,-0.907573497062369));
#41281=CARTESIAN_POINT('Ctrl Pts',(-49.2583977356421,43.2529846500602,-1.10343605486766));
#41282=CARTESIAN_POINT('Ctrl Pts',(-50.0910487975607,47.194498393518,-1.29929861267296));
#41283=CARTESIAN_POINT('Ctrl Pts',(-47.2684276451423,50.0686921364886,-1.49516117047825));
#41284=CARTESIAN_POINT('Ctrl Pts',(-43.3125527914738,49.3077054790043,-1.69102372828354));
#41285=CARTESIAN_POINT('Ctrl Pts',(-41.7577904310017,45.5913914106565,-1.88688628608883));
#41286=CARTESIAN_POINT('Ctrl Pts',(-43.9932885410775,42.2401629767734,-2.08274884389413));
#41287=CARTESIAN_POINT('Ctrl Pts',(-48.0217019131448,42.2481999639685,-2.27861140169942));
#41288=CARTESIAN_POINT('Ctrl Pts',(-50.2438043724803,45.6083285823682,-2.47447395950472));
#41289=CARTESIAN_POINT('Ctrl Pts',(-48.6742294343635,49.318399464546,-2.67033651731001));
#41290=CARTESIAN_POINT('Ctrl Pts',(-44.7153336428526,50.0636083223831,-2.8661990751153));
#41291=CARTESIAN_POINT('Ctrl Pts',(-41.9042376867801,47.1781388271428,-3.0620616329206));
#41292=CARTESIAN_POINT('Ctrl Pts',(-42.7525482970759,43.2400476342577,-3.25792419072589));
#41293=CARTESIAN_POINT('Ctrl Pts',(-46.5023323151801,41.7678678968555,-3.45378674853118));
#41294=CARTESIAN_POINT('Ctrl Pts',(-49.8033017174126,44.0769358072666,-3.64964930633648));
#41295=CARTESIAN_POINT('Ctrl Pts',(-49.706166980877,48.1041877566808,-3.84551186414177));
#41296=CARTESIAN_POINT('Ctrl Pts',(-46.2977142866525,50.2514287059059,-4.04137442194707));
#41297=CARTESIAN_POINT('Ctrl Pts',(-42.6232652990147,48.6001812609472,-4.23723697975236));
#41298=CARTESIAN_POINT('Ctrl Pts',(-41.965799179179,44.6257716488452,-4.43309953755766));
#41299=CARTESIAN_POINT('Ctrl Pts',(-44.912736669181,41.8791823287028,-4.62896209536295));
#41300=CARTESIAN_POINT('Ctrl Pts',(-48.8311022219279,42.8143854522443,-4.82482465316824));
#41301=CARTESIAN_POINT('Ctrl Pts',(-50.2199865841366,46.5958129196444,-5.02068721097354));
#41302=CARTESIAN_POINT('Ctrl Pts',(-47.8384748951817,49.8449044075027,-5.21654976877883));
#41303=CARTESIAN_POINT('Ctrl Pts',(-43.8143564221583,49.6587213673604,-5.41241232658412));
#41304=CARTESIAN_POINT('Ctrl Pts',(-41.743026649472,46.2036111904731,-5.60827488438941));
#41305=CARTESIAN_POINT('Ctrl Pts',(-43.4751391076183,42.5665822426429,-5.80413744219471));
#41306=CARTESIAN_POINT('Ctrl Pts',(-47.4631180535614,41.9971802678274,-6.));
#41307=CARTESIAN_POINT('Ctrl Pts',(-50.1438568058577,45.0041441638159,-6.1958625578053));
#41308=CARTESIAN_POINT('Ctrl Pts',(-49.1222192745738,48.9008669140022,-6.39172511561059));
#41309=CARTESIAN_POINT('Ctrl Pts',(-45.3109971254615,50.2057766434817,-6.58758767341588));
#41310=CARTESIAN_POINT('Ctrl Pts',(-42.1153757065243,47.7529858582244,-6.78345023122117));
#41311=CARTESIAN_POINT('Ctrl Pts',(-42.3905106671381,43.7339704850681,-6.97931278902647));
#41312=CARTESIAN_POINT('Ctrl Pts',(-45.890598797081,41.7395634717496,-7.17517534683176));
#41313=CARTESIAN_POINT('Ctrl Pts',(-49.4884061818182,43.5516971790367,-7.37103790463706));
#41314=CARTESIAN_POINT('Ctrl Pts',(-49.9695107393009,47.551286938872,-7.56690046244235));
#41315=CARTESIAN_POINT('Ctrl Pts',(-46.9038989408082,50.1648788507288,-7.76276302024764));
#41316=CARTESIAN_POINT('Ctrl Pts',(-43.0309147492218,49.0572755733668,-7.95862557805294));
#41317=CARTESIAN_POINT('Ctrl Pts',(-41.8102309759155,45.21818703578,-8.15448813585822));
#41318=CARTESIAN_POINT('Ctrl Pts',(-44.3338922619607,42.0774688231145,-8.35035069366353));
#41319=CARTESIAN_POINT('Ctrl Pts',(-48.3442200075673,42.4416875341121,-8.54621325146881));
#41320=CARTESIAN_POINT('Ctrl Pts',(-50.2640478274637,45.9844848271084,-8.74207580927412));
#41321=CARTESIAN_POINT('Ctrl Pts',(-48.3659245361215,49.5424361072444,-8.9379383670794));
#41322=CARTESIAN_POINT('Ctrl Pts',(-45.7046122045012,49.8000619885861,-9.06851340561627));
#41323=CARTESIAN_POINT('Ctrl Pts',(-44.6075085003234,49.3430868480087,-9.1338009248847));
#41324=CARTESIAN_POINT('Ctrl Pts',(-46.8778534927228,42.72589274644,0.401402774654088));
#41325=CARTESIAN_POINT('Ctrl Pts',(-47.9523201036921,43.0139786868831,0.336115255385657));
#41326=CARTESIAN_POINT('Ctrl Pts',(-49.7781245818222,44.7256166335971,0.205540216848794));
#41327=CARTESIAN_POINT('Ctrl Pts',(-49.1523587493435,48.4479293398696,0.00967765904350058));
#41328=CARTESIAN_POINT('Ctrl Pts',(-45.7047491316919,49.9774749076231,-0.186184898761793));
#41329=CARTESIAN_POINT('Ctrl Pts',(-42.5235145676241,47.9560403798747,-0.382047456567086));
#41330=CARTESIAN_POINT('Ctrl Pts',(-42.4471251536154,44.1856253895909,-0.57791001437238));
#41331=CARTESIAN_POINT('Ctrl Pts',(-45.5457098550374,42.0369365930118,-0.773772572177673));
#41332=CARTESIAN_POINT('Ctrl Pts',(-49.0498836737243,43.4287739106838,-0.969635129982967));
#41333=CARTESIAN_POINT('Ctrl Pts',(-49.82925104557,47.1180590720496,-1.16549768778826));
#41334=CARTESIAN_POINT('Ctrl Pts',(-47.1872573823336,49.8083250503002,-1.36136024559355));
#41335=CARTESIAN_POINT('Ctrl Pts',(-43.4845301187073,49.0960360755087,-1.55722280339885));
#41336=CARTESIAN_POINT('Ctrl Pts',(-42.0292613871291,45.6175394268322,-1.75308536120414));
#41337=CARTESIAN_POINT('Ctrl Pts',(-44.1217036675735,42.4807655530906,-1.94894791900944));
#41338=CARTESIAN_POINT('Ctrl Pts',(-47.8923275052001,42.4882882308056,-2.14481047681473));
#41339=CARTESIAN_POINT('Ctrl Pts',(-49.9722313603797,45.6333927411522,-2.34067303462002));
#41340=CARTESIAN_POINT('Ctrl Pts',(-48.5030979497815,49.1060457227516,-2.53653559242532));
#41341=CARTESIAN_POINT('Ctrl Pts',(-44.7975430666463,49.8035665637991,-2.73239815023061));
#41342=CARTESIAN_POINT('Ctrl Pts',(-42.1663370699331,47.1027464004715,-2.9282607080359));
#41343=CARTESIAN_POINT('Ctrl Pts',(-42.960361891485,43.4166647710134,-3.1241232658412));
#41344=CARTESIAN_POINT('Ctrl Pts',(-46.4701866534259,42.0386939675179,-3.31998582364649));
#41345=CARTESIAN_POINT('Ctrl Pts',(-49.5599177127155,44.1999981092592,-3.51584838145178));
#41346=CARTESIAN_POINT('Ctrl Pts',(-49.4689989019545,47.9695348469442,-3.71171093925708));
#41347=CARTESIAN_POINT('Ctrl Pts',(-46.2786627097004,49.9793677912038,-3.90757349706237));
#41348=CARTESIAN_POINT('Ctrl Pts',(-42.8393520771325,48.4337883278464,-4.10343605486766));
#41349=CARTESIAN_POINT('Ctrl Pts',(-42.2239590687897,44.7137123972589,-4.29929861267296));
#41350=CARTESIAN_POINT('Ctrl Pts',(-44.9823137165143,42.1428850748917,-4.49516117047826));
#41351=CARTESIAN_POINT('Ctrl Pts',(-48.6499320051857,43.018241912673,-4.69102372828354));
#41352=CARTESIAN_POINT('Ctrl Pts',(-49.9499377394939,46.557685170334,-4.88688628608884));
#41353=CARTESIAN_POINT('Ctrl Pts',(-47.7208257009366,49.59885812932,-5.08274884389413));
#41354=CARTESIAN_POINT('Ctrl Pts',(-43.9542219196496,49.4245894670743,-5.27861140169942));
#41355=CARTESIAN_POINT('Ctrl Pts',(-42.015442381623,46.1905815360779,-5.47447395950472));
#41356=CARTESIAN_POINT('Ctrl Pts',(-43.6367120778818,42.7862963294211,-5.67033651731001));
#41357=CARTESIAN_POINT('Ctrl Pts',(-47.3694890023636,42.2533319930603,-5.86619907511531));
#41358=CARTESIAN_POINT('Ctrl Pts',(-49.8786797204628,45.0678717877384,-6.06206163292059));
#41359=CARTESIAN_POINT('Ctrl Pts',(-48.9224196564922,48.7152322578321,-6.2579241907259));
#41360=CARTESIAN_POINT('Ctrl Pts',(-45.3550883628422,49.9366371330228,-6.45378674853118));
#41361=CARTESIAN_POINT('Ctrl Pts',(-42.3639637722466,47.6408073485894,-6.64964930633649));
#41362=CARTESIAN_POINT('Ctrl Pts',(-42.6214920706699,43.8789801054148,-6.84551186414177));
#41363=CARTESIAN_POINT('Ctrl Pts',(-45.8975996886388,42.0122008224115,-7.04137442194707));
#41364=CARTESIAN_POINT('Ctrl Pts',(-49.2651732306554,43.7083709823662,-7.23723697975236));
#41365=CARTESIAN_POINT('Ctrl Pts',(-49.715490550475,47.4520157120093,-7.43309953755766));
#41366=CARTESIAN_POINT('Ctrl Pts',(-46.8460558979993,49.8983565053867,-7.62896209536295));
#41367=CARTESIAN_POINT('Ctrl Pts',(-43.2209148891825,48.8616318859092,-7.82482465316825));
#41368=CARTESIAN_POINT('Ctrl Pts',(-42.0783461136572,45.2682174525847,-8.02068721097353));
#41369=CARTESIAN_POINT('Ctrl Pts',(-44.440511195632,42.3284826572283,-8.21654976877883));
#41370=CARTESIAN_POINT('Ctrl Pts',(-48.1942067570486,42.6693939855741,-8.41241232658413));
#41371=CARTESIAN_POINT('Ctrl Pts',(-49.9911793795789,45.9854776867847,-8.60827488438941));
#41372=CARTESIAN_POINT('Ctrl Pts',(-48.2145223515996,49.3157456287537,-8.8041374421947));
#41373=CARTESIAN_POINT('Ctrl Pts',(-45.723514902722,49.5568853032748,-8.93471248073157));
#41374=CARTESIAN_POINT('Ctrl Pts',(-44.696617959125,49.1291532909119,-9.));
#41375=CARTESIAN_POINT('Ctrl Pts',(-49.3881106776293,46.0027671006797,-1.10898219675043));
#41376=CARTESIAN_POINT('Ctrl Pts',(-49.3906991281383,46.3240935175671,-1.12782069376304));
#41377=CARTESIAN_POINT('Ctrl Pts',(-49.3485999788577,46.6447561566529,-1.14665919077565));
#41378=CARTESIAN_POINT('Ctrl Pts',(-49.2590242063896,46.9515558748637,-1.16549768778826));
#41379=CARTESIAN_POINT('Ctrl Pts',(-48.9485864911578,48.0148143981331,-1.23078520705669));
#41380=CARTESIAN_POINT('Ctrl Pts',(-48.0679219367457,48.9115697242166,-1.29607272632512));
#41381=CARTESIAN_POINT('Ctrl Pts',(-47.0104684489353,49.2412325581265,-1.36136024559355));
#41382=CARTESIAN_POINT('Ctrl Pts',(-45.9530149611248,49.5708953920363,-1.42664776486198));
#41383=CARTESIAN_POINT('Ctrl Pts',(-44.7187725399161,49.3334657337725,-1.49193528413041));
#41384=CARTESIAN_POINT('Ctrl Pts',(-43.8591065407153,48.6350014631945,-1.55722280339884));
#41385=CARTESIAN_POINT('Ctrl Pts',(-42.9994405415145,47.9365371926165,-1.62251032266727));
#41386=CARTESIAN_POINT('Ctrl Pts',(-42.5143509643218,46.7770383097244,-1.6877978419357));
#41387=CARTESIAN_POINT('Ctrl Pts',(-42.6205465557995,45.6744932226547,-1.75308536120414));
#41388=CARTESIAN_POINT('Ctrl Pts',(-42.7267421472772,44.571948135585,-1.81837288047257));
#41389=CARTESIAN_POINT('Ctrl Pts',(-43.4242229074254,43.5263568443378,-1.883660399741));
#41390=CARTESIAN_POINT('Ctrl Pts',(-44.4014005937706,43.0048149783333,-1.94894791900943));
#41391=CARTESIAN_POINT('Ctrl Pts',(-45.3785782801157,42.4832731123289,-2.01423543827786));
#41392=CARTESIAN_POINT('Ctrl Pts',(-46.6354528926579,42.4857806715673,-2.07952295754629));
#41393=CARTESIAN_POINT('Ctrl Pts',(-47.610540841459,43.0112185362442,-2.14481047681472));
#41394=CARTESIAN_POINT('Ctrl Pts',(-48.58562879026,43.5366564009211,-2.21009799608315));
#41395=CARTESIAN_POINT('Ctrl Pts',(-49.2789300753199,44.5850245710367,-2.27538551535158));
#41396=CARTESIAN_POINT('Ctrl Pts',(-49.3807251494168,45.6879841530277,-2.34067303462002));
#41397=CARTESIAN_POINT('Ctrl Pts',(-49.3902409166803,45.7910884218386,-2.34677608866349));
#41398=CARTESIAN_POINT('Ctrl Pts',(-49.394587840163,45.8946697346342,-2.35287914270696));
#41399=CARTESIAN_POINT('Ctrl Pts',(-49.3939446252011,45.9983056787136,-2.35898219675043));
#41400=CARTESIAN_POINT('Ctrl Pts',(-47.0579044229729,42.0543614925016,5.55111512312578E-16));
#41401=CARTESIAN_POINT('Ctrl Pts',(-47.1733692374414,42.0960014311082,5.66013339959512E-16));
#41402=CARTESIAN_POINT('Ctrl Pts',(-47.2864784544055,42.1431495258543,1.12270800514822E-15));
#41403=CARTESIAN_POINT('Ctrl Pts',(-47.3970074324165,42.1954516216316,9.71445146547012E-16));
#41404=CARTESIAN_POINT('Ctrl Pts',(-47.5098931343429,42.2488689145469,8.16957026998136E-16));
#41405=CARTESIAN_POINT('Ctrl Pts',(-47.620088014245,42.3076628912825,-2.48568638880629E-16));
#41406=CARTESIAN_POINT('Ctrl Pts',(-47.7273254658327,42.3715030108371,-1.94289029309402E-16));
#41407=CARTESIAN_POINT('Ctrl Pts',(-47.8392938527237,42.4381595296151,-1.37614796242688E-16));
#41408=CARTESIAN_POINT('Ctrl Pts',(-47.9480390302718,42.5103177737784,2.81552683011295E-16));
#41409=CARTESIAN_POINT('Ctrl Pts',(-48.0532159541544,42.5876437997826,2.08166817117217E-16));
#41410=CARTESIAN_POINT('Ctrl Pts',(-48.1452457625517,42.6553040725363,1.43954184459898E-16));
#41411=CARTESIAN_POINT('Ctrl Pts',(-48.234543268668,42.7269219306243,3.57553482541936E-16));
#41412=CARTESIAN_POINT('Ctrl Pts',(-48.3208447022047,42.8022930418766,2.91433543964104E-16));
#41413=CARTESIAN_POINT('Ctrl Pts',(-48.3378037817389,42.8171042057001,2.78440326456705E-16));
#41414=CARTESIAN_POINT('Ctrl Pts',(-48.3546470605663,42.8320603488493,-9.65298675504177E-17));
#41415=CARTESIAN_POINT('Ctrl Pts',(-48.3713723802753,42.8471599789909,-1.11022302462516E-16));
#41416=CARTESIAN_POINT('Ctrl Pts',(-48.3839949979561,42.8585556869185,-1.21959759464334E-16));
#41417=CARTESIAN_POINT('Ctrl Pts',(-48.3965503865158,42.8700331641752,6.34306447284316E-16));
#41418=CARTESIAN_POINT('Ctrl Pts',(-48.4090271849394,42.8815818936618,6.24500451351651E-16));
#41419=CARTESIAN_POINT('Ctrl Pts',(-48.4995023665661,42.9653272073537,5.53392525029661E-16));
#41420=CARTESIAN_POINT('Ctrl Pts',(-48.5859893911482,43.0529427915412,6.24851978512991E-16));
#41421=CARTESIAN_POINT('Ctrl Pts',(-48.6682306336821,43.1441142001542,5.55111512312578E-16));
#41422=CARTESIAN_POINT('Ctrl Pts',(-48.7501460833931,43.2349244397276,4.85647318000291E-16));
#41423=CARTESIAN_POINT('Ctrl Pts',(-48.8278497989444,43.3292631204114,2.29444790427909E-16));
#41424=CARTESIAN_POINT('Ctrl Pts',(-48.9010447261095,43.4268484092624,1.80411241501588E-16));
#41425=CARTESIAN_POINT('Ctrl Pts',(-48.9731604547005,43.5229948838586,1.32100651640001E-16));
#41426=CARTESIAN_POINT('Ctrl Pts',(-49.0408997240368,43.6222936314722,4.78619745031733E-16));
#41427=CARTESIAN_POINT('Ctrl Pts',(-49.1039311102743,43.7244925695876,5.55111512312578E-16));
#41428=CARTESIAN_POINT('Ctrl Pts',(-49.155490252746,43.8080904392409,6.17681132982036E-16));
#41429=CARTESIAN_POINT('Ctrl Pts',(-49.2038985462528,43.8936293247998,4.03026082704482E-17));
#41430=CARTESIAN_POINT('Ctrl Pts',(-49.2489479688624,43.9809753984075,-2.77555756156289E-17));
#41431=CARTESIAN_POINT('Ctrl Pts',(-49.2595819350771,44.0015935360423,-4.38207854709016E-17));
#41432=CARTESIAN_POINT('Ctrl Pts',(-49.270028632464,44.0223123771606,-2.25961482045739E-16));
#41433=CARTESIAN_POINT('Ctrl Pts',(-49.2802851129785,44.0431301684709,-2.4980018054066E-16));
#41434=CARTESIAN_POINT('Ctrl Pts',(-49.2875269453717,44.0578290659389,-2.66632061489241E-16));
#41435=CARTESIAN_POINT('Ctrl Pts',(-49.2946732228582,44.0725759485657,7.95634595235508E-16));
#41436=CARTESIAN_POINT('Ctrl Pts',(-49.301717831292,44.0873590873138,7.7715611723761E-16));
#41437=CARTESIAN_POINT('Ctrl Pts',(-49.3523570973335,44.1936257880164,6.44325943328169E-16));
#41438=CARTESIAN_POINT('Ctrl Pts',(-49.397823772424,44.3019195500152,4.63255393197704E-18));
#41439=CARTESIAN_POINT('Ctrl Pts',(-49.4378467145292,44.4119843341003,1.38777878078145E-16));
#41440=CARTESIAN_POINT('Ctrl Pts',(-49.4770635111394,44.5198321839678,2.70221235726126E-16));
#41441=CARTESIAN_POINT('Ctrl Pts',(-49.5110538889566,44.6293810645388,7.52076617720226E-16));
#41442=CARTESIAN_POINT('Ctrl Pts',(-49.5395138665875,44.7404008831522,8.04911692853238E-16));
#41443=CARTESIAN_POINT('Ctrl Pts',(-49.5449744944973,44.7617023025674,8.15049180999944E-16));
#41444=CARTESIAN_POINT('Ctrl Pts',(-49.5502313718793,44.7830578900246,-4.5156980917228E-16));
#41445=CARTESIAN_POINT('Ctrl Pts',(-49.5552821294542,44.804466037532,-4.71844785465692E-16));
#41446=CARTESIAN_POINT('Ctrl Pts',(-49.5824900757527,44.9197896734607,-6.10151655747883E-16));
#41447=CARTESIAN_POINT('Ctrl Pts',(-49.6037208233721,45.0366392601437,7.24995094299097E-16));
#41448=CARTESIAN_POINT('Ctrl Pts',(-49.6190589580299,45.1545782432542,8.04911692853238E-16));
#41449=CARTESIAN_POINT('Ctrl Pts',(-49.6275693456393,45.2200168694572,8.4925354049578E-16));
#41450=CARTESIAN_POINT('Ctrl Pts',(-49.6342647061823,45.285790742732,9.91139680797571E-17));
#41451=CARTESIAN_POINT('Ctrl Pts',(-49.6391528952321,45.3518232724505,5.55111512312578E-17));
#41452=CARTESIAN_POINT('Ctrl Pts',(-49.6410791584549,45.3778443678321,3.83288160858751E-17));
#41453=CARTESIAN_POINT('Ctrl Pts',(-49.6427247418287,45.4039056075073,7.48033515296283E-16));
#41454=CARTESIAN_POINT('Ctrl Pts',(-49.6440899361851,45.4300022098967,7.7715611723761E-16));
#41455=CARTESIAN_POINT('Ctrl Pts',(-49.6449643353021,45.4467169333192,7.95808975932785E-16));
#41456=CARTESIAN_POINT('Ctrl Pts',(-49.6457236611113,45.4634466313103,-2.3566119177251E-16));
#41457=CARTESIAN_POINT('Ctrl Pts',(-49.6463675672004,45.4801746114213,-2.22044604925031E-16));
#41458=CARTESIAN_POINT('Ctrl Pts',(-49.650944859773,45.5990876958098,-1.25249275773564E-16));
#41459=CARTESIAN_POINT('Ctrl Pts',(-49.6497054380441,45.7181030341178,-2.85690848750654E-16));
#41460=CARTESIAN_POINT('Ctrl Pts',(-49.642802430889,45.8367853608077,-2.22044604925031E-16));
#41461=CARTESIAN_POINT('Ctrl Pts',(-49.6360413171965,45.9530281353007,-1.59706629468275E-16));
#41462=CARTESIAN_POINT('Ctrl Pts',(-49.6238465215681,46.0689523583233,3.31802632205194E-16));
#41463=CARTESIAN_POINT('Ctrl Pts',(-49.6063095800648,46.1841392093055,1.11022302462516E-16));
#41464=CARTESIAN_POINT('Ctrl Pts',(-49.5889758936611,46.297991031893,-1.07199158740278E-16));
#41465=CARTESIAN_POINT('Ctrl Pts',(-49.5664227750947,46.4111232891586,5.10322680618708E-17));
#41466=CARTESIAN_POINT('Ctrl Pts',(-49.5386937107918,46.5231091504923,-5.55111512312578E-17));
#41467=CARTESIAN_POINT('Ctrl Pts',(-49.5206040122694,46.5961657256503,-1.25017223037783E-16));
#41468=CARTESIAN_POINT('Ctrl Pts',(-49.5003105810002,46.6687339212223,-6.47114358888512E-16));
#41469=CARTESIAN_POINT('Ctrl Pts',(-49.477816188174,46.7406875318196,-7.21644966006352E-16));
#41470=CARTESIAN_POINT('Ctrl Pts',(-49.4685898886408,46.7702000227321,-7.52214437739744E-16));
#41471=CARTESIAN_POINT('Ctrl Pts',(-49.458993237021,46.799609039298,3.77824931536309E-18));
#41472=CARTESIAN_POINT('Ctrl Pts',(-49.4490260923412,46.8289055070053,0.));
#41473=CARTESIAN_POINT('Ctrl Pts',(-49.4429393126163,46.8467964026811,-2.30731789967445E-18));
#41474=CARTESIAN_POINT('Ctrl Pts',(-49.4367170562216,46.8646373229998,2.9761811420164E-16));
#41475=CARTESIAN_POINT('Ctrl Pts',(-49.4303611602144,46.8824221857011,3.33066907387547E-16));
#41476=CARTESIAN_POINT('Ctrl Pts',(-49.392180766493,46.9892573289204,5.46010743984259E-16));
#41477=CARTESIAN_POINT('Ctrl Pts',(-49.3491646814368,47.0941213407157,-6.96374359617231E-16));
#41478=CARTESIAN_POINT('Ctrl Pts',(-49.3013722120853,47.1966033447963,-6.66133814775094E-16));
#41479=CARTESIAN_POINT('Ctrl Pts',(-49.2629805514864,47.278927074278,-6.41841604105534E-16));
#41480=CARTESIAN_POINT('Ctrl Pts',(-49.2215058246924,47.3597134134632,1.18644211359586E-16));
#41481=CARTESIAN_POINT('Ctrl Pts',(-49.1769600904346,47.4387325885125,2.77555756156289E-16));
#41482=CARTESIAN_POINT('Ctrl Pts',(-49.1548835763497,47.4778938675894,3.56311062706237E-16));
#41483=CARTESIAN_POINT('Ctrl Pts',(-49.1320525422512,47.5166208499627,-1.58005809035499E-16));
#41484=CARTESIAN_POINT('Ctrl Pts',(-49.1084670740132,47.5548838684341,-1.66533453693773E-16));
#41485=CARTESIAN_POINT('Ctrl Pts',(-49.0950717251622,47.5766153208413,-1.71376723029023E-16));
#41486=CARTESIAN_POINT('Ctrl Pts',(-49.0814312209137,47.5981996315565,7.12245490477885E-18));
#41487=CARTESIAN_POINT('Ctrl Pts',(-49.0675592202023,47.6196105788371,0.));
#41488=CARTESIAN_POINT('Ctrl Pts',(-49.0090089012406,47.709980945637,-3.0062138485895E-17));
#41489=CARTESIAN_POINT('Ctrl Pts',(-48.9462915591126,47.7973423071076,5.3888875104828E-16));
#41490=CARTESIAN_POINT('Ctrl Pts',(-48.8794391108352,47.8813135513516,3.88578058618805E-16));
#41491=CARTESIAN_POINT('Ctrl Pts',(-48.8212022036609,47.954463087118,2.57638503406439E-16));
#41492=CARTESIAN_POINT('Ctrl Pts',(-48.7598266730131,48.0250397676994,8.03315147564942E-16));
#41493=CARTESIAN_POINT('Ctrl Pts',(-48.6953141039964,48.0927658834935,9.99200722162641E-16));
#41494=CARTESIAN_POINT('Ctrl Pts',(-48.6572947310406,48.1326791049708,1.06036603675156E-15));
#41495=CARTESIAN_POINT('Ctrl Pts',(-48.6181854212265,48.1716017502292,2.12735497367301E-16));
#41496=CARTESIAN_POINT('Ctrl Pts',(-48.5780352480409,48.2095125055216,2.77555756156289E-16));
#41497=CARTESIAN_POINT('Origin',(-46.,46.,-5.));
#41498=CARTESIAN_POINT('Origin',(46.,-46.,-9.));
#41499=CARTESIAN_POINT('Ctrl Pts',(47.3033820408749,-42.8708467090881,-9.));
#41500=CARTESIAN_POINT('Ctrl Pts',(47.2095002176375,-42.8200478993858,-9.));
#41501=CARTESIAN_POINT('Ctrl Pts',(47.1132610952936,-42.7741603120111,-9.));
#41502=CARTESIAN_POINT('Ctrl Pts',(47.0150558684064,-42.7330710668746,-9.));
#41503=CARTESIAN_POINT('Ctrl Pts',(46.9145913812888,-42.6910365431579,-9.));
#41504=CARTESIAN_POINT('Ctrl Pts',(46.8120687118127,-42.6540234152959,-9.));
#41505=CARTESIAN_POINT('Ctrl Pts',(46.7078720919618,-42.6219531198193,-9.));
#41506=CARTESIAN_POINT('Ctrl Pts',(46.6771618756247,-42.6125009349644,-9.));
#41507=CARTESIAN_POINT('Ctrl Pts',(46.6463060552087,-42.6034784112983,-9.));
#41508=CARTESIAN_POINT('Ctrl Pts',(46.6153140309619,-42.594884267454,-9.));
#41509=CARTESIAN_POINT('Ctrl Pts',(46.5945562374165,-42.5891280941173,-9.));
#41510=CARTESIAN_POINT('Ctrl Pts',(46.5737373386698,-42.5835641003044,-9.));
#41511=CARTESIAN_POINT('Ctrl Pts',(46.5528601193257,-42.5781919859202,-9.));
#41512=CARTESIAN_POINT('Ctrl Pts',(46.5322674936134,-42.5728931030098,-9.));
#41513=CARTESIAN_POINT('Ctrl Pts',(46.511625647447,-42.5677828752221,-9.));
#41514=CARTESIAN_POINT('Ctrl Pts',(46.4909429939031,-42.562861907011,-9.));
#41515=CARTESIAN_POINT('Ctrl Pts',(46.3816028037924,-42.5368468892283,-9.));
#41516=CARTESIAN_POINT('Ctrl Pts',(46.2710760141354,-42.5161050297694,-9.));
#41517=CARTESIAN_POINT('Ctrl Pts',(46.1597772205501,-42.5005437397571,-9.));
#41518=CARTESIAN_POINT('Ctrl Pts',(46.064224827999,-42.4871840397643,-9.));
#41519=CARTESIAN_POINT('Ctrl Pts',(45.9681025618294,-42.477643419586,-9.));
#41520=CARTESIAN_POINT('Ctrl Pts',(45.871658973384,-42.471890733761,-9.));
#41521=CARTESIAN_POINT('Ctrl Pts',(45.8389980828378,-42.469942570642,-9.));
#41522=CARTESIAN_POINT('Ctrl Pts',(45.8063002614413,-42.4684290474514,-9.));
#41523=CARTESIAN_POINT('Ctrl Pts',(45.7735749583434,-42.4673496294112,-9.));
#41524=CARTESIAN_POINT('Ctrl Pts',(45.7546017607775,-42.4667238136114,-9.));
#41525=CARTESIAN_POINT('Ctrl Pts',(45.7356172459526,-42.4662438876058,-9.));
#41526=CARTESIAN_POINT('Ctrl Pts',(45.7166298744102,-42.46590991102,-9.));
#41527=CARTESIAN_POINT('Ctrl Pts',(45.6016682057186,-42.4638878035618,-9.));
#41528=CARTESIAN_POINT('Ctrl Pts',(45.4868633730437,-42.4672155558052,-9.));
#41529=CARTESIAN_POINT('Ctrl Pts',(45.3726343407908,-42.4757909550345,-9.));
#41530=CARTESIAN_POINT('Ctrl Pts',(45.2568060982418,-42.4844864101417,-9.));
#41531=CARTESIAN_POINT('Ctrl Pts',(45.1415690483829,-42.4985772818533,-9.));
#41532=CARTESIAN_POINT('Ctrl Pts',(45.027340505856,-42.5180066648298,-9.));
#41533=CARTESIAN_POINT('Ctrl Pts',(44.9134537535134,-42.5373779119652,-9.));
#41534=CARTESIAN_POINT('Ctrl Pts',(44.8005685677885,-42.5620557089792,-9.));
#41535=CARTESIAN_POINT('Ctrl Pts',(44.6890925895062,-42.59203438769,-9.));
#41536=CARTESIAN_POINT('Ctrl Pts',(44.6225628516896,-42.609925898179,-9.));
#41537=CARTESIAN_POINT('Ctrl Pts',(44.5565349943705,-42.6297064480852,-9.));
#41538=CARTESIAN_POINT('Ctrl Pts',(44.4910967187206,-42.6513836327597,-9.));
#41539=CARTESIAN_POINT('Ctrl Pts',(44.4459984914548,-42.6663229414629,-9.));
#41540=CARTESIAN_POINT('Ctrl Pts',(44.4011803109893,-42.6821632091557,-9.));
#41541=CARTESIAN_POINT('Ctrl Pts',(44.3566714285601,-42.6989087753146,-9.));
#41542=CARTESIAN_POINT('Ctrl Pts',(44.3429060791653,-42.7040877094151,-9.));
#41543=CARTESIAN_POINT('Ctrl Pts',(44.3291728649523,-42.7093523251889,-9.));
#41544=CARTESIAN_POINT('Ctrl Pts',(44.3154805206596,-42.7146994889312,-9.));
#41545=CARTESIAN_POINT('Ctrl Pts',(44.2045216811668,-42.7580313735766,-9.));
#41546=CARTESIAN_POINT('Ctrl Pts',(44.0960958559045,-42.8068365700647,-9.));
#41547=CARTESIAN_POINT('Ctrl Pts',(43.9906304039359,-42.8610553783041,-9.));
#41548=CARTESIAN_POINT('Ctrl Pts',(43.9680107837524,-42.8726839147232,-9.));
#41549=CARTESIAN_POINT('Ctrl Pts',(43.9455273277897,-42.884561663214,-9.));
#41550=CARTESIAN_POINT('Ctrl Pts',(43.9231842511489,-42.8966883475411,-9.));
#41551=CARTESIAN_POINT('Ctrl Pts',(43.8230347394897,-42.9510444030179,-9.));
#41552=CARTESIAN_POINT('Ctrl Pts',(43.7257044811106,-43.0103978109749,-9.));
#41553=CARTESIAN_POINT('Ctrl Pts',(43.6313338306458,-43.0743591133346,-9.));
#41554=CARTESIAN_POINT('Ctrl Pts',(43.5349268596731,-43.1397005663137,-9.));
#41555=CARTESIAN_POINT('Ctrl Pts',(43.4416080440628,-43.2098513003804,-9.));
#41556=CARTESIAN_POINT('Ctrl Pts',(43.3515468190621,-43.2844468665137,-9.));
#41557=CARTESIAN_POINT('Ctrl Pts',(43.3010492668727,-43.3262727854248,-9.));
#41558=CARTESIAN_POINT('Ctrl Pts',(43.2515762599215,-43.3694969769026,-9.));
#41559=CARTESIAN_POINT('Ctrl Pts',(43.2031613209412,-43.4140612153216,-9.));
#41560=CARTESIAN_POINT('Ctrl Pts',(43.1829736128673,-43.432643286366,-9.));
#41561=CARTESIAN_POINT('Ctrl Pts',(43.1629699022135,-43.451458393887,-9.));
#41562=CARTESIAN_POINT('Ctrl Pts',(43.1431527778045,-43.4705025119526,-9.));
#41563=CARTESIAN_POINT('Ctrl Pts',(43.132421404081,-43.480815287105,-9.));
#41564=CARTESIAN_POINT('Ctrl Pts',(43.121746294682,-43.4911937816965,-9.));
#41565=CARTESIAN_POINT('Ctrl Pts',(43.1111342308463,-43.5016308664422,-9.));
#41566=CARTESIAN_POINT('Ctrl Pts',(43.0256549583025,-43.5857006972837,-9.));
#41567=CARTESIAN_POINT('Ctrl Pts',(42.9441443682772,-43.673682830914,-9.));
#41568=CARTESIAN_POINT('Ctrl Pts',(42.866748874609,-43.7651447138442,-9.));
#41569=CARTESIAN_POINT('Ctrl Pts',(42.7879338689578,-43.858284100627,-9.));
#41570=CARTESIAN_POINT('Ctrl Pts',(42.7133857019319,-43.9550325573196,-9.));
#41571=CARTESIAN_POINT('Ctrl Pts',(42.6432828812115,-44.0549833302515,-9.));
#41572=CARTESIAN_POINT('Ctrl Pts',(42.5726118605758,-44.1557442277995,-9.));
#41573=CARTESIAN_POINT('Ctrl Pts',(42.5064579319861,-44.2597602054382,-9.));
#41574=CARTESIAN_POINT('Ctrl Pts',(42.4450370917787,-44.3666560823119,-9.));
#41575=CARTESIAN_POINT('Ctrl Pts',(42.4087736821331,-44.4297683575496,-9.));
#41576=CARTESIAN_POINT('Ctrl Pts',(42.3741608145198,-44.4938852541093,-9.));
#41577=CARTESIAN_POINT('Ctrl Pts',(42.3412496253407,-44.558934856722,-9.));
#41578=CARTESIAN_POINT('Ctrl Pts',(42.3239094669499,-44.5932080155078,-9.));
#41579=CARTESIAN_POINT('Ctrl Pts',(42.3070417829367,-44.6277401515673,-9.));
#41580=CARTESIAN_POINT('Ctrl Pts',(42.2906546830202,-44.6625210933121,-9.));
#41581=CARTESIAN_POINT('Ctrl Pts',(42.2831062240436,-44.6785423852592,-9.));
#41582=CARTESIAN_POINT('Ctrl Pts',(42.2756589959128,-44.6946181175088,-9.));
#41583=CARTESIAN_POINT('Ctrl Pts',(42.2683161828643,-44.7107421228823,-9.));
#41584=CARTESIAN_POINT('Ctrl Pts',(42.2159001543897,-44.8258419244431,-9.));
#41585=CARTESIAN_POINT('Ctrl Pts',(42.168966222388,-44.943034798637,-9.));
#41586=CARTESIAN_POINT('Ctrl Pts',(42.1276953421017,-45.0618930156386,-9.));
#41587=CARTESIAN_POINT('Ctrl Pts',(42.0863446247567,-45.1809811596584,-9.));
#41588=CARTESIAN_POINT('Ctrl Pts',(42.0506783113667,-45.3017418378647,-9.));
#41589=CARTESIAN_POINT('Ctrl Pts',(42.0209163435797,-45.4237808328287,-9.));
#41590=CARTESIAN_POINT('Ctrl Pts',(41.9916671564445,-45.5437171699371,-9.));
#41591=CARTESIAN_POINT('Ctrl Pts',(41.9681201892527,-45.664888939155,-9.));
#41592=CARTESIAN_POINT('Ctrl Pts',(41.9505280204683,-45.7869452163697,-9.));
#41593=CARTESIAN_POINT('Ctrl Pts',(41.9396360398584,-45.8625148985972,-9.));
#41594=CARTESIAN_POINT('Ctrl Pts',(41.9310276093539,-45.9384240544824,-9.));
#41595=CARTESIAN_POINT('Ctrl Pts',(41.9247724176044,-46.0145920214405,-9.));
#41596=CARTESIAN_POINT('Ctrl Pts',(41.919370954043,-46.0803643453827,-9.));
#41597=CARTESIAN_POINT('Ctrl Pts',(41.9157243497761,-46.1463297083195,-9.));
#41598=CARTESIAN_POINT('Ctrl Pts',(41.9138040800513,-46.2124372338607,-9.));
#41599=CARTESIAN_POINT('Ctrl Pts',(42.5743852316216,-48.2253962475631,-9.));
#41600=CARTESIAN_POINT('Ctrl Pts',(42.6510842550578,-48.3241664787627,-9.));
#41601=CARTESIAN_POINT('Ctrl Pts',(42.7325420415582,-48.4189430401456,-9.00000000000001));
#41602=CARTESIAN_POINT('Ctrl Pts',(42.8183507401128,-48.5095866491488,-9.));
#41603=CARTESIAN_POINT('Ctrl Pts',(42.9053643616367,-48.6015030727773,-9.));
#41604=CARTESIAN_POINT('Ctrl Pts',(42.9968527373842,-48.689170063398,-9.));
#41605=CARTESIAN_POINT('Ctrl Pts',(43.0924206860801,-48.7723984663639,-9.));
#41606=CARTESIAN_POINT('Ctrl Pts',(43.13283898909,-48.8075980375173,-9.));
#41607=CARTESIAN_POINT('Ctrl Pts',(43.173987290164,-48.8420031211714,-9.));
#41608=CARTESIAN_POINT('Ctrl Pts',(43.2158367460076,-48.8755968220645,-9.));
#41609=CARTESIAN_POINT('Ctrl Pts',(43.2398457476193,-48.8948695032171,-9.));
#41610=CARTESIAN_POINT('Ctrl Pts',(43.2640899473829,-48.9138783400765,-9.));
#41611=CARTESIAN_POINT('Ctrl Pts',(43.2885385460266,-48.9326008816648,-9.));
#41612=CARTESIAN_POINT('Ctrl Pts',(43.3879651732933,-49.0087409987781,-9.));
#41613=CARTESIAN_POINT('Ctrl Pts',(43.4908354399055,-49.0802047565596,-9.));
#41614=CARTESIAN_POINT('Ctrl Pts',(43.5967559275673,-49.1468201834493,-9.));
#41615=CARTESIAN_POINT('Ctrl Pts',(43.6847795863373,-49.202179951279,-9.));
#41616=CARTESIAN_POINT('Ctrl Pts',(43.7749105352022,-49.2541906389536,-9.00000000000001));
#41617=CARTESIAN_POINT('Ctrl Pts',(43.8669315767247,-49.3027275435314,-9.00000000000001));
#41618=CARTESIAN_POINT('Ctrl Pts',(43.9071907823908,-49.3239624392841,-9.00000000000001));
#41619=CARTESIAN_POINT('Ctrl Pts',(43.9478118296589,-49.3445321151676,-9.));
#41620=CARTESIAN_POINT('Ctrl Pts',(43.9887767271923,-49.3644246152224,-9.));
#41621=CARTESIAN_POINT('Ctrl Pts',(44.011146208365,-49.37528720569,-9.));
#41622=CARTESIAN_POINT('Ctrl Pts',(44.0336182221398,-49.3859478550071,-9.));
#41623=CARTESIAN_POINT('Ctrl Pts',(44.0561898414164,-49.396404496071,-9.));
#41624=CARTESIAN_POINT('Ctrl Pts',(44.0723897277928,-49.4039093363325,-9.));
#41625=CARTESIAN_POINT('Ctrl Pts',(44.0886323780177,-49.411305127036,-9.00000000000001));
#41626=CARTESIAN_POINT('Ctrl Pts',(44.1049159223051,-49.4185911402604,-9.00000000000001));
#41627=CARTESIAN_POINT('Ctrl Pts',(44.2166372855396,-49.468580461725,-9.00000000000001));
#41628=CARTESIAN_POINT('Ctrl Pts',(44.3302932415966,-49.5134112908577,-9.));
#41629=CARTESIAN_POINT('Ctrl Pts',(44.4455169815829,-49.5529254759394,-9.));
#41630=CARTESIAN_POINT('Ctrl Pts',(44.5598774224311,-49.5921436060422,-9.));
#41631=CARTESIAN_POINT('Ctrl Pts',(44.67578306281,-49.6261246444362,-9.));
#41632=CARTESIAN_POINT('Ctrl Pts',(44.7928842528278,-49.6546636633717,-9.));
#41633=CARTESIAN_POINT('Ctrl Pts',(44.9068413606339,-49.682436430301,-9.));
#41634=CARTESIAN_POINT('Ctrl Pts',(45.0219313774996,-49.7050554811712,-9.));
#41635=CARTESIAN_POINT('Ctrl Pts',(45.1378294998974,-49.7222830855843,-9.));
#41636=CARTESIAN_POINT('Ctrl Pts',(45.2059630414309,-49.732410753544,-9.));
#41637=CARTESIAN_POINT('Ctrl Pts',(45.2743757607225,-49.7406742325277,-9.));
#41638=CARTESIAN_POINT('Ctrl Pts',(45.3429998134215,-49.7470169883357,-9.));
#41639=CARTESIAN_POINT('Ctrl Pts',(45.3908534678175,-49.7514399862849,-9.));
#41640=CARTESIAN_POINT('Ctrl Pts',(45.4388098562325,-49.7549288664261,-9.));
#41641=CARTESIAN_POINT('Ctrl Pts',(45.4868453505332,-49.7574626301393,-9.));
#41642=CARTESIAN_POINT('Ctrl Pts',(45.5023235914912,-49.7582790723526,-9.));
#41643=CARTESIAN_POINT('Ctrl Pts',(45.5178066093579,-49.7589961163705,-9.00000000000001));
#41644=CARTESIAN_POINT('Ctrl Pts',(45.5332851460771,-49.7596129312151,-9.00000000000001));
#41645=CARTESIAN_POINT('Ctrl Pts',(45.6490326352122,-49.764225432436,-9.00000000000001));
#41646=CARTESIAN_POINT('Ctrl Pts',(45.764670435547,-49.7632450163518,-9.));
#41647=CARTESIAN_POINT('Ctrl Pts',(45.8798848286888,-49.7564882368775,-9.));
#41648=CARTESIAN_POINT('Ctrl Pts',(45.9071546175464,-49.7548889926807,-9.));
#41649=CARTESIAN_POINT('Ctrl Pts',(45.9344006665752,-49.752965923366,-9.00000000000001));
#41650=CARTESIAN_POINT('Ctrl Pts',(45.9616187611747,-49.7507161676903,-9.00000000000001));
#41651=CARTESIAN_POINT('Ctrl Pts',(46.0782931677331,-49.7410722557185,-9.00000000000001));
#41652=CARTESIAN_POINT('Ctrl Pts',(46.1944552709857,-49.725429296288,-9.));
#41653=CARTESIAN_POINT('Ctrl Pts',(46.3097422789741,-49.7040305580922,-9.));
#41654=CARTESIAN_POINT('Ctrl Pts',(46.4259795694295,-49.6824554353576,-9.));
#41655=CARTESIAN_POINT('Ctrl Pts',(46.5413280980213,-49.6550287317031,-9.));
#41656=CARTESIAN_POINT('Ctrl Pts',(46.6553913624472,-49.6219534192776,-9.));
#41657=CARTESIAN_POINT('Ctrl Pts',(46.7119959587765,-49.6055395921112,-9.));
#41658=CARTESIAN_POINT('Ctrl Pts',(46.7682835756122,-49.5877340165484,-9.));
#41659=CARTESIAN_POINT('Ctrl Pts',(46.8242025716789,-49.5685579250005,-9.));
#41660=CARTESIAN_POINT('Ctrl Pts',(46.8468231694633,-49.5608007282607,-9.));
#41661=CARTESIAN_POINT('Ctrl Pts',(46.8693834188428,-49.5528192356515,-9.));
#41662=CARTESIAN_POINT('Ctrl Pts',(46.8918797845697,-49.5446147561897,-9.));
#41663=CARTESIAN_POINT('Ctrl Pts',(46.907099956639,-49.5390639223056,-9.));
#41664=CARTESIAN_POINT('Ctrl Pts',(46.9222905170742,-49.5334110892113,-9.));
#41665=CARTESIAN_POINT('Ctrl Pts',(46.9374375956582,-49.5276616978241,-9.));
#41666=CARTESIAN_POINT('Ctrl Pts',(47.0458981301604,-49.4864932269893,-9.));
#41667=CARTESIAN_POINT('Ctrl Pts',(47.1523014498086,-49.4403165384569,-9.));
#41668=CARTESIAN_POINT('Ctrl Pts',(47.2563056915469,-49.3893803260793,-9.));
#41669=CARTESIAN_POINT('Ctrl Pts',(47.3602083916416,-49.3384938438533,-9.));
#41670=CARTESIAN_POINT('Ctrl Pts',(47.4617174352489,-49.2828565194432,-9.));
#41671=CARTESIAN_POINT('Ctrl Pts',(47.5604628206564,-49.222673454704,-9.));
#41672=CARTESIAN_POINT('Ctrl Pts',(47.6578162292091,-49.1633387681732,-9.));
#41673=CARTESIAN_POINT('Ctrl Pts',(47.7524839476778,-49.0995849704782,-9.));
#41674=CARTESIAN_POINT('Ctrl Pts',(47.8440732492731,-49.0315762020744,-9.));
#41675=CARTESIAN_POINT('Ctrl Pts',(47.8943353485933,-48.9942545562859,-9.));
#41676=CARTESIAN_POINT('Ctrl Pts',(47.9436696390876,-48.9556509834542,-9.));
#41677=CARTESIAN_POINT('Ctrl Pts',(47.9920052439302,-48.9157893805739,-9.));
#41678=CARTESIAN_POINT('Ctrl Pts',(48.0190282317517,-48.8935039532438,-9.));
#41679=CARTESIAN_POINT('Ctrl Pts',(48.0457389902699,-48.8708252799141,-9.));
#41680=CARTESIAN_POINT('Ctrl Pts',(48.072124481961,-48.8477572841386,-9.));
#41681=CARTESIAN_POINT('Ctrl Pts',(48.0885412369069,-48.8334046376852,-9.));
#41682=CARTESIAN_POINT('Ctrl Pts',(48.1048355682913,-48.8188979730226,-9.));
#41683=CARTESIAN_POINT('Ctrl Pts',(48.1209823789593,-48.8042583984171,-9.));
#41684=CARTESIAN_POINT('Ctrl Pts',(48.2035982369658,-48.7293543791815,-9.));
#41685=CARTESIAN_POINT('Ctrl Pts',(48.2824582102327,-48.6508865866008,-9.));
#41686=CARTESIAN_POINT('Ctrl Pts',(48.3572280393153,-48.5690423763841,-9.));
#41687=CARTESIAN_POINT('Ctrl Pts',(48.4308862472868,-48.4884149638116,-9.));
#41688=CARTESIAN_POINT('Ctrl Pts',(48.5005755215514,-48.4045101950566,-9.));
#41689=CARTESIAN_POINT('Ctrl Pts',(48.565933985507,-48.3174806712345,-9.));
#41690=CARTESIAN_POINT('Ctrl Pts',(48.6294066043965,-48.23296228657,-9.));
#41691=CARTESIAN_POINT('Ctrl Pts',(48.6887950229853,-48.1454963378325,-9.));
#41692=CARTESIAN_POINT('Ctrl Pts',(48.7437220341769,-48.0552055938548,-9.));
#41693=CARTESIAN_POINT('Ctrl Pts',(48.771376110491,-48.0097469557412,-9.));
#41694=CARTESIAN_POINT('Ctrl Pts',(48.7978985435134,-47.9635720608222,-9.));
#41695=CARTESIAN_POINT('Ctrl Pts',(48.8232362548565,-47.9166954935817,-9.));
#41696=CARTESIAN_POINT('Ctrl Pts',(48.8494364512248,-47.8682232677308,-9.));
#41697=CARTESIAN_POINT('Ctrl Pts',(48.8743698413062,-47.8190007093841,-9.));
#41698=CARTESIAN_POINT('Ctrl Pts',(48.8980278172144,-47.7690799369094,-9.));
#41699=CARTESIAN_POINT('Origin',(46.,-46.,2.76038497140452));
#41700=CARTESIAN_POINT('Ctrl Pts',(41.9098425569998,-45.9981377324218,-0.364615028595479));
#41701=CARTESIAN_POINT('Ctrl Pts',(41.9091325173901,-45.879255340082,-0.370425837919348));
#41702=CARTESIAN_POINT('Ctrl Pts',(41.9672597965486,-44.4253404423929,-0.441524166511649));
#41703=CARTESIAN_POINT('Ctrl Pts',(43.700874641208,-41.7778217753375,-0.577910014372381));
#41704=CARTESIAN_POINT('Ctrl Pts',(48.2448534714975,-41.7491667594488,-0.773772572177674));
#41705=CARTESIAN_POINT('Ctrl Pts',(50.7830591782025,-45.5179447043461,-0.969635129982967));
#41706=CARTESIAN_POINT('Ctrl Pts',(49.0478255306161,-49.7176766340539,-1.16549768778826));
#41707=CARTESIAN_POINT('Ctrl Pts',(44.5894569428605,-50.5956818776348,-1.36136024559355));
#41708=CARTESIAN_POINT('Ctrl Pts',(42.1450235329037,-48.1283900611451,-1.51106602586263));
#41709=CARTESIAN_POINT('Ctrl Pts',(41.9140056632401,-46.3965852194679,-1.59548428686327));
#41710=CARTESIAN_POINT('Ctrl Pts',(41.9171327032046,-46.0033110738038,-1.61461502859548));
#41711=CARTESIAN_POINT('Ctrl Pts',(41.9194196464784,-46.0038358614086,-0.260384971404518));
#41712=CARTESIAN_POINT('Ctrl Pts',(41.9254629522515,-45.1031478464201,-0.304165019473208));
#41713=CARTESIAN_POINT('Ctrl Pts',(42.6573083539943,-42.8475830013967,-0.413232586810328));
#41714=CARTESIAN_POINT('Ctrl Pts',(46.3558078226787,-41.2067330502749,-0.58758767341588));
#41715=CARTESIAN_POINT('Ctrl Pts',(50.1895243958238,-43.6427681215851,-0.783450231221173));
#41716=CARTESIAN_POINT('Ctrl Pts',(50.2815817385072,-48.1865095580738,-0.979312789026466));
#41717=CARTESIAN_POINT('Ctrl Pts',(46.547466535547,-50.7759010051096,-1.17517534683176));
#41718=CARTESIAN_POINT('Ctrl Pts',(42.7307419251195,-49.2599206787868,-1.35219940762444));
#41719=CARTESIAN_POINT('Ctrl Pts',(41.9246674400896,-46.9514404731118,-1.4639359491487));
#41720=CARTESIAN_POINT('Ctrl Pts',(41.9169762239431,-45.9966653623493,-1.51038497140452));
#41721=CARTESIAN_POINT('Ctrl Pts',(48.5732344270147,-43.7934484719077,0.));
#41722=CARTESIAN_POINT('Ctrl Pts',(49.2973603516436,-44.6379090408209,-0.0652875192684312));
#41723=CARTESIAN_POINT('Ctrl Pts',(49.8377909604978,-47.0815093877498,-0.195862557805293));
#41724=CARTESIAN_POINT('Ctrl Pts',(47.2195289512052,-49.8003259140453,-0.391725115610587));
#41725=CARTESIAN_POINT('Ctrl Pts',(43.5104537866883,-49.1160268913033,-0.58758767341588));
#41726=CARTESIAN_POINT('Ctrl Pts',(42.0262712437735,-45.6513999754492,-0.783450231221174));
#41727=CARTESIAN_POINT('Ctrl Pts',(44.0921762093107,-42.4964189382987,-0.979312789026468));
#41728=CARTESIAN_POINT('Ctrl Pts',(47.8627887527562,-42.4726408868645,-1.17517534683176));
#41729=CARTESIAN_POINT('Ctrl Pts',(49.9690024110922,-45.5999885095611,-1.37103790463705));
#41730=CARTESIAN_POINT('Ctrl Pts',(48.5290983090345,-49.0849435422972,-1.56690046244235));
#41731=CARTESIAN_POINT('Ctrl Pts',(44.8295255011166,-49.8135159472981,-1.76276302024764));
#41732=CARTESIAN_POINT('Ctrl Pts',(42.1757347751709,-47.1349090709021,-1.95862557805294));
#41733=CARTESIAN_POINT('Ctrl Pts',(42.9387743307483,-43.4422796081895,-2.15448813585823));
#41734=CARTESIAN_POINT('Ctrl Pts',(46.436903464158,-42.034887332994,-2.35035069366352));
#41735=CARTESIAN_POINT('Ctrl Pts',(49.5446751782708,-44.1701650985836,-2.54621325146882));
#41736=CARTESIAN_POINT('Ctrl Pts',(49.485416115998,-47.9403330390778,-2.74207580927411));
#41737=CARTESIAN_POINT('Ctrl Pts',(46.3120712894746,-49.9768864478569,-2.9379383670794));
#41738=CARTESIAN_POINT('Ctrl Pts',(42.8599028524774,-48.4602451351121,-3.13380092488469));
#41739=CARTESIAN_POINT('Ctrl Pts',(42.2132906545528,-44.7454688702612,-3.32966348268999));
#41740=CARTESIAN_POINT('Ctrl Pts',(44.9499579596742,-42.1515681913754,-3.52552604049528));
#41741=CARTESIAN_POINT('Ctrl Pts',(48.6247975171733,-42.9960935595406,-3.72138859830058));
#41742=CARTESIAN_POINT('Ctrl Pts',(49.9544812319427,-46.524494090566,-3.91725115610587));
#41743=CARTESIAN_POINT('Ctrl Pts',(47.7509877249507,-49.5842792607275,-4.11311371391117));
#41744=CARTESIAN_POINT('Ctrl Pts',(43.983053885447,-49.4416484758484,-4.30897627171645));
#41745=CARTESIAN_POINT('Ctrl Pts',(42.017183993459,-46.2240368540166,-4.50483882952175));
#41746=CARTESIAN_POINT('Ctrl Pts',(43.6098073546396,-42.8062569035684,-4.70070138732704));
#41747=CARTESIAN_POINT('Ctrl Pts',(47.3379761142184,-42.241963841087,-4.89656394513234));
#41748=CARTESIAN_POINT('Ctrl Pts',(49.8707145657737,-45.0353318650296,-5.09242650293763));
#41749=CARTESIAN_POINT('Ctrl Pts',(48.9451180958786,-48.6905938439567,-5.28828906074293));
#41750=CARTESIAN_POINT('Ctrl Pts',(45.3881716416347,-49.9419134851903,-5.48415161854822));
#41751=CARTESIAN_POINT('Ctrl Pts',(42.3778703273949,-47.6712846986755,-5.68001417635351));
#41752=CARTESIAN_POINT('Ctrl Pts',(42.6038029048162,-43.9074271905735,-5.8758767341588));
#41753=CARTESIAN_POINT('Ctrl Pts',(45.864107175315,-42.0132031450575,-6.0717392919641));
#41754=CARTESIAN_POINT('Ctrl Pts',(49.2458266222607,-43.6810291595308,-6.26760184976939));
#41755=CARTESIAN_POINT('Ctrl Pts',(49.7275242358509,-47.4207664762398,-6.46346440757469));
#41756=CARTESIAN_POINT('Ctrl Pts',(46.878822635117,-49.8911037740211,-6.65932696537998));
#41757=CARTESIAN_POINT('Ctrl Pts',(43.244925432142,-48.8848885613543,-6.85518952318528));
#41758=CARTESIAN_POINT('Ctrl Pts',(42.0725842897717,-45.3011373968387,-7.05105208099057));
#41759=CARTESIAN_POINT('Ctrl Pts',(44.4092329111238,-42.3417905650828,-7.24691463879586));
#41760=CARTESIAN_POINT('Ctrl Pts',(48.1671820163374,-42.6509187502963,-7.44277719660115));
#41761=CARTESIAN_POINT('Ctrl Pts',(49.9888143927997,-45.9523117139429,-7.63863975440644));
#41762=CARTESIAN_POINT('Ctrl Pts',(48.2466407242209,-49.2963343841598,-7.83450231221174));
#41763=CARTESIAN_POINT('Ctrl Pts',(44.4970846743848,-49.6951637116331,-8.03036487001703));
#41764=CARTESIAN_POINT('Ctrl Pts',(42.0905201956602,-46.7925982020384,-8.22622742782233));
#41765=CARTESIAN_POINT('Ctrl Pts',(43.1765285368071,-43.1816883123461,-8.42208998562762));
#41766=CARTESIAN_POINT('Ctrl Pts',(46.7860124730819,-42.08921662613,-8.61795254343292));
#41767=CARTESIAN_POINT('Ctrl Pts',(49.6915640274424,-44.4900930602074,-8.81381510123821));
#41768=CARTESIAN_POINT('Ctrl Pts',(49.302253143976,-48.24161818535,-9.0096776590435));
#41769=CARTESIAN_POINT('Ctrl Pts',(45.9554882647734,-49.987019026503,-9.2055402168488));
#41770=CARTESIAN_POINT('Ctrl Pts',(43.7634250628647,-48.7794980878294,-9.33611525538566));
#41771=CARTESIAN_POINT('Ctrl Pts',(43.1574106092752,-47.8466430673628,-9.40140277465409));
#41772=CARTESIAN_POINT('Ctrl Pts',(48.7491609934165,-43.6425912356409,0.133800924884696));
#41773=CARTESIAN_POINT('Ctrl Pts',(49.5227938678302,-44.5447857781054,0.0685134056162645));
#41774=CARTESIAN_POINT('Ctrl Pts',(50.1001725683141,-47.1554498850168,-0.0620616329205977));
#41775=CARTESIAN_POINT('Ctrl Pts',(47.3029055525598,-50.0601461162962,-0.257924190725891));
#41776=CARTESIAN_POINT('Ctrl Pts',(43.3402488055142,-49.3290630243691,-0.453786748531185));
#41777=CARTESIAN_POINT('Ctrl Pts',(41.7545958579027,-45.627566932986,-0.649649306336477));
#41778=CARTESIAN_POINT('Ctrl Pts',(43.9617423532765,-42.256886550645,-0.845511864141773));
#41779=CARTESIAN_POINT('Ctrl Pts',(47.9901436590033,-42.2314828443926,-1.04137442194706));
#41780=CARTESIAN_POINT('Ctrl Pts',(50.2403546667957,-45.5726405744894,-1.23723697975236));
#41781=CARTESIAN_POINT('Ctrl Pts',(48.702007382895,-49.2958545728828,-1.43309953755765));
#41782=CARTESIAN_POINT('Ctrl Pts',(44.7495026483646,-50.0742379240769,-1.62896209536295));
#41783=CARTESIAN_POINT('Ctrl Pts',(41.9142778931429,-47.2125003909646,-1.82482465316824));
#41784=CARTESIAN_POINT('Ctrl Pts',(42.7294848407124,-43.2674137033876,-2.02068721097353));
#41785=CARTESIAN_POINT('Ctrl Pts',(46.4667736250309,-41.7638010108231,-2.21654976877883));
#41786=CARTESIAN_POINT('Ctrl Pts',(49.7870170832974,-44.045063177084,-2.41241232658412));
#41787=CARTESIAN_POINT('Ctrl Pts',(49.7237066049375,-48.0729894833012,-2.60827488438941));
#41788=CARTESIAN_POINT('Ctrl Pts',(46.3334069399903,-50.2487777183904,-2.80413744219471));
#41789=CARTESIAN_POINT('Ctrl Pts',(42.6452210871736,-48.6284468638715,-3.));
#41790=CARTESIAN_POINT('Ctrl Pts',(41.9544013881446,-44.659699244384,-3.19586255780529));
#41791=CARTESIAN_POINT('Ctrl Pts',(44.8781688180426,-41.8884590913979,-3.39172511561059));
#41792=CARTESIAN_POINT('Ctrl Pts',(48.8042493424128,-42.7907228633015,-3.58758767341588));
#41793=CARTESIAN_POINT('Ctrl Pts',(50.2248407055034,-46.5603526363256,-3.78345023122117));
#41794=CARTESIAN_POINT('Ctrl Pts',(47.8706990326452,-49.8293288126631,-3.97931278902647));
#41795=CARTESIAN_POINT('Ctrl Pts',(43.8451595681529,-49.6769466642923,-4.17517534683176));
#41796=CARTESIAN_POINT('Ctrl Pts',(41.7448873316061,-46.2393537773645,-4.37103790463705));
#41797=CARTESIAN_POINT('Ctrl Pts',(43.4463949656544,-42.5879074788031,-4.56690046244235));
#41798=CARTESIAN_POINT('Ctrl Pts',(47.4294506962584,-41.9850348994753,-4.76276302024764));
#41799=CARTESIAN_POINT('Ctrl Pts',(50.1353470904784,-44.9693795557798,-4.95862557805293));
#41800=CARTESIAN_POINT('Ctrl Pts',(49.1464695579982,-48.8745440241578,-5.15448813585823));
#41801=CARTESIAN_POINT('Ctrl Pts',(45.3463422376812,-50.211413728628,-5.35035069366352));
#41802=CARTESIAN_POINT('Ctrl Pts',(42.1302330232793,-47.7855468799332,-5.54621325146881));
#41803=CARTESIAN_POINT('Ctrl Pts',(42.3716121306267,-43.7643624369532,-5.74207580927411));
#41804=CARTESIAN_POINT('Ctrl Pts',(45.8548164718352,-41.7406343210637,-5.9379383670794));
#41805=CARTESIAN_POINT('Ctrl Pts',(49.4677368869436,-43.5224860539098,-6.1338009248847));
#41806=CARTESIAN_POINT('Ctrl Pts',(49.9823671421591,-47.5179012592972,-6.32966348268999));
#41807=CARTESIAN_POINT('Ctrl Pts',(46.9389058700719,-50.157130265541,-6.52552604049529));
#41808=CARTESIAN_POINT('Ctrl Pts',(43.0565668419507,-49.0821222582622,-6.72138859830057));
#41809=CARTESIAN_POINT('Ctrl Pts',(41.8040752283821,-45.2533576466263,-6.91725115610587));
#41810=CARTESIAN_POINT('Ctrl Pts',(44.3004755476465,-42.0916865643329,-7.11311371391116));
#41811=CARTESIAN_POINT('Ctrl Pts',(48.3153476427955,-42.4219491862816,-7.30897627171646));
#41812=CARTESIAN_POINT('Ctrl Pts',(50.2615211515669,-45.949051367223,-7.50483882952175));
#41813=CARTESIAN_POINT('Ctrl Pts',(48.4002387735869,-49.5216977571311,-7.70070138732704));
#41814=CARTESIAN_POINT('Ctrl Pts',(44.3943335491657,-49.9477941977075,-7.89656394513234));
#41815=CARTESIAN_POINT('Ctrl Pts',(41.8232373740198,-46.8467864558395,-8.09242650293763));
#41816=CARTESIAN_POINT('Ctrl Pts',(42.9834937963114,-42.989006334733,-8.28828906074292));
#41817=CARTESIAN_POINT('Ctrl Pts',(46.8397504745972,-41.8218446822126,-8.48415161854822));
#41818=CARTESIAN_POINT('Ctrl Pts',(49.9439484107626,-44.386863933193,-8.68001417635351));
#41819=CARTESIAN_POINT('Ctrl Pts',(49.5280211699711,-48.3948728544126,-8.8758767341588));
#41820=CARTESIAN_POINT('Ctrl Pts',(45.9524450920796,-50.2596030398939,-9.07173929196411));
#41821=CARTESIAN_POINT('Ctrl Pts',(43.6105151899593,-48.9695264621503,-9.20231433050096));
#41822=CARTESIAN_POINT('Ctrl Pts',(42.963068816724,-47.9728941274296,-9.2676018497694));
#41823=CARTESIAN_POINT('Ctrl Pts',(48.9250875598184,-43.4917339993741,0.267601849769391));
#41824=CARTESIAN_POINT('Ctrl Pts',(49.7482273840168,-44.45166251539,0.20231433050096));
#41825=CARTESIAN_POINT('Ctrl Pts',(50.3625541761304,-47.2293903822839,0.071739291964098));
#41826=CARTESIAN_POINT('Ctrl Pts',(47.3862821539145,-50.3199663185471,-0.124123265841196));
#41827=CARTESIAN_POINT('Ctrl Pts',(43.17004382434,-49.5420991574348,-0.319985823646489));
#41828=CARTESIAN_POINT('Ctrl Pts',(41.482920472032,-45.6037338905227,-0.515848381451783));
#41829=CARTESIAN_POINT('Ctrl Pts',(43.8313084972421,-42.0173541629913,-0.711710939257076));
#41830=CARTESIAN_POINT('Ctrl Pts',(48.1174985652505,-41.9903248019207,-0.907573497062369));
#41831=CARTESIAN_POINT('Ctrl Pts',(50.511706922499,-45.5452926394177,-1.10343605486766));
#41832=CARTESIAN_POINT('Ctrl Pts',(48.8749164567556,-49.5067656034683,-1.29929861267296));
#41833=CARTESIAN_POINT('Ctrl Pts',(44.6694797956125,-50.3349599008559,-1.49516117047825));
#41834=CARTESIAN_POINT('Ctrl Pts',(41.652821011115,-47.290091711027,-1.69102372828354));
#41835=CARTESIAN_POINT('Ctrl Pts',(42.5201953506765,-43.0925477985858,-1.88688628608884));
#41836=CARTESIAN_POINT('Ctrl Pts',(46.4966437859037,-41.4927146886523,-2.08274884389413));
#41837=CARTESIAN_POINT('Ctrl Pts',(50.0293589883241,-43.9199612555844,-2.27861140169942));
#41838=CARTESIAN_POINT('Ctrl Pts',(49.961997093877,-48.2056459275246,-2.47447395950472));
#41839=CARTESIAN_POINT('Ctrl Pts',(46.354742590506,-50.5206689889239,-2.67033651731001));
#41840=CARTESIAN_POINT('Ctrl Pts',(42.4305393218699,-48.7966485926308,-2.8661990751153));
#41841=CARTESIAN_POINT('Ctrl Pts',(41.6955121217363,-44.5739296185069,-3.0620616329206));
#41842=CARTESIAN_POINT('Ctrl Pts',(44.8063796764111,-41.6253499914204,-3.25792419072589));
#41843=CARTESIAN_POINT('Ctrl Pts',(48.983701167652,-42.5853521670624,-3.45378674853119));
#41844=CARTESIAN_POINT('Ctrl Pts',(50.4952001790642,-46.5962111820853,-3.64964930633648));
#41845=CARTESIAN_POINT('Ctrl Pts',(47.9904103403397,-50.0743783645986,-3.84551186414178));
#41846=CARTESIAN_POINT('Ctrl Pts',(43.7072652508588,-49.9122448527363,-4.04137442194706));
#41847=CARTESIAN_POINT('Ctrl Pts',(41.4725906697532,-46.2546707007123,-4.23723697975236));
#41848=CARTESIAN_POINT('Ctrl Pts',(43.2829825766694,-42.3695580540379,-4.43309953755765));
#41849=CARTESIAN_POINT('Ctrl Pts',(47.5209252782984,-41.7281059578637,-4.62896209536295));
#41850=CARTESIAN_POINT('Ctrl Pts',(50.3999796151832,-44.9034272465301,-4.82482465316824));
#41851=CARTESIAN_POINT('Ctrl Pts',(49.3478210201178,-49.058494204359,-5.02068721097353));
#41852=CARTESIAN_POINT('Ctrl Pts',(45.3045128337278,-50.4809139720657,-5.21654976877883));
#41853=CARTESIAN_POINT('Ctrl Pts',(41.8825957191635,-47.8998090611908,-5.41241232658412));
#41854=CARTESIAN_POINT('Ctrl Pts',(42.1394213564373,-43.6212976833329,-5.60827488438942));
#41855=CARTESIAN_POINT('Ctrl Pts',(45.8455257683553,-41.4680654970699,-5.80413744219471));
#41856=CARTESIAN_POINT('Ctrl Pts',(49.6896471516265,-43.3639429482889,-6.));
#41857=CARTESIAN_POINT('Ctrl Pts',(50.2372100484674,-47.6150360423544,-6.19586255780529));
#41858=CARTESIAN_POINT('Ctrl Pts',(46.9989891050268,-50.4231567570609,-6.39172511561059));
#41859=CARTESIAN_POINT('Ctrl Pts',(42.8682082517594,-49.2793559551702,-6.58758767341588));
#41860=CARTESIAN_POINT('Ctrl Pts',(41.5355661669926,-45.2055778964139,-6.78345023122117));
#41861=CARTESIAN_POINT('Ctrl Pts',(44.1917181841692,-41.8415825635829,-6.97931278902647));
#41862=CARTESIAN_POINT('Ctrl Pts',(48.4635132692535,-42.1929796222669,-7.17517534683176));
#41863=CARTESIAN_POINT('Ctrl Pts',(50.5342279103342,-45.9457910205032,-7.37103790463706));
#41864=CARTESIAN_POINT('Ctrl Pts',(48.5538368229528,-49.7470611301022,-7.56690046244235));
#41865=CARTESIAN_POINT('Ctrl Pts',(44.2915824239466,-50.200424683782,-7.76276302024764));
#41866=CARTESIAN_POINT('Ctrl Pts',(41.5559545523793,-46.9009747096407,-7.95862557805294));
#41867=CARTESIAN_POINT('Ctrl Pts',(42.7904590558158,-42.79632435712,-8.15448813585823));
#41868=CARTESIAN_POINT('Ctrl Pts',(46.8934884761126,-41.554472738295,-8.35035069366352));
#41869=CARTESIAN_POINT('Ctrl Pts',(50.1963327940828,-44.2836348061786,-8.54621325146883));
#41870=CARTESIAN_POINT('Ctrl Pts',(49.753789195966,-48.5481275234752,-8.7420758092741));
#41871=CARTESIAN_POINT('Ctrl Pts',(45.9494019193858,-50.5321870532849,-8.93793836707941));
#41872=CARTESIAN_POINT('Ctrl Pts',(43.4576053170538,-49.1595548364713,-9.06851340561627));
#41873=CARTESIAN_POINT('Ctrl Pts',(42.7687270241728,-48.0991451874963,-9.1338009248847));
#41874=CARTESIAN_POINT('Ctrl Pts',(49.1010141262202,-43.3408767631073,0.401402774654087));
#41875=CARTESIAN_POINT('Ctrl Pts',(49.9736609002034,-44.3585392526745,0.336115255385656));
#41876=CARTESIAN_POINT('Ctrl Pts',(50.6249357839467,-47.303330879551,0.205540216848794));
#41877=CARTESIAN_POINT('Ctrl Pts',(47.469658755269,-50.579786520798,0.00967765904349996));
#41878=CARTESIAN_POINT('Ctrl Pts',(42.999838843166,-49.7551352905006,-0.186184898761793));
#41879=CARTESIAN_POINT('Ctrl Pts',(41.2112450861611,-45.5799008480595,-0.382047456567087));
#41880=CARTESIAN_POINT('Ctrl Pts',(43.700874641208,-41.7778217753375,-0.577910014372381));
#41881=CARTESIAN_POINT('Ctrl Pts',(48.2448534714975,-41.7491667594488,-0.773772572177674));
#41882=CARTESIAN_POINT('Ctrl Pts',(50.7830591782025,-45.5179447043461,-0.969635129982967));
#41883=CARTESIAN_POINT('Ctrl Pts',(49.0478255306161,-49.7176766340539,-1.16549768778826));
#41884=CARTESIAN_POINT('Ctrl Pts',(44.5894569428605,-50.5956818776348,-1.36136024559355));
#41885=CARTESIAN_POINT('Ctrl Pts',(41.3913641290871,-47.3676830310895,-1.55722280339885));
#41886=CARTESIAN_POINT('Ctrl Pts',(42.3109058606407,-42.9176818937838,-1.75308536120414));
#41887=CARTESIAN_POINT('Ctrl Pts',(46.5265139467765,-41.2216283664815,-1.94894791900943));
#41888=CARTESIAN_POINT('Ctrl Pts',(50.2717008933508,-43.7948593340848,-2.14481047681473));
#41889=CARTESIAN_POINT('Ctrl Pts',(50.2002875828164,-48.338302371748,-2.34067303462002));
#41890=CARTESIAN_POINT('Ctrl Pts',(46.3760782410217,-50.7925602594573,-2.53653559242531));
#41891=CARTESIAN_POINT('Ctrl Pts',(42.2158575565662,-48.9648503213903,-2.73239815023061));
#41892=CARTESIAN_POINT('Ctrl Pts',(41.436622855328,-44.4881599926298,-2.9282607080359));
#41893=CARTESIAN_POINT('Ctrl Pts',(44.7345905347796,-41.3622408914429,-3.12412326584119));
#41894=CARTESIAN_POINT('Ctrl Pts',(49.1631529928913,-42.3799814708233,-3.31998582364649));
#41895=CARTESIAN_POINT('Ctrl Pts',(50.765559652625,-46.6320697278449,-3.51584838145178));
#41896=CARTESIAN_POINT('Ctrl Pts',(48.1101216480341,-50.3194279165342,-3.71171093925708));
#41897=CARTESIAN_POINT('Ctrl Pts',(43.5693709335647,-50.1475430411802,-3.90757349706237));
#41898=CARTESIAN_POINT('Ctrl Pts',(41.2002940079003,-46.2699876240602,-4.10343605486767));
#41899=CARTESIAN_POINT('Ctrl Pts',(43.1195701876843,-42.1512086292726,-4.29929861267295));
#41900=CARTESIAN_POINT('Ctrl Pts',(47.6123998603384,-41.4711770162521,-4.49516117047826));
#41901=CARTESIAN_POINT('Ctrl Pts',(50.6646121398881,-44.8374749372802,-4.69102372828354));
#41902=CARTESIAN_POINT('Ctrl Pts',(49.5491724822373,-49.2424443845602,-4.88688628608884));
#41903=CARTESIAN_POINT('Ctrl Pts',(45.2626834297744,-50.7504142155033,-5.08274884389412));
#41904=CARTESIAN_POINT('Ctrl Pts',(41.6349584150478,-48.0140712424484,-5.27861140169943));
#41905=CARTESIAN_POINT('Ctrl Pts',(41.9072305822478,-43.4782329297126,-5.47447395950471));
#41906=CARTESIAN_POINT('Ctrl Pts',(45.8362350648755,-41.1954966730761,-5.67033651731001));
#41907=CARTESIAN_POINT('Ctrl Pts',(49.9115574163095,-43.2053998426678,-5.86619907511531));
#41908=CARTESIAN_POINT('Ctrl Pts',(50.4920529547756,-47.7121708254118,-6.0620616329206));
#41909=CARTESIAN_POINT('Ctrl Pts',(47.0590723399817,-50.6891832485807,-6.25792419072589));
#41910=CARTESIAN_POINT('Ctrl Pts',(42.679849661568,-49.4765896520782,-6.45378674853119));
#41911=CARTESIAN_POINT('Ctrl Pts',(41.267057105603,-45.1577981462014,-6.64964930633648));
#41912=CARTESIAN_POINT('Ctrl Pts',(44.0829608206919,-41.591478562833,-6.84551186414177));
#41913=CARTESIAN_POINT('Ctrl Pts',(48.6116788957116,-41.9640100582522,-7.04137442194706));
#41914=CARTESIAN_POINT('Ctrl Pts',(50.8069346691015,-45.9425306737833,-7.23723697975236));
#41915=CARTESIAN_POINT('Ctrl Pts',(48.7074348723187,-49.9724245030734,-7.43309953755765));
#41916=CARTESIAN_POINT('Ctrl Pts',(44.1888312987275,-50.4530551698565,-7.62896209536294));
#41917=CARTESIAN_POINT('Ctrl Pts',(41.2886717307389,-46.9551629634418,-7.82482465316825));
#41918=CARTESIAN_POINT('Ctrl Pts',(42.5974243153202,-42.603642379507,-8.02068721097353));
#41919=CARTESIAN_POINT('Ctrl Pts',(46.947226477628,-41.2871007943775,-8.21654976877883));
#41920=CARTESIAN_POINT('Ctrl Pts',(50.4487171774031,-44.1804056791643,-8.41241232658412));
#41921=CARTESIAN_POINT('Ctrl Pts',(49.979557221961,-48.7013821925377,-8.60827488438941));
#41922=CARTESIAN_POINT('Ctrl Pts',(45.946358746692,-50.8047710666759,-8.80413744219471));
#41923=CARTESIAN_POINT('Ctrl Pts',(43.3046954441484,-49.3495832107922,-8.93471248073157));
#41924=CARTESIAN_POINT('Ctrl Pts',(42.5743852316216,-48.2253962475631,-9.));
#41925=CARTESIAN_POINT('Ctrl Pts',(48.5732344270147,-43.7934484719077,0.));
#41926=CARTESIAN_POINT('Ctrl Pts',(48.6498724033581,-43.8663851681741,3.87614628204605E-17));
#41927=CARTESIAN_POINT('Ctrl Pts',(48.7225776093513,-43.942957995891,-1.95539500540648E-17));
#41928=CARTESIAN_POINT('Ctrl Pts',(48.7913525374548,-44.022751380685,4.85722573273506E-17));
#41929=CARTESIAN_POINT('Ctrl Pts',(48.8618446331577,-44.1045370411351,1.1839943509454E-16));
#41930=CARTESIAN_POINT('Ctrl Pts',(48.9282081375236,-44.1897064969362,3.17350500352468E-16));
#41931=CARTESIAN_POINT('Ctrl Pts',(48.9904195836878,-44.2778605693834,3.05311331771918E-16));
#41932=CARTESIAN_POINT('Ctrl Pts',(49.0539465298674,-44.3678787149361,2.9301758742712E-16));
#41933=CARTESIAN_POINT('Ctrl Pts',(49.1131444138394,-44.4610095732985,3.8989011672772E-16));
#41934=CARTESIAN_POINT('Ctrl Pts',(49.1679548280974,-44.5568705359006,3.67761376907083E-16));
#41935=CARTESIAN_POINT('Ctrl Pts',(49.2206156820432,-44.6489720136768,3.4650048421955E-16));
#41936=CARTESIAN_POINT('Ctrl Pts',(49.2692265344368,-44.7435944760072,-5.92281301081711E-19));
#41937=CARTESIAN_POINT('Ctrl Pts',(49.3137017428961,-44.8404267203043,2.77555756156289E-17));
#41938=CARTESIAN_POINT('Ctrl Pts',(49.3201147960405,-44.8543893379128,3.18431632680741E-17));
#41939=CARTESIAN_POINT('Ctrl Pts',(49.3264418005973,-44.8683979386779,1.52397213062401E-16));
#41940=CARTESIAN_POINT('Ctrl Pts',(49.3326824371613,-44.8824516252654,1.66533453693773E-16));
#41941=CARTESIAN_POINT('Ctrl Pts',(49.3392327263543,-44.8972026383122,1.81371117013511E-16));
#41942=CARTESIAN_POINT('Ctrl Pts',(49.345684301834,-44.9119953356503,-6.93889390390723E-17));
#41943=CARTESIAN_POINT('Ctrl Pts',(49.3520358333759,-44.9268254977065,-6.93889390390723E-17));
#41944=CARTESIAN_POINT('Ctrl Pts',(49.3968932976766,-45.0315629867066,-6.93889390390723E-17));
#41945=CARTESIAN_POINT('Ctrl Pts',(49.4367846336838,-45.1382131707156,-9.08116252949891E-17));
#41946=CARTESIAN_POINT('Ctrl Pts',(49.4716807095004,-45.2463465785723,-1.2490009027033E-16));
#41947=CARTESIAN_POINT('Ctrl Pts',(49.5070983411891,-45.3560961456251,-1.59498040586468E-16));
#41948=CARTESIAN_POINT('Ctrl Pts',(49.5373707252924,-45.4673743159336,1.38995551510238E-16));
#41949=CARTESIAN_POINT('Ctrl Pts',(49.5624277251463,-45.5797685483207,1.2490009027033E-16));
#41950=CARTESIAN_POINT('Ctrl Pts',(49.5887043183169,-45.6976333181011,1.10118564041589E-16));
#41951=CARTESIAN_POINT('Ctrl Pts',(49.6092463289301,-45.8167261990927,-1.8576267690903E-16));
#41952=CARTESIAN_POINT('Ctrl Pts',(49.6239191637252,-45.9366000763245,-2.22044604925031E-16));
#41953=CARTESIAN_POINT('Ctrl Pts',(49.6349237898216,-46.0265054842483,-2.49256050937032E-16));
#41954=CARTESIAN_POINT('Ctrl Pts',(49.6426259276078,-46.1168509125721,-3.71444925944582E-16));
#41955=CARTESIAN_POINT('Ctrl Pts',(49.6469460860109,-46.2074531754375,-3.88578058618805E-16));
#41956=CARTESIAN_POINT('Ctrl Pts',(49.6478995072093,-46.2274483029239,-3.92359191244283E-16));
#41957=CARTESIAN_POINT('Ctrl Pts',(49.6486881115146,-46.2474583007511,3.11387392686402E-18));
#41958=CARTESIAN_POINT('Ctrl Pts',(49.6493104445425,-46.2674574556759,0.));
#41959=CARTESIAN_POINT('Ctrl Pts',(49.6529983798999,-46.3859721210812,-1.84527660266109E-17));
#41960=CARTESIAN_POINT('Ctrl Pts',(49.6508611272068,-46.5042818926988,-4.93086514076101E-16));
#41961=CARTESIAN_POINT('Ctrl Pts',(49.6428326820612,-46.6219591778934,-5.27355936696949E-16));
#41962=CARTESIAN_POINT('Ctrl Pts',(49.6348301571772,-46.7392565357239,-5.61514718667094E-16));
#41963=CARTESIAN_POINT('Ctrl Pts',(49.6209747430515,-46.8559263686311,3.35081433764176E-17));
#41964=CARTESIAN_POINT('Ctrl Pts',(49.6011528370971,-46.9715627523068,1.11022302462516E-16));
#41965=CARTESIAN_POINT('Ctrl Pts',(49.5985997294166,-46.9864569880065,1.21006306794016E-16));
#41966=CARTESIAN_POINT('Ctrl Pts',(49.5959475676709,-47.0013340919922,-3.9670406639623E-16));
#41967=CARTESIAN_POINT('Ctrl Pts',(49.5931960463113,-47.0161932062988,-4.16333634234434E-16));
#41968=CARTESIAN_POINT('Ctrl Pts',(49.5723030878064,-47.1290220082781,-5.94426135246255E-16));
#41969=CARTESIAN_POINT('Ctrl Pts',(49.5456857086921,-47.2408138147752,-1.38518759257453E-16));
#41970=CARTESIAN_POINT('Ctrl Pts',(49.5136421664862,-47.35130678912,-8.32667268468867E-17));
#41971=CARTESIAN_POINT('Ctrl Pts',(49.4934325244267,-47.4209939493983,-4.84196493640788E-17));
#41972=CARTESIAN_POINT('Ctrl Pts',(49.4710634035422,-47.4901644562924,-3.44816612477604E-16));
#41973=CARTESIAN_POINT('Ctrl Pts',(49.4465992519874,-47.5587510924403,-3.88578058618805E-16));
#41974=CARTESIAN_POINT('Ctrl Pts',(49.4379571492393,-47.5829797175535,-4.04037042066843E-16));
#41975=CARTESIAN_POINT('Ctrl Pts',(49.4290535388707,-47.6071354647896,-6.52106218683356E-16));
#41976=CARTESIAN_POINT('Ctrl Pts',(49.4198910389393,-47.6312153075406,-6.66133814775094E-16));
#41977=CARTESIAN_POINT('Ctrl Pts',(49.4140168574915,-47.646653164743,-6.75127063925236E-16));
#41978=CARTESIAN_POINT('Ctrl Pts',(49.4080376321108,-47.6620561076285,5.84477223823245E-17));
#41979=CARTESIAN_POINT('Ctrl Pts',(49.4019578356655,-47.6774144897037,5.55111512312578E-17));
#41980=CARTESIAN_POINT('Ctrl Pts',(49.3590826893517,-47.7857228655749,3.48022477513383E-17));
#41981=CARTESIAN_POINT('Ctrl Pts',(49.311160597646,-47.8919462670934,-4.80329790939922E-16));
#41982=CARTESIAN_POINT('Ctrl Pts',(49.2585457221187,-47.99582861299,-4.44089209850063E-16));
#41983=CARTESIAN_POINT('Ctrl Pts',(49.2040866933149,-48.1033520388407,-4.06578395091634E-16));
#41984=CARTESIAN_POINT('Ctrl Pts',(49.1446000346224,-48.2083681046694,-4.35125637352618E-16));
#41985=CARTESIAN_POINT('Ctrl Pts',(49.0804225521245,-48.3105894369623,-6.10622663543836E-16));
#41986=CARTESIAN_POINT('Ctrl Pts',(49.0155495073654,-48.4139186547353,-7.88021744842209E-16));
#41987=CARTESIAN_POINT('Ctrl Pts',(48.9458830288196,-48.5143929921466,2.12533168780725E-16));
#41988=CARTESIAN_POINT('Ctrl Pts',(48.8717189601,-48.6117011858697,3.88578058618805E-16));
#41989=CARTESIAN_POINT('Ctrl Pts',(48.819020255279,-48.680845393654,5.13670139528005E-16));
#41990=CARTESIAN_POINT('Ctrl Pts',(48.7640495726607,-48.7483907131672,2.85916815352541E-16));
#41991=CARTESIAN_POINT('Ctrl Pts',(48.7068990197081,-48.8142178472156,3.33066907387547E-16));
#41992=CARTESIAN_POINT('Ctrl Pts',(48.6896326846016,-48.8341055525284,3.47311901483314E-16));
#41993=CARTESIAN_POINT('Ctrl Pts',(48.6721673038657,-48.8538363742111,-2.93254321078155E-16));
#41994=CARTESIAN_POINT('Ctrl Pts',(48.6545052298657,-48.8734068741477,-2.77555756156289E-16));
#41995=CARTESIAN_POINT('Ctrl Pts',(48.6371213308794,-48.8926691416486,-2.62104441274986E-16));
#41996=CARTESIAN_POINT('Ctrl Pts',(48.6195431892455,-48.9117798961928,2.3663751342404E-16));
#41997=CARTESIAN_POINT('Ctrl Pts',(48.6017947545563,-48.9307129811787,2.22044604925031E-16));
#41998=CARTESIAN_POINT('Ctrl Pts',(48.5161347739284,-49.0220904869426,1.51614266632079E-16));
#41999=CARTESIAN_POINT('Ctrl Pts',(48.4264328955782,-49.1094220783965,-1.89444256750939E-16));
#42000=CARTESIAN_POINT('Ctrl Pts',(48.3330184543456,-49.1923915218619,-3.33066907387547E-16));
#42001=CARTESIAN_POINT('Ctrl Pts',(48.2522204472863,-49.2641552191059,-4.57292067725676E-16));
#42002=CARTESIAN_POINT('Ctrl Pts',(48.1686439750736,-49.3326555431842,-7.0435694103298E-16));
#42003=CARTESIAN_POINT('Ctrl Pts',(48.0824754422125,-49.3976719692188,-6.66133814775094E-16));
#42004=CARTESIAN_POINT('Ctrl Pts',(48.0430744318381,-49.4274010685969,-6.48656091246299E-16));
#42005=CARTESIAN_POINT('Ctrl Pts',(48.0031311516611,-49.4564015054461,-5.92672758068129E-16));
#42006=CARTESIAN_POINT('Ctrl Pts',(47.9626619300835,-49.4846508230087,-6.66133814775094E-16));
#42007=CARTESIAN_POINT('Ctrl Pts',(47.944142628871,-49.4975781193735,-6.99750656995116E-16));
#42008=CARTESIAN_POINT('Ctrl Pts',(47.9255112318031,-49.5103494157158,-7.97651143721192E-16));
#42009=CARTESIAN_POINT('Ctrl Pts',(47.9067755363185,-49.522958267244,-7.7715611723761E-16));
#42010=CARTESIAN_POINT('Ctrl Pts',(47.8018201646528,-49.5935917112763,-6.62345160598864E-16));
#42011=CARTESIAN_POINT('Ctrl Pts',(47.6937577817196,-49.659022014658,-1.03399818926308E-15));
#42012=CARTESIAN_POINT('Ctrl Pts',(47.5828994522725,-49.7189169737277,-9.43689570931383E-16));
#42013=CARTESIAN_POINT('Ctrl Pts',(47.4730678387123,-49.7782572148403,-8.54217347064921E-16));
#42014=CARTESIAN_POINT('Ctrl Pts',(47.360491247089,-49.8321648668083,-3.07975410823444E-16));
#42015=CARTESIAN_POINT('Ctrl Pts',(47.2454367515685,-49.8802809428291,-5.55111512312578E-17));
#42016=CARTESIAN_POINT('Ctrl Pts',(47.1845210132458,-49.9057560560156,2.0809105445999E-17));
#42017=CARTESIAN_POINT('Ctrl Pts',(47.122910127501,-49.9296070150102,-3.22723620147229E-16));
#42018=CARTESIAN_POINT('Ctrl Pts',(47.0606641786102,-49.9518499819597,-2.77555756156289E-16));
#42019=CARTESIAN_POINT('Ctrl Pts',(42.6120197259946,-46.0027475428216,-2.01601780324957));
#42020=CARTESIAN_POINT('Ctrl Pts',(42.6094248952187,-46.3290880655303,-1.99688706151736));
#42021=CARTESIAN_POINT('Ctrl Pts',(42.6528675733331,-46.654752224773,-1.97775631978515));
#42022=CARTESIAN_POINT('Ctrl Pts',(42.7452064887581,-46.965905306516,-1.95862557805294));
#42023=CARTESIAN_POINT('Ctrl Pts',(43.0603316838194,-48.0277780297008,-1.8933380587845));
#42024=CARTESIAN_POINT('Ctrl Pts',(43.944928592468,-48.9206469884994,-1.82805053951607));
#42025=CARTESIAN_POINT('Ctrl Pts',(45.0038225147786,-49.245652733732,-1.76276302024764));
#42026=CARTESIAN_POINT('Ctrl Pts',(46.0627164370892,-49.5706584789645,-1.69747550097921));
#42027=CARTESIAN_POINT('Ctrl Pts',(47.2959073730619,-49.3278010106308,-1.63218798171078));
#42028=CARTESIAN_POINT('Ctrl Pts',(48.1524868580578,-48.6255464376747,-1.56690046244235));
#42029=CARTESIAN_POINT('Ctrl Pts',(49.0090663430538,-47.9232918647185,-1.50161294317392));
#42030=CARTESIAN_POINT('Ctrl Pts',(49.489034377073,-46.7616401871398,-1.43632542390549));
#42031=CARTESIAN_POINT('Ctrl Pts',(49.3779827843599,-45.6595897445677,-1.37103790463706));
#42032=CARTESIAN_POINT('Ctrl Pts',(49.2669311916469,-44.5575393019956,-1.30575038536862));
#42033=CARTESIAN_POINT('Ctrl Pts',(48.5648599722015,-43.51509009443,-1.24046286610019));
#42034=CARTESIAN_POINT('Ctrl Pts',(47.5853889385713,-42.9978284992196,-1.17517534683176));
#42035=CARTESIAN_POINT('Ctrl Pts',(46.605917904941,-42.4805669040093,-1.10988782756333));
#42036=CARTESIAN_POINT('Ctrl Pts',(45.3490470571259,-42.488492921154,-1.0446003082949));
#42037=CARTESIAN_POINT('Ctrl Pts',(44.3762941389621,-43.0182861025848,-0.979312789026468));
#42038=CARTESIAN_POINT('Ctrl Pts',(43.4035412207983,-43.5480792840155,-0.914025269758037));
#42039=CARTESIAN_POINT('Ctrl Pts',(42.7149062322859,-44.5997396297324,-0.848737750489605));
#42040=CARTESIAN_POINT('Ctrl Pts',(42.6179524951822,-45.7030076218998,-0.783450231221174));
#42041=CARTESIAN_POINT('Ctrl Pts',(42.6093232857121,-45.8012021927373,-0.777639421897305));
#42042=CARTESIAN_POINT('Ctrl Pts',(42.6053811385124,-45.8998055787131,-0.771828612573435));
#42043=CARTESIAN_POINT('Ctrl Pts',(42.6059703323355,-45.9984546826137,-0.766017803249566));
#42044=CARTESIAN_POINT('Ctrl Pts',(44.942095577027,-49.9456385074984,5.55111512312578E-16));
#42045=CARTESIAN_POINT('Ctrl Pts',(43.6472519732776,-49.5984650974504,-0.0652875192684306));
#42046=CARTESIAN_POINT('Ctrl Pts',(41.4469671882449,-47.5357720342741,-0.195862557805293));
#42047=CARTESIAN_POINT('Ctrl Pts',(42.2010820840665,-43.0499891012353,-0.391725115610587));
#42048=CARTESIAN_POINT('Ctrl Pts',(46.3558078226787,-41.2067330502749,-0.58758767341588));
#42049=CARTESIAN_POINT('Ctrl Pts',(50.1895243958238,-43.6427681215851,-0.783450231221173));
#42050=CARTESIAN_POINT('Ctrl Pts',(50.2815817385072,-48.1865095580738,-0.979312789026466));
#42051=CARTESIAN_POINT('Ctrl Pts',(46.547466535547,-50.7759010051096,-1.17517534683176));
#42052=CARTESIAN_POINT('Ctrl Pts',(42.3245747925301,-49.0985935082275,-1.37103790463705));
#42053=CARTESIAN_POINT('Ctrl Pts',(41.3853564274817,-44.6526231071457,-1.56690046244235));
#42054=CARTESIAN_POINT('Ctrl Pts',(44.5692320816632,-41.4105744865513,-1.76276302024764));
#42055=CARTESIAN_POINT('Ctrl Pts',(49.0314013549138,-42.268956305567,-1.95862557805293));
#42056=CARTESIAN_POINT('Ctrl Pts',(50.7851507003408,-46.4609045572623,-2.15448813585823));
#42057=CARTESIAN_POINT('Ctrl Pts',(48.263541336862,-50.2410414729541,-2.35035069366352));
#42058=CARTESIAN_POINT('Ctrl Pts',(43.7195496474102,-50.2319758772438,-2.54621325146881));
#42059=CARTESIAN_POINT('Ctrl Pts',(41.2130503891591,-46.4417996610074,-2.74207580927411));
#42060=CARTESIAN_POINT('Ctrl Pts',(42.9835080927057,-42.2568936678579,-2.9379383670794));
#42061=CARTESIAN_POINT('Ctrl Pts',(47.4490849663269,-41.4163089133544,-3.13380092488469));
#42062=CARTESIAN_POINT('Ctrl Pts',(50.6199603203723,-44.6710765381374,-3.32966348268999));
#42063=CARTESIAN_POINT('Ctrl Pts',(49.6630782896489,-49.1131861274939,-3.52552604049528));
#42064=CARTESIAN_POINT('Ctrl Pts',(45.433376454472,-50.7737834599584,-3.72138859830057));
#42065=CARTESIAN_POINT('Ctrl Pts',(41.7099309782434,-48.1691884401856,-3.91725115610587));
#42066=CARTESIAN_POINT('Ctrl Pts',(41.8194975483498,-43.6265068139424,-4.11311371391116));
#42067=CARTESIAN_POINT('Ctrl Pts',(45.6641826146291,-41.204450252827,-4.30897627171645));
#42068=CARTESIAN_POINT('Ctrl Pts',(49.8089076312337,-43.0670333548852,-4.50483882952175));
#42069=CARTESIAN_POINT('Ctrl Pts',(50.5505198521649,-47.5501095932216,-4.70070138732704));
#42070=CARTESIAN_POINT('Ctrl Pts',(47.2264172239299,-50.6482223997432,-4.89656394513234));
#42071=CARTESIAN_POINT('Ctrl Pts',(42.8065578694184,-49.5933268780552,-5.09242650293763));
#42072=CARTESIAN_POINT('Ctrl Pts',(41.2399165089103,-45.3279316921833,-5.28828906074292));
#42073=CARTESIAN_POINT('Ctrl Pts',(43.9262270571184,-41.6630037489246,-5.48415161854821));
#42074=CARTESIAN_POINT('Ctrl Pts',(48.4653741677054,-41.8730155103115,-5.68001417635351));
#42075=CARTESIAN_POINT('Ctrl Pts',(50.8018040255352,-45.7703295385275,-5.8758767341588));
#42076=CARTESIAN_POINT('Ctrl Pts',(48.8480063650781,-49.8728452943253,-6.0717392919641));
#42077=CARTESIAN_POINT('Ctrl Pts',(44.349624114825,-50.5151224407608,-6.26760184976939));
#42078=CARTESIAN_POINT('Ctrl Pts',(41.3257897924298,-47.1233108990577,-6.46346440757468));
#42079=CARTESIAN_POINT('Ctrl Pts',(42.4781820663993,-42.7278643121404,-6.65932696537998));
#42080=CARTESIAN_POINT('Ctrl Pts',(46.777185224748,-41.255945113868,-6.85518952318527));
#42081=CARTESIAN_POINT('Ctrl Pts',(50.3817996987672,-44.0226574502926,-7.05105208099057));
#42082=CARTESIAN_POINT('Ctrl Pts',(50.071451482069,-48.5560483299491,-7.24691463879586));
#42083=CARTESIAN_POINT('Ctrl Pts',(46.1234029447301,-50.8057104508671,-7.44277719660115));
#42084=CARTESIAN_POINT('Ctrl Pts',(42.0651286013526,-48.7616499517032,-7.63863975440644));
#42085=CARTESIAN_POINT('Ctrl Pts',(41.522449548134,-44.2501709386981,-7.83450231221174));
#42086=CARTESIAN_POINT('Ctrl Pts',(44.9804152684286,-41.3020771440901,-8.03036487001703));
#42087=CARTESIAN_POINT('Ctrl Pts',(49.3490847557137,-42.5514377898613,-8.22622742782233));
#42088=CARTESIAN_POINT('Ctrl Pts',(50.7259989091243,-46.8818733140433,-8.42208998562761));
#42089=CARTESIAN_POINT('Ctrl Pts',(47.8793446557761,-50.4245587866615,-8.61795254343292));
#42090=CARTESIAN_POINT('Ctrl Pts',(43.3557549422264,-50.0137233751776,-8.8138151012382));
#42091=CARTESIAN_POINT('Ctrl Pts',(41.1902146341594,-46.0175034104326,-9.0096776590435));
#42092=CARTESIAN_POINT('Ctrl Pts',(43.3312750455412,-42.0041758492615,-9.20554021684879));
#42093=CARTESIAN_POINT('Ctrl Pts',(46.3331931919405,-41.7135846407914,-9.33611525538566));
#42094=CARTESIAN_POINT('Ctrl Pts',(47.5707104172798,-42.2290460377978,-9.40140277465409));
#42095=CARTESIAN_POINT('Ctrl Pts',(45.0021125537771,-49.7217947561856,0.133800924884696));
#42096=CARTESIAN_POINT('Ctrl Pts',(43.780727947621,-49.3943171693393,0.0685134056162651));
#42097=CARTESIAN_POINT('Ctrl Pts',(41.7052696005152,-47.4486446979355,-0.0620616329205971));
#42098=CARTESIAN_POINT('Ctrl Pts',(42.4166020906803,-43.2173489606696,-0.257924190725891));
#42099=CARTESIAN_POINT('Ctrl Pts',(46.3356221524447,-41.4786644127225,-0.453786748531184));
#42100=CARTESIAN_POINT('Ctrl Pts',(49.9518445234292,-43.7764984735613,-0.649649306336477));
#42101=CARTESIAN_POINT('Ctrl Pts',(50.0386792739052,-48.0624646155809,-0.84551186414177));
#42102=CARTESIAN_POINT('Ctrl Pts',(46.5164076935365,-50.5049548464966,-1.04137442194706));
#42103=CARTESIAN_POINT('Ctrl Pts',(42.5330888174582,-48.9228042681952,-1.23723697975236));
#42104=CARTESIAN_POINT('Ctrl Pts',(41.6471541381135,-44.7290624204674,-1.43309953755765));
#42105=CARTESIAN_POINT('Ctrl Pts',(44.6504023301515,-41.6709415276141,-1.62896209536294));
#42106=CARTESIAN_POINT('Ctrl Pts',(48.8594240565046,-42.4806256755021,-1.82482465316824));
#42107=CARTESIAN_POINT('Ctrl Pts',(50.5136797885161,-46.434756544742,-2.02068721097353));
#42108=CARTESIAN_POINT('Ctrl Pts',(48.1351262316434,-50.0004389365142,-2.21654976877883));
#42109=CARTESIAN_POINT('Ctrl Pts',(43.8489240339983,-49.9918876496915,-2.41241232658412));
#42110=CARTESIAN_POINT('Ctrl Pts',(41.4846233566774,-46.4167355064324,-2.60827488438941));
#42111=CARTESIAN_POINT('Ctrl Pts',(43.1546395491354,-42.4692473747058,-2.8041374421947));
#42112=CARTESIAN_POINT('Ctrl Pts',(47.3668755560586,-41.6763506292247,-3.));
#42113=CARTESIAN_POINT('Ctrl Pts',(50.3578609802875,-44.7464689524058,-3.19586255780529));
#42114=CARTESIAN_POINT('Ctrl Pts',(49.4552647293978,-48.9365690197714,-3.39172511561059));
#42115=CARTESIAN_POINT('Ctrl Pts',(45.465522110941,-50.5029574338028,-3.58758767341588));
#42116=CARTESIAN_POINT('Ctrl Pts',(41.9533149429416,-48.0461261584199,-3.78345023122117));
#42117=CARTESIAN_POINT('Ctrl Pts',(42.0566655882934,-43.761159701548,-3.97931278902647));
#42118=CARTESIAN_POINT('Ctrl Pts',(45.6832341884503,-41.4765111228166,-4.17517534683176));
#42119=CARTESIAN_POINT('Ctrl Pts',(49.5928208886295,-43.2334262606392,-4.37103790463705));
#42120=CARTESIAN_POINT('Ctrl Pts',(50.2923600049827,-47.4621688592611,-4.56690046244235));
#42121=CARTESIAN_POINT('Ctrl Pts',(47.1568401880312,-50.3845196968936,-4.76276302024764));
#42122=CARTESIAN_POINT('Ctrl Pts',(42.9877280563859,-49.38947045113,-4.95862557805294));
#42123=CARTESIAN_POINT('Ctrl Pts',(41.5099653091698,-45.3660594352277,-5.15448813585822));
#42124=CARTESIAN_POINT('Ctrl Pts',(44.0438762320297,-41.9090499866692,-5.35035069366353));
#42125=CARTESIAN_POINT('Ctrl Pts',(48.3255086931973,-42.1071473721194,-5.54621325146881));
#42126=CARTESIAN_POINT('Ctrl Pts',(50.5293883381624,-45.7833591907788,-5.74207580927411));
#42127=CARTESIAN_POINT('Ctrl Pts',(48.6864334213556,-49.6531312436619,-5.93793836707939));
#42128=CARTESIAN_POINT('Ctrl Pts',(44.4432531506607,-50.258970757616,-6.1338009248847));
#42129=CARTESIAN_POINT('Ctrl Pts',(41.5909668341935,-47.0595832856289,-6.32966348268998));
#42130=CARTESIAN_POINT('Ctrl Pts',(42.6779816517388,-42.9134989377614,-6.52552604049528));
#42131=CARTESIAN_POINT('Ctrl Pts',(46.7330939944334,-41.5250845801742,-6.72138859830057));
#42132=CARTESIAN_POINT('Ctrl Pts',(50.1332116742411,-44.1348359413317,-6.91725115610587));
#42133=CARTESIAN_POINT('Ctrl Pts',(49.8404701158586,-48.4110387337518,-7.11311371391116));
#42134=CARTESIAN_POINT('Ctrl Pts',(46.1164020555156,-50.5330731443828,-7.30897627171646));
#42135=CARTESIAN_POINT('Ctrl Pts',(42.2883615136259,-48.6049761753734,-7.50483882952175));
#42136=CARTESIAN_POINT('Ctrl Pts',(41.7764696992283,-44.3494421467659,-7.70070138732704));
#42137=CARTESIAN_POINT('Ctrl Pts',(45.0382582945098,-41.5685994505422,-7.89656394513233));
#42138=CARTESIAN_POINT('Ctrl Pts',(49.1590846597194,-42.7470814354426,-8.09242650293763));
#42139=CARTESIAN_POINT('Ctrl Pts',(50.4578837935332,-46.8318429246848,-8.28828906074292));
#42140=CARTESIAN_POINT('Ctrl Pts',(47.7727257759778,-50.1735449558638,-8.48415161854821));
#42141=CARTESIAN_POINT('Ctrl Pts',(43.5057681104367,-49.7860170368184,-8.68001417635351));
#42142=CARTESIAN_POINT('Ctrl Pts',(41.4630831185005,-46.0165104078946,-8.8758767341588));
#42143=CARTESIAN_POINT('Ctrl Pts',(43.4826770059318,-42.2308667297838,-9.0717392919641));
#42144=CARTESIAN_POINT('Ctrl Pts',(46.3142904937196,-41.9567613261026,-9.20231433050096));
#42145=CARTESIAN_POINT('Ctrl Pts',(47.4816009584782,-42.4429795948945,-9.26760184976939));
#42146=CARTESIAN_POINT('Ctrl Pts',(45.0621295305272,-49.4979510048728,0.267601849769392));
#42147=CARTESIAN_POINT('Ctrl Pts',(43.9142039219644,-49.1901692412281,0.202314330500961));
#42148=CARTESIAN_POINT('Ctrl Pts',(41.9635720127856,-47.361517361597,0.0717392919640984));
#42149=CARTESIAN_POINT('Ctrl Pts',(42.6321220972942,-43.3847088201037,-0.124123265841195));
#42150=CARTESIAN_POINT('Ctrl Pts',(46.3154364822107,-41.7505957751702,-0.319985823646489));
#42151=CARTESIAN_POINT('Ctrl Pts',(49.7141646510345,-43.9102288255375,-0.515848381451781));
#42152=CARTESIAN_POINT('Ctrl Pts',(49.7957768093032,-47.938419673088,-0.711710939257075));
#42153=CARTESIAN_POINT('Ctrl Pts',(46.4853488515259,-50.2340086878835,-0.907573497062368));
#42154=CARTESIAN_POINT('Ctrl Pts',(42.7416028423862,-48.747015028163,-1.10343605486766));
#42155=CARTESIAN_POINT('Ctrl Pts',(41.9089518487454,-44.805501733789,-1.29929861267296));
#42156=CARTESIAN_POINT('Ctrl Pts',(44.7315725786397,-41.931308568677,-1.49516117047825));
#42157=CARTESIAN_POINT('Ctrl Pts',(48.6874467580956,-42.6922950454372,-1.69102372828354));
#42158=CARTESIAN_POINT('Ctrl Pts',(50.2422088766913,-46.4086085322216,-1.88688628608884));
#42159=CARTESIAN_POINT('Ctrl Pts',(48.0067111264249,-49.7598364000743,-2.08274884389413));
#42160=CARTESIAN_POINT('Ctrl Pts',(43.9782984205864,-49.7517994221391,-2.27861140169942));
#42161=CARTESIAN_POINT('Ctrl Pts',(41.7561963241958,-46.3916713518576,-2.47447395950472));
#42162=CARTESIAN_POINT('Ctrl Pts',(43.3257710055652,-42.6816010815537,-2.67033651731001));
#42163=CARTESIAN_POINT('Ctrl Pts',(47.2846661457903,-41.936392345095,-2.8661990751153));
#42164=CARTESIAN_POINT('Ctrl Pts',(50.0957616402027,-44.8218613666743,-3.0620616329206));
#42165=CARTESIAN_POINT('Ctrl Pts',(49.2474511691466,-48.7599519120487,-3.25792419072589));
#42166=CARTESIAN_POINT('Ctrl Pts',(45.4976677674101,-50.2321314076473,-3.45378674853118));
#42167=CARTESIAN_POINT('Ctrl Pts',(42.1966989076398,-47.9230638766541,-3.64964930633647));
#42168=CARTESIAN_POINT('Ctrl Pts',(42.2938336282371,-43.8958125891536,-3.84551186414177));
#42169=CARTESIAN_POINT('Ctrl Pts',(45.7022857622716,-41.7485719928062,-4.04137442194706));
#42170=CARTESIAN_POINT('Ctrl Pts',(49.3767341460252,-43.3998191663933,-4.23723697975236));
#42171=CARTESIAN_POINT('Ctrl Pts',(50.0342001578005,-47.3742281253005,-4.43309953755765));
#42172=CARTESIAN_POINT('Ctrl Pts',(47.0872631521327,-50.1208169940441,-4.62896209536294));
#42173=CARTESIAN_POINT('Ctrl Pts',(43.1688982433533,-49.1856140242049,-4.82482465316824));
#42174=CARTESIAN_POINT('Ctrl Pts',(41.7800141094294,-45.4041871782722,-5.02068721097353));
#42175=CARTESIAN_POINT('Ctrl Pts',(44.161525406941,-42.1550962244138,-5.21654976877882));
#42176=CARTESIAN_POINT('Ctrl Pts',(48.1856432186892,-42.3412792339273,-5.41241232658412));
#42177=CARTESIAN_POINT('Ctrl Pts',(50.2569726507896,-45.79638884303,-5.60827488438941));
#42178=CARTESIAN_POINT('Ctrl Pts',(48.524860477633,-49.4334171929985,-5.80413744219471));
#42179=CARTESIAN_POINT('Ctrl Pts',(44.5368821864965,-50.0028190744713,-6.));
#42180=CARTESIAN_POINT('Ctrl Pts',(41.8561438759571,-46.9958556722001,-6.19586255780529));
#42181=CARTESIAN_POINT('Ctrl Pts',(42.8777812370783,-43.0991335633823,-6.39172511561059));
#42182=CARTESIAN_POINT('Ctrl Pts',(46.6890027641187,-41.7942240464804,-6.58758767341588));
#42183=CARTESIAN_POINT('Ctrl Pts',(49.8846236497149,-44.2470144323708,-6.78345023122117));
#42184=CARTESIAN_POINT('Ctrl Pts',(49.6094887496482,-48.2660291375546,-6.97931278902647));
#42185=CARTESIAN_POINT('Ctrl Pts',(46.1094011663011,-50.2604358378984,-7.17517534683175));
#42186=CARTESIAN_POINT('Ctrl Pts',(42.5115944258992,-48.4483023990436,-7.37103790463706));
#42187=CARTESIAN_POINT('Ctrl Pts',(42.0304898503225,-44.4487133548336,-7.56690046244234));
#42188=CARTESIAN_POINT('Ctrl Pts',(45.096101320591,-41.8351217569944,-7.76276302024765));
#42189=CARTESIAN_POINT('Ctrl Pts',(48.9690845637251,-42.9427250810239,-7.95862557805293));
#42190=CARTESIAN_POINT('Ctrl Pts',(50.1897686779422,-46.7818125353263,-8.15448813585822));
#42191=CARTESIAN_POINT('Ctrl Pts',(47.6661068961795,-49.922531125066,-8.35035069366353));
#42192=CARTESIAN_POINT('Ctrl Pts',(43.655781278647,-49.5583106984592,-8.54621325146881));
#42193=CARTESIAN_POINT('Ctrl Pts',(41.7359516028417,-46.0155174053566,-8.74207580927411));
#42194=CARTESIAN_POINT('Ctrl Pts',(43.6340789663225,-42.4575576103061,-8.9379383670794));
#42195=CARTESIAN_POINT('Ctrl Pts',(46.2953877954988,-42.1999380114139,-9.06851340561627));
#42196=CARTESIAN_POINT('Ctrl Pts',(47.3924914996766,-42.6569131519913,-9.1338009248847));
#42197=CARTESIAN_POINT('Ctrl Pts',(45.1221465072772,-49.27410725356,0.401402774654088));
#42198=CARTESIAN_POINT('Ctrl Pts',(44.0476798963079,-48.9860213131169,0.336115255385657));
#42199=CARTESIAN_POINT('Ctrl Pts',(42.2218744250559,-47.2743900252584,0.205540216848794));
#42200=CARTESIAN_POINT('Ctrl Pts',(42.8476421039081,-43.5520686795379,0.00967765904350066));
#42201=CARTESIAN_POINT('Ctrl Pts',(46.2952508119767,-42.0225271376179,-0.186184898761793));
#42202=CARTESIAN_POINT('Ctrl Pts',(49.4764847786399,-44.0439591775136,-0.382047456567085));
#42203=CARTESIAN_POINT('Ctrl Pts',(49.5528743447013,-47.814374730595,-0.57791001437238));
#42204=CARTESIAN_POINT('Ctrl Pts',(46.4542900095154,-49.9630625292705,-0.773772572177672));
#42205=CARTESIAN_POINT('Ctrl Pts',(42.9501168673143,-48.5712257881308,-0.969635129982967));
#42206=CARTESIAN_POINT('Ctrl Pts',(42.1707495593773,-44.8819410471107,-1.16549768778826));
#42207=CARTESIAN_POINT('Ctrl Pts',(44.812742827128,-42.1916756097399,-1.36136024559355));
#42208=CARTESIAN_POINT('Ctrl Pts',(48.5154694596864,-42.9039644153723,-1.55722280339885));
#42209=CARTESIAN_POINT('Ctrl Pts',(49.9707379648667,-46.3824605197014,-1.75308536120414));
#42210=CARTESIAN_POINT('Ctrl Pts',(47.8782960212063,-49.5192338636343,-1.94894791900943));
#42211=CARTESIAN_POINT('Ctrl Pts',(44.1076728071747,-49.5117111945868,-2.14481047681473));
#42212=CARTESIAN_POINT('Ctrl Pts',(42.027769291714,-46.3666071972827,-2.34067303462002));
#42213=CARTESIAN_POINT('Ctrl Pts',(43.4969024619949,-42.8939547884017,-2.53653559242531));
#42214=CARTESIAN_POINT('Ctrl Pts',(47.2024567355219,-42.1964340609653,-2.73239815023061));
#42215=CARTESIAN_POINT('Ctrl Pts',(49.833662300118,-44.8972537809427,-2.9282607080359));
#42216=CARTESIAN_POINT('Ctrl Pts',(49.0396376088954,-48.5833348043262,-3.12412326584119));
#42217=CARTESIAN_POINT('Ctrl Pts',(45.5298134238792,-49.9613053814918,-3.31998582364649));
#42218=CARTESIAN_POINT('Ctrl Pts',(42.440082872338,-47.8000015948883,-3.51584838145178));
#42219=CARTESIAN_POINT('Ctrl Pts',(42.5310016681808,-44.0304654767592,-3.71171093925708));
#42220=CARTESIAN_POINT('Ctrl Pts',(45.7213373360928,-42.0206328627957,-3.90757349706236));
#42221=CARTESIAN_POINT('Ctrl Pts',(49.1606474034209,-43.5662120721474,-4.10343605486766));
#42222=CARTESIAN_POINT('Ctrl Pts',(49.7760403106183,-47.2862873913398,-4.29929861267295));
#42223=CARTESIAN_POINT('Ctrl Pts',(47.0176861162341,-49.8571142911945,-4.49516117047825));
#42224=CARTESIAN_POINT('Ctrl Pts',(43.3500684303209,-48.9817575972797,-4.69102372828354));
#42225=CARTESIAN_POINT('Ctrl Pts',(42.0500629096888,-45.4423149213166,-4.88688628608883));
#42226=CARTESIAN_POINT('Ctrl Pts',(44.2791745818524,-42.4011424621584,-5.08274884389413));
#42227=CARTESIAN_POINT('Ctrl Pts',(48.0457777441811,-42.5754110957352,-5.27861140169942));
#42228=CARTESIAN_POINT('Ctrl Pts',(49.9845569634168,-45.8094184952813,-5.47447395950472));
#42229=CARTESIAN_POINT('Ctrl Pts',(48.3632875339104,-49.2137031423351,-5.67033651731001));
#42230=CARTESIAN_POINT('Ctrl Pts',(44.6305112223323,-49.7466673913265,-5.86619907511531));
#42231=CARTESIAN_POINT('Ctrl Pts',(42.1213209177207,-46.9321280587713,-6.06206163292059));
#42232=CARTESIAN_POINT('Ctrl Pts',(43.0775808224178,-43.2847681890032,-6.25792419072589));
#42233=CARTESIAN_POINT('Ctrl Pts',(46.6449115338041,-42.0633635127868,-6.45378674853118));
#42234=CARTESIAN_POINT('Ctrl Pts',(49.6360356251888,-44.3591929234098,-6.64964930633648));
#42235=CARTESIAN_POINT('Ctrl Pts',(49.3785073834378,-48.1210195413575,-6.84551186414177));
#42236=CARTESIAN_POINT('Ctrl Pts',(46.1024002770866,-49.9877985314141,-7.04137442194706));
#42237=CARTESIAN_POINT('Ctrl Pts',(42.7348273381726,-48.2916286227139,-7.23723697975236));
#42238=CARTESIAN_POINT('Ctrl Pts',(42.2845100014167,-44.5479845629013,-7.43309953755765));
#42239=CARTESIAN_POINT('Ctrl Pts',(45.1539443466722,-42.1016440634466,-7.62896209536294));
#42240=CARTESIAN_POINT('Ctrl Pts',(48.7790844677308,-43.1383687266052,-7.82482465316824));
#42241=CARTESIAN_POINT('Ctrl Pts',(49.9216535623511,-46.7317821459677,-8.02068721097353));
#42242=CARTESIAN_POINT('Ctrl Pts',(47.5594880163812,-49.6715172942683,-8.21654976877883));
#42243=CARTESIAN_POINT('Ctrl Pts',(43.8057944468573,-49.3306043600999,-8.41241232658412));
#42244=CARTESIAN_POINT('Ctrl Pts',(42.0088200871828,-46.0145244028186,-8.60827488438941));
#42245=CARTESIAN_POINT('Ctrl Pts',(43.7854809267131,-42.6842484908284,-8.80413744219471));
#42246=CARTESIAN_POINT('Ctrl Pts',(46.2764850972779,-42.4431146967252,-8.93471248073157));
#42247=CARTESIAN_POINT('Ctrl Pts',(47.3033820408749,-42.8708467090881,-9.));
#42248=CARTESIAN_POINT('Ctrl Pts',(42.6118898788522,-45.9972329038001,-1.10898219675043));
#42249=CARTESIAN_POINT('Ctrl Pts',(42.6093014257603,-45.675906530902,-1.12782069376304));
#42250=CARTESIAN_POINT('Ctrl Pts',(42.6514005654697,-45.35524393637,-1.14665919077564));
#42251=CARTESIAN_POINT('Ctrl Pts',(42.7409763219919,-45.0484442643856,-1.16549768778825));
#42252=CARTESIAN_POINT('Ctrl Pts',(43.0514139819609,-43.9851859013204,-1.23078520705669));
#42253=CARTESIAN_POINT('Ctrl Pts',(43.9320784045444,-43.0884307555301,-1.29607272632512));
#42254=CARTESIAN_POINT('Ctrl Pts',(44.9895317212626,-42.7587679835737,-1.36136024559355));
#42255=CARTESIAN_POINT('Ctrl Pts',(46.0469850379808,-42.4291052116173,-1.42664776486198));
#42256=CARTESIAN_POINT('Ctrl Pts',(47.2812272488336,-42.6665348134948,-1.49193528413041));
#42257=CARTESIAN_POINT('Ctrl Pts',(48.1408931051234,-43.3649989651551,-1.55722280339884));
#42258=CARTESIAN_POINT('Ctrl Pts',(49.0005589614132,-44.0634631168153,-1.62251032266727));
#42259=CARTESIAN_POINT('Ctrl Pts',(49.4856484631399,-45.2229618182583,-1.68779784193571));
#42260=CARTESIAN_POINT('Ctrl Pts',(49.3794528900599,-46.325506726302,-1.75308536120414));
#42261=CARTESIAN_POINT('Ctrl Pts',(49.2732573169799,-47.4280516343457,-1.81837288047257));
#42262=CARTESIAN_POINT('Ctrl Pts',(48.5757766690931,-48.47364274899,-1.883660399741));
#42263=CARTESIAN_POINT('Ctrl Pts',(47.5985991428111,-48.9951845281376,-1.94894791900943));
#42264=CARTESIAN_POINT('Ctrl Pts',(46.6214216165291,-49.5167263072851,-2.01423543827786));
#42265=CARTESIAN_POINT('Ctrl Pts',(45.3645472118519,-49.514218750936,-2.0795229575463));
#42266=CARTESIAN_POINT('Ctrl Pts',(44.3894594236032,-48.9887809732107,-2.14481047681473));
#42267=CARTESIAN_POINT('Ctrl Pts',(43.4143716353545,-48.4633431954854,-2.21009799608316));
#42268=CARTESIAN_POINT('Ctrl Pts',(42.7210704635343,-47.4149751963841,-2.27538551535159));
#42269=CARTESIAN_POINT('Ctrl Pts',(42.6192754060043,-46.3120157953532,-2.34067303462002));
#42270=CARTESIAN_POINT('Ctrl Pts',(42.6097596402894,-46.2089115434583,-2.34677608866349));
#42271=CARTESIAN_POINT('Ctrl Pts',(42.6054127175106,-46.1053302476658,-2.35287914270696));
#42272=CARTESIAN_POINT('Ctrl Pts',(42.6060559323604,-46.0016943206056,-2.35898219675043));
#42273=CARTESIAN_POINT('Ctrl Pts',(44.942095577027,-49.9456385074984,5.55111512312578E-16));
#42274=CARTESIAN_POINT('Ctrl Pts',(44.82663061034,-49.9039985139974,5.42846940041275E-16));
#42275=CARTESIAN_POINT('Ctrl Pts',(44.7135212423861,-49.8568503832162,-2.95193080891787E-17));
#42276=CARTESIAN_POINT('Ctrl Pts',(44.6029921165273,-49.8045482654284,1.38777878078145E-16));
#42277=CARTESIAN_POINT('Ctrl Pts',(44.4901063321701,-49.7511309824801,3.10663430578551E-16));
#42278=CARTESIAN_POINT('Ctrl Pts',(44.3799113698433,-49.6923370368737,-1.16889976070159E-16));
#42279=CARTESIAN_POINT('Ctrl Pts',(44.2726738374971,-49.6284969638907,-6.93889390390723E-18));
#42280=CARTESIAN_POINT('Ctrl Pts',(44.160705472714,-49.5618405570977,1.07862730181961E-16));
#42281=CARTESIAN_POINT('Ctrl Pts',(44.0519603129653,-49.4896824522167,5.85955431398957E-16));
#42282=CARTESIAN_POINT('Ctrl Pts',(43.9467834035794,-49.412356585367,5.48172618408671E-16));
#42283=CARTESIAN_POINT('Ctrl Pts',(43.8547536078667,-49.3446964518735,5.15112657042171E-16));
#42284=CARTESIAN_POINT('Ctrl Pts',(43.7654561119054,-49.2730787482686,1.19154455589423E-15));
#42285=CARTESIAN_POINT('Ctrl Pts',(43.679154686656,-49.1977078017425,1.36002320516582E-15));
#42286=CARTESIAN_POINT('Ctrl Pts',(43.6621944745782,-49.1828956797654,1.39313312906316E-15));
#42287=CARTESIAN_POINT('Ctrl Pts',(43.6453500786238,-49.1679385594659,5.1622689728816E-16));
#42288=CARTESIAN_POINT('Ctrl Pts',(43.6286236576442,-49.152837933438,5.13478148889135E-16));
#42289=CARTESIAN_POINT('Ctrl Pts',(43.6160017913096,-49.1414429025748,5.11403925424206E-16));
#42290=CARTESIAN_POINT('Ctrl Pts',(43.6034471475502,-49.1299661133717,1.00052068254941E-15));
#42291=CARTESIAN_POINT('Ctrl Pts',(43.5909710847022,-49.1184180804733,9.99200722162641E-16));
#42292=CARTESIAN_POINT('Ctrl Pts',(43.5004959172789,-49.034672893981,9.89628500666128E-16));
#42293=CARTESIAN_POINT('Ctrl Pts',(43.4140089081737,-48.9470574449428,1.70135956276898E-16));
#42294=CARTESIAN_POINT('Ctrl Pts',(43.3317676836786,-48.8558861730966,3.19189119579733E-16));
#42295=CARTESIAN_POINT('Ctrl Pts',(43.249852288359,-48.7650761101272,4.67651753381386E-16));
#42296=CARTESIAN_POINT('Ctrl Pts',(43.1721486259969,-48.6707376107984,1.09689163767266E-15));
#42297=CARTESIAN_POINT('Ctrl Pts',(43.0989537517469,-48.5731525014645,1.346145417358E-15));
#42298=CARTESIAN_POINT('Ctrl Pts',(43.0268380871154,-48.4770062195034,1.59172411625057E-15));
#42299=CARTESIAN_POINT('Ctrl Pts',(42.9590988800379,-48.3777076637844,9.41922024275774E-16));
#42300=CARTESIAN_POINT('Ctrl Pts',(42.8960675550739,-48.2755089103244,9.71445146547012E-16));
#42301=CARTESIAN_POINT('Ctrl Pts',(42.8445085118557,-48.1919112713806,9.95594788617647E-16));
#42302=CARTESIAN_POINT('Ctrl Pts',(42.7961003109415,-48.1063726153879,5.70479466357528E-16));
#42303=CARTESIAN_POINT('Ctrl Pts',(42.7510509740316,-48.0190267661575,5.55111512312578E-16));
#42304=CARTESIAN_POINT('Ctrl Pts',(42.7404166838962,-47.9984080142168,5.51483772298812E-16));
#42305=CARTESIAN_POINT('Ctrl Pts',(42.7299696743251,-47.9776885519846,5.63921738060297E-16));
#42306=CARTESIAN_POINT('Ctrl Pts',(42.7197128936464,-47.9568701328682,5.55111512312578E-16));
#42307=CARTESIAN_POINT('Ctrl Pts',(42.7124710693496,-47.9421712387317,5.48891031551775E-16));
#42308=CARTESIAN_POINT('Ctrl Pts',(42.705324800963,-47.9274243606889,3.80345069376565E-16));
#42309=CARTESIAN_POINT('Ctrl Pts',(42.6982802017053,-47.9126412259157,3.88578058618805E-16));
#42310=CARTESIAN_POINT('Ctrl Pts',(42.6476410529925,-47.8063746615825,4.47759787959845E-16));
#42311=CARTESIAN_POINT('Ctrl Pts',(42.6021744956729,-47.6980810220835,2.79773749468683E-16));
#42312=CARTESIAN_POINT('Ctrl Pts',(42.5621516727626,-47.5880163403607,1.94289029309402E-16));
#42313=CARTESIAN_POINT('Ctrl Pts',(42.5229349918356,-47.4801685877389,1.10526147262437E-16));
#42314=CARTESIAN_POINT('Ctrl Pts',(42.4889447313643,-47.3706197849924,1.994436682046E-16));
#42315=CARTESIAN_POINT('Ctrl Pts',(42.4604848736845,-47.2596000187875,1.94289029309402E-16));
#42316=CARTESIAN_POINT('Ctrl Pts',(42.4550245237132,-47.2382996038655,1.93300052742487E-16));
#42317=CARTESIAN_POINT('Ctrl Pts',(42.4497679053429,-47.2169450250228,4.20536784643823E-16));
#42318=CARTESIAN_POINT('Ctrl Pts',(42.4447173875259,-47.1955378899826,4.16333634234434E-16));
#42319=CARTESIAN_POINT('Ctrl Pts',(42.4175094478094,-47.080214261639,3.67266964756074E-16));
#42320=CARTESIAN_POINT('Ctrl Pts',(42.3962787129898,-46.9633646502898,-2.91090424899702E-16));
#42321=CARTESIAN_POINT('Ctrl Pts',(42.380940596355,-46.845425615413,-2.4980018054066E-16));
#42322=CARTESIAN_POINT('Ctrl Pts',(42.3724302191523,-46.7799869636134,-2.26890226036143E-16));
#42323=CARTESIAN_POINT('Ctrl Pts',(42.3657348704511,-46.7142130564285,9.61593993794892E-16));
#42324=CARTESIAN_POINT('Ctrl Pts',(42.3608466945119,-46.6481804853459,1.0547118733939E-15));
#42325=CARTESIAN_POINT('Ctrl Pts',(42.3589204350846,-46.6221593551456,1.09140637777708E-15));
#42326=CARTESIAN_POINT('Ctrl Pts',(42.3572748561029,-46.5960980794369,9.6891319473525E-16));
#42327=CARTESIAN_POINT('Ctrl Pts',(42.3559096667242,-46.5700014398623,9.99200722162641E-16));
#42328=CARTESIAN_POINT('Ctrl Pts',(42.355035272559,-46.5532867263352,1.01859966979129E-15));
#42329=CARTESIAN_POINT('Ctrl Pts',(42.3542759514787,-46.5365570378457,1.12141472518015E-16));
#42330=CARTESIAN_POINT('Ctrl Pts',(42.3536320498877,-46.5198290668053,1.11022302462516E-16));
#42331=CARTESIAN_POINT('Ctrl Pts',(42.3490547833004,-46.4009158912789,1.03066521995632E-16));
#42332=CARTESIAN_POINT('Ctrl Pts',(42.350294234656,-46.2819004401008,3.95995902974907E-17));
#42333=CARTESIAN_POINT('Ctrl Pts',(42.3571972740339,-46.163217984259,5.55111512312578E-17));
#42334=CARTESIAN_POINT('Ctrl Pts',(42.3639584195197,-46.0469750792689,7.10956456095611E-17));
#42335=CARTESIAN_POINT('Ctrl Pts',(42.3761532498072,-45.9310507101419,5.29470641973068E-16));
#42336=CARTESIAN_POINT('Ctrl Pts',(42.3936902278642,-45.815863702484,4.9960036108132E-16));
#42337=CARTESIAN_POINT('Ctrl Pts',(42.4110239463115,-45.7020117518776,4.70076287022706E-16));
#42338=CARTESIAN_POINT('Ctrl Pts',(42.4335770963145,-45.5888793559188,1.28993477976455E-16));
#42339=CARTESIAN_POINT('Ctrl Pts',(42.4613061905346,-45.4768933497828,1.11022302462516E-16));
#42340=CARTESIAN_POINT('Ctrl Pts',(42.4793959127936,-45.4038366631192,9.92983863787067E-17));
#42341=CARTESIAN_POINT('Ctrl Pts',(42.4996893681797,-45.331268353669,-2.62013610217355E-17));
#42342=CARTESIAN_POINT('Ctrl Pts',(42.522183785235,-45.2593146281972,-5.55111512312578E-17));
#42343=CARTESIAN_POINT('Ctrl Pts',(42.5314102394662,-45.2298016271181,-6.75330425844794E-17));
#42344=CARTESIAN_POINT('Ctrl Pts',(42.5410070574239,-45.2003921034647,5.52363651431842E-16));
#42345=CARTESIAN_POINT('Ctrl Pts',(42.5509743800709,-45.1710951322748,5.55111512312578E-16));
#42346=CARTESIAN_POINT('Ctrl Pts',(42.5570610432268,-45.1532045912102,5.56789525975078E-16));
#42347=CARTESIAN_POINT('Ctrl Pts',(42.5632831769561,-45.1353640243178,1.12910067832828E-16));
#42348=CARTESIAN_POINT('Ctrl Pts',(42.5696389447263,-45.1175795122746,1.11022302462516E-16));
#42349=CARTESIAN_POINT('Ctrl Pts',(42.6078193744145,-45.0107442193322,9.96821000518763E-17));
#42350=CARTESIAN_POINT('Ctrl Pts',(42.6508354931777,-44.9058800578143,1.89284020183184E-16));
#42351=CARTESIAN_POINT('Ctrl Pts',(42.6986279931034,-44.8033979085955,2.22044604925031E-16));
#42352=CARTESIAN_POINT('Ctrl Pts',(42.7370196795508,-44.7210740597619,2.48361162945569E-16));
#42353=CARTESIAN_POINT('Ctrl Pts',(42.7784944303779,-44.6402876042849,-1.09142067611465E-17));
#42354=CARTESIAN_POINT('Ctrl Pts',(42.8230401863722,-44.5612683184574,2.77555756156289E-16));
#42355=CARTESIAN_POINT('Ctrl Pts',(42.8451166911604,-44.5221070200802,4.2051906153628E-16));
#42356=CARTESIAN_POINT('Ctrl Pts',(42.8679477140259,-44.4833800189724,1.95633996835777E-17));
#42357=CARTESIAN_POINT('Ctrl Pts',(42.8915331690334,-44.4451169825572,0.));
#42358=CARTESIAN_POINT('Ctrl Pts',(42.9049285238735,-44.4233854980522,-1.11110292574829E-17));
#42359=CARTESIAN_POINT('Ctrl Pts',(42.9185690339628,-44.4018011557844,2.38874525753449E-17));
#42360=CARTESIAN_POINT('Ctrl Pts',(42.9324410403483,-44.3803901775881,5.55111512312578E-17));
#42361=CARTESIAN_POINT('Ctrl Pts',(42.9909913459386,-44.2900197379023,1.88986956298474E-16));
#42362=CARTESIAN_POINT('Ctrl Pts',(43.0537086663914,-44.2026583110029,-7.69983934686249E-16));
#42363=CARTESIAN_POINT('Ctrl Pts',(43.120561083899,-44.1186870123308,-1.11022302462516E-16));
#42364=CARTESIAN_POINT('Ctrl Pts',(43.1787980554028,-44.0455373146802,4.63017219645686E-16));
#42365=CARTESIAN_POINT('Ctrl Pts',(43.2401736532957,-43.9749604886065,-2.51258776215073E-17));
#42366=CARTESIAN_POINT('Ctrl Pts',(43.304686291877,-43.9072342474385,-1.11022302462516E-16));
#42367=CARTESIAN_POINT('Ctrl Pts',(43.3427056719154,-43.8673209876779,-2.14685645937026E-16));
#42368=CARTESIAN_POINT('Ctrl Pts',(43.3818149876739,-43.8283983093625,3.12743896641743E-16));
#42369=CARTESIAN_POINT('Ctrl Pts',(43.4219651657257,-43.7904875258606,2.77555756156289E-16));
#42370=CARTESIAN_POINT('Origin',(46.,-46.,-5.));
#42371=CARTESIAN_POINT('Origin',(-46.,-46.,-9.));
#42372=CARTESIAN_POINT('Ctrl Pts',(-44.696617959125,-42.8708467090881,-9.));
#42373=CARTESIAN_POINT('Ctrl Pts',(-44.7904997272541,-42.8200479292046,
-9.));
#42374=CARTESIAN_POINT('Ctrl Pts',(-44.886738796863,-42.7741603751026,-9.));
#42375=CARTESIAN_POINT('Ctrl Pts',(-44.9849439731347,-42.733071165152,-9.));
#42376=CARTESIAN_POINT('Ctrl Pts',(-45.0854084189225,-42.6910366730583,
-9.));
#42377=CARTESIAN_POINT('Ctrl Pts',(-45.1879310497138,-42.6540235798679,
-9.));
#42378=CARTESIAN_POINT('Ctrl Pts',(-45.2921276331192,-42.6219533204472,
-9.));
#42379=CARTESIAN_POINT('Ctrl Pts',(-45.3228379835846,-42.6125011016303,
-9.));
#42380=CARTESIAN_POINT('Ctrl Pts',(-45.3536939396971,-42.6034785481757,
-9.));
#42381=CARTESIAN_POINT('Ctrl Pts',(-45.3846861010656,-42.5948843786566,
-9.));
#42382=CARTESIAN_POINT('Ctrl Pts',(-45.4054440163549,-42.5891281798314,
-9.));
#42383=CARTESIAN_POINT('Ctrl Pts',(-45.4262630376611,-42.5835641629292,
-9.));
#42384=CARTESIAN_POINT('Ctrl Pts',(-45.4471403803258,-42.5781920278371,
-9.));
#42385=CARTESIAN_POINT('Ctrl Pts',(-45.4677328861357,-42.5728931866545,
-9.));
#42386=CARTESIAN_POINT('Ctrl Pts',(-45.4883746116549,-42.567782998565,-9.));
#42387=CARTESIAN_POINT('Ctrl Pts',(-45.5090571442629,-42.5628620679155,
-9.));
#42388=CARTESIAN_POINT('Ctrl Pts',(-45.6183973166331,-42.5368471008109,
-9.));
#42389=CARTESIAN_POINT('Ctrl Pts',(-45.7289240905594,-42.5161052932284,
-9.));
#42390=CARTESIAN_POINT('Ctrl Pts',(-45.8402228698817,-42.5005440545346,
-9.));
#42391=CARTESIAN_POINT('Ctrl Pts',(-45.9357752888625,-42.4871843931926,
-9.));
#42392=CARTESIAN_POINT('Ctrl Pts',(-46.0318975830046,-42.4776438143453,
-9.));
#42393=CARTESIAN_POINT('Ctrl Pts',(-46.128341200326,-42.4718911713871,-9.));
#42394=CARTESIAN_POINT('Ctrl Pts',(-46.1610020619997,-42.4699430250905,
-9.));
#42395=CARTESIAN_POINT('Ctrl Pts',(-46.1936998545402,-42.4684295178701,
-9.));
#42396=CARTESIAN_POINT('Ctrl Pts',(-46.2264251288074,-42.4673501149057,
-9.));
#42397=CARTESIAN_POINT('Ctrl Pts',(-46.2453983262225,-42.4667243073,-9.));
#42398=CARTESIAN_POINT('Ctrl Pts',(-46.2643828408655,-42.4662443894445,
-9.));
#42399=CARTESIAN_POINT('Ctrl Pts',(-46.2833702123848,-42.4659104209501,
-9.));
#42400=CARTESIAN_POINT('Ctrl Pts',(-46.3983318693734,-42.4638883626863,
-9.));
#42401=CARTESIAN_POINT('Ctrl Pts',(-46.5131366913024,-42.4672161609136,
-9.));
#42402=CARTESIAN_POINT('Ctrl Pts',(-46.6273657132139,-42.4757916011297,
-9.));
#42403=CARTESIAN_POINT('Ctrl Pts',(-46.7431939697372,-42.4844870996338,
-9.));
#42404=CARTESIAN_POINT('Ctrl Pts',(-46.8584310337364,-42.4985780118847,
-9.));
#42405=CARTESIAN_POINT('Ctrl Pts',(-46.9726595897454,-42.5180074306283,
-9.));
#42406=CARTESIAN_POINT('Ctrl Pts',(-47.0865463926996,-42.5373787197462,
-9.));
#42407=CARTESIAN_POINT('Ctrl Pts',(-47.1994316277292,-42.5620565574636,
-9.));
#42408=CARTESIAN_POINT('Ctrl Pts',(-47.3109076528104,-42.5920352736768,
-9.));
#42409=CARTESIAN_POINT('Ctrl Pts',(-47.3774374342275,-42.6099268107619,
-9.));
#42410=CARTESIAN_POINT('Ctrl Pts',(-47.4434653340186,-42.6297073870142,
-9.));
#42411=CARTESIAN_POINT('Ctrl Pts',(-47.5089036506937,-42.6513845973822,
-9.));
#42412=CARTESIAN_POINT('Ctrl Pts',(-47.5540019340407,-42.6663239330042,
-9.));
#42413=CARTESIAN_POINT('Ctrl Pts',(-47.5988201695549,-42.682164228417,-9.));
#42414=CARTESIAN_POINT('Ctrl Pts',(-47.6433291058402,-42.698909822974,-9.));
#42415=CARTESIAN_POINT('Ctrl Pts',(-47.6570944305462,-42.7040887503021,
-9.));
#42416=CARTESIAN_POINT('Ctrl Pts',(-47.6708276202054,-42.7093533588747,
-9.));
#42417=CARTESIAN_POINT('Ctrl Pts',(-47.684519940033,-42.7147005149645,-9.));
#42418=CARTESIAN_POINT('Ctrl Pts',(-47.7954788044728,-42.7580324247633,
-9.));
#42419=CARTESIAN_POINT('Ctrl Pts',(-47.9039046508829,-42.8068376390484,
-9.));
#42420=CARTESIAN_POINT('Ctrl Pts',(-48.0093701191363,-42.861056455776,-9.));
#42421=CARTESIAN_POINT('Ctrl Pts',(-48.0319897960043,-42.872685021361,-9.));
#42422=CARTESIAN_POINT('Ctrl Pts',(-48.0544733077876,-42.8845627997616,
-9.));
#42423=CARTESIAN_POINT('Ctrl Pts',(-48.0768164393444,-42.8966895147212,
-9.));
#42424=CARTESIAN_POINT('Ctrl Pts',(-48.1769659944078,-42.9510455974617,
-9.));
#42425=CARTESIAN_POINT('Ctrl Pts',(-48.2742962894481,-43.0103990269558,
-9.));
#42426=CARTESIAN_POINT('Ctrl Pts',(-48.3686669704147,-43.0743603461825,
-9.));
#42427=CARTESIAN_POINT('Ctrl Pts',(-48.4650739604994,-43.1397018082269,
-9.));
#42428=CARTESIAN_POINT('Ctrl Pts',(-48.5583927895653,-43.2098525452832,
-9.));
#42429=CARTESIAN_POINT('Ctrl Pts',(-48.6484540229757,-43.2844481095684,
-9.));
#42430=CARTESIAN_POINT('Ctrl Pts',(-48.6989515653842,-43.3262740154365,
-9.));
#42431=CARTESIAN_POINT('Ctrl Pts',(-48.7484245615551,-43.3694981915471,
-9.));
#42432=CARTESIAN_POINT('Ctrl Pts',(-48.7968394888843,-43.4140624125384,
-9.));
#42433=CARTESIAN_POINT('Ctrl Pts',(-48.8170272914924,-43.4326445678031,
-9.));
#42434=CARTESIAN_POINT('Ctrl Pts',(-48.8370310947172,-43.4514597614807,
-9.00000000000001));
#42435=CARTESIAN_POINT('Ctrl Pts',(-48.8568483097048,-43.4705039675987,
-9.00000000000001));
#42436=CARTESIAN_POINT('Ctrl Pts',(-48.8675797536332,-43.4808168107629,
-9.00000000000001));
#42437=CARTESIAN_POINT('Ctrl Pts',(-48.8782549321768,-43.4911953739355,
-9.));
#42438=CARTESIAN_POINT('Ctrl Pts',(-48.888867064305,-43.5016325280181,-9.));
#42439=CARTESIAN_POINT('Ctrl Pts',(-48.9743463294842,-43.5857023690979,
-9.));
#42440=CARTESIAN_POINT('Ctrl Pts',(-49.0558569064676,-43.6736845088744,
-9.));
#42441=CARTESIAN_POINT('Ctrl Pts',(-49.1332523820262,-43.7651463951702,
-9.));
#42442=CARTESIAN_POINT('Ctrl Pts',(-49.2120673577358,-43.8582857717904,
-9.));
#42443=CARTESIAN_POINT('Ctrl Pts',(-49.286615490809,-43.9550342143835,-9.));
#42444=CARTESIAN_POINT('Ctrl Pts',(-49.3567182741951,-44.0549849707905,
-9.));
#42445=CARTESIAN_POINT('Ctrl Pts',(-49.4273892475969,-44.1557458379964,
-9.));
#42446=CARTESIAN_POINT('Ctrl Pts',(-49.4935431267415,-44.2597617819432,
-9.));
#42447=CARTESIAN_POINT('Ctrl Pts',(-49.5549639159556,-44.3666576234218,
-9.));
#42448=CARTESIAN_POINT('Ctrl Pts',(-49.5912272721098,-44.4297698370639,
-9.));
#42449=CARTESIAN_POINT('Ctrl Pts',(-49.6258400878192,-44.4938866701378,
-9.));
#42450=CARTESIAN_POINT('Ctrl Pts',(-49.6587512269125,-44.5589362078444,
-9.));
#42451=CARTESIAN_POINT('Ctrl Pts',(-49.6760912942311,-44.5932092045848,
-9.));
#42452=CARTESIAN_POINT('Ctrl Pts',(-49.6929588912015,-44.6277411762725,
-9.));
#42453=CARTESIAN_POINT('Ctrl Pts',(-49.7093459082312,-44.6625219515001,
-9.));
#42454=CARTESIAN_POINT('Ctrl Pts',(-49.7168943224581,-44.6785431528006,
-9.));
#42455=CARTESIAN_POINT('Ctrl Pts',(-49.7243415069159,-44.6946187938948,
-9.));
#42456=CARTESIAN_POINT('Ctrl Pts',(-49.7316842773234,-44.7107427074915,
-9.));
#42457=CARTESIAN_POINT('Ctrl Pts',(-49.7841002776772,-44.8258424605655,
-9.));
#42458=CARTESIAN_POINT('Ctrl Pts',(-49.8310341812553,-44.9430352874127,
-9.));
#42459=CARTESIAN_POINT('Ctrl Pts',(-49.8723050335951,-45.0618934597966,
-9.));
#42460=CARTESIAN_POINT('Ctrl Pts',(-49.9136557204705,-45.1809815520019,
-9.));
#42461=CARTESIAN_POINT('Ctrl Pts',(-49.9493220045472,-45.3017421809313,
-9.));
#42462=CARTESIAN_POINT('Ctrl Pts',(-49.9790839449739,-45.4237811307975,
-9.));
#42463=CARTESIAN_POINT('Ctrl Pts',(-50.0083331061446,-45.5437174273752,
-9.));
#42464=CARTESIAN_POINT('Ctrl Pts',(-50.0318800488967,-45.664889160174,-9.));
#42465=CARTESIAN_POINT('Ctrl Pts',(-50.0494721954982,-45.78694540661,-9.));
#42466=CARTESIAN_POINT('Ctrl Pts',(-50.0603641529683,-45.862515004525,-9.));
#42467=CARTESIAN_POINT('Ctrl Pts',(-50.0689725651408,-45.9384240776739,
-9.));
#42468=CARTESIAN_POINT('Ctrl Pts',(-50.0752277437256,-46.0145919640507,
-9.));
#42469=CARTESIAN_POINT('Ctrl Pts',(-50.0806292004451,-46.080364273521,-9.));
#42470=CARTESIAN_POINT('Ctrl Pts',(-50.0842757987835,-46.1463296239162,
-9.));
#42471=CARTESIAN_POINT('Ctrl Pts',(-50.0861960634202,-46.2124371387131,
-9.));
#42472=CARTESIAN_POINT('Ctrl Pts',(-49.4256147683784,-48.2253962475631,
-9.));
#42473=CARTESIAN_POINT('Ctrl Pts',(-49.3489157903097,-48.32416642034,-9.));
#42474=CARTESIAN_POINT('Ctrl Pts',(-49.2674580358364,-48.4189429185709,
-9.));
#42475=CARTESIAN_POINT('Ctrl Pts',(-49.181649358739,-48.509586461748,-9.));
#42476=CARTESIAN_POINT('Ctrl Pts',(-49.0946357246301,-48.6015028549048,
-9.));
#42477=CARTESIAN_POINT('Ctrl Pts',(-49.0031473218947,-48.6891698089487,
-9.));
#42478=CARTESIAN_POINT('Ctrl Pts',(-48.9075793351274,-48.7723981712024,
-9.));
#42479=CARTESIAN_POINT('Ctrl Pts',(-48.8671612794576,-48.8075974957113,
-9.));
#42480=CARTESIAN_POINT('Ctrl Pts',(-48.8260132332562,-48.8420023423363,
-9.));
#42481=CARTESIAN_POINT('Ctrl Pts',(-48.7841640395052,-48.8755958163019,
-9.));
#42482=CARTESIAN_POINT('Ctrl Pts',(-48.7601546692882,-48.8948687838556,
-9.));
#42483=CARTESIAN_POINT('Ctrl Pts',(-48.7359100930681,-48.9138778990817,
-9.));
#42484=CARTESIAN_POINT('Ctrl Pts',(-48.7114611111693,-48.9326007103251,
-9.));
#42485=CARTESIAN_POINT('Ctrl Pts',(-48.6120344070545,-49.0087407893434,
-9.));
#42486=CARTESIAN_POINT('Ctrl Pts',(-48.5091640540545,-49.0802045044556,
-9.));
#42487=CARTESIAN_POINT('Ctrl Pts',(-48.4032434739676,-49.146819885912,-9.));
#42488=CARTESIAN_POINT('Ctrl Pts',(-48.315219738108,-49.2021796161617,-9.));
#42489=CARTESIAN_POINT('Ctrl Pts',(-48.2250887079674,-49.2541902643244,
-9.00000000000001));
#42490=CARTESIAN_POINT('Ctrl Pts',(-48.1330675829928,-49.3027271284968,
-9.00000000000001));
#42491=CARTESIAN_POINT('Ctrl Pts',(-48.0928083408164,-49.3239620065723,
-9.00000000000001));
#42492=CARTESIAN_POINT('Ctrl Pts',(-48.0521872566217,-49.3445316646075,
-9.00000000000001));
#42493=CARTESIAN_POINT('Ctrl Pts',(-48.0112223219151,-49.3644241467311,
-9.00000000000001));
#42494=CARTESIAN_POINT('Ctrl Pts',(-47.9888528780583,-49.3752866994295,
-9.00000000000001));
#42495=CARTESIAN_POINT('Ctrl Pts',(-47.966380902054,-49.3859473119928,-9.));
#42496=CARTESIAN_POINT('Ctrl Pts',(-47.9438093210079,-49.3964039173489,
-9.));
#42497=CARTESIAN_POINT('Ctrl Pts',(-47.9276093772253,-49.403908771288,-9.));
#42498=CARTESIAN_POINT('Ctrl Pts',(-47.9113666692195,-49.4113045751474,
-9.));
#42499=CARTESIAN_POINT('Ctrl Pts',(-47.8950830669899,-49.4185906009187,
-9.));
#42500=CARTESIAN_POINT('Ctrl Pts',(-47.7833615965889,-49.4685798785413,
-9.));
#42501=CARTESIAN_POINT('Ctrl Pts',(-47.6697055328393,-49.5134106633889,
-9.));
#42502=CARTESIAN_POINT('Ctrl Pts',(-47.5544816880324,-49.5529248054346,
-9.));
#42503=CARTESIAN_POINT('Ctrl Pts',(-47.440121123448,-49.5921428995799,-9.));
#42504=CARTESIAN_POINT('Ctrl Pts',(-47.3242153616244,-49.6261239014414,
-9.00000000000001));
#42505=CARTESIAN_POINT('Ctrl Pts',(-47.207114055994,-49.6546628848245,-9.00000000000001));
#42506=CARTESIAN_POINT('Ctrl Pts',(-47.093156836174,-49.6824356170355,-9.00000000000001));
#42507=CARTESIAN_POINT('Ctrl Pts',(-46.9780667128225,-49.7050546341585,
-9.));
#42508=CARTESIAN_POINT('Ctrl Pts',(-46.8621684928363,-49.7222822072425,
-9.));
#42509=CARTESIAN_POINT('Ctrl Pts',(-46.7940349211499,-49.7324098527391,
-9.));
#42510=CARTESIAN_POINT('Ctrl Pts',(-46.725622175006,-49.7406733115846,-9.));
#42511=CARTESIAN_POINT('Ctrl Pts',(-46.6569980993869,-49.7470160499487,
-9.));
#42512=CARTESIAN_POINT('Ctrl Pts',(-46.6091444604989,-49.751439032823,-9.));
#42513=CARTESIAN_POINT('Ctrl Pts',(-46.5611880896396,-49.754927900429,-9.00000000000001));
#42514=CARTESIAN_POINT('Ctrl Pts',(-46.5131526151167,-49.7574616543188,
-9.00000000000001));
#42515=CARTESIAN_POINT('Ctrl Pts',(-46.4976743750253,-49.7582780936572,
-9.00000000000001));
#42516=CARTESIAN_POINT('Ctrl Pts',(-46.4821913582372,-49.7589951350126,
-9.));
#42517=CARTESIAN_POINT('Ctrl Pts',(-46.4667128228249,-49.7596119474122,
-9.));
#42518=CARTESIAN_POINT('Ctrl Pts',(-46.3509652583505,-49.7642244337419,
-9.));
#42519=CARTESIAN_POINT('Ctrl Pts',(-46.2353273954703,-49.7632440066829,
-9.00000000000001));
#42520=CARTESIAN_POINT('Ctrl Pts',(-46.1201129558431,-49.7564872215625,
-9.00000000000001));
#42521=CARTESIAN_POINT('Ctrl Pts',(-46.0928431815546,-49.754887977529,-9.00000000000001));
#42522=CARTESIAN_POINT('Ctrl Pts',(-46.0655971479505,-49.7529649092835,
-9.));
#42523=CARTESIAN_POINT('Ctrl Pts',(-46.0383790696643,-49.7507151556099,
-9.));
#42524=CARTESIAN_POINT('Ctrl Pts',(-45.9217046490404,-49.7410712452773,
-9.));
#42525=CARTESIAN_POINT('Ctrl Pts',(-45.8055425487772,-49.7254282959812,
-9.));
#42526=CARTESIAN_POINT('Ctrl Pts',(-45.6902555581451,-49.7040295749359,
-9.));
#42527=CARTESIAN_POINT('Ctrl Pts',(-45.574018295102,-49.6824544713332,-9.));
#42528=CARTESIAN_POINT('Ctrl Pts',(-45.4586698083806,-49.6550277949428,
-9.));
#42529=CARTESIAN_POINT('Ctrl Pts',(-45.3446065975032,-49.6219525163758,
-9.));
#42530=CARTESIAN_POINT('Ctrl Pts',(-45.2880020256639,-49.6055387054077,
-9.));
#42531=CARTESIAN_POINT('Ctrl Pts',(-45.2317144362182,-49.587733147565,-9.));
#42532=CARTESIAN_POINT('Ctrl Pts',(-45.1757954701078,-49.5685570750744,
-9.));
#42533=CARTESIAN_POINT('Ctrl Pts',(-45.1531748577313,-49.5607998768841,
-9.));
#42534=CARTESIAN_POINT('Ctrl Pts',(-45.130614594322,-49.5528183825136,-9.00000000000001));
#42535=CARTESIAN_POINT('Ctrl Pts',(-45.1081182151183,-49.5446139009718,
-9.00000000000001));
#42536=CARTESIAN_POINT('Ctrl Pts',(-45.0928980597617,-49.5390630751009,
-9.00000000000001));
#42537=CARTESIAN_POINT('Ctrl Pts',(-45.0777075162266,-49.5334102502331,
-9.));
#42538=CARTESIAN_POINT('Ctrl Pts',(-45.0625604546644,-49.5276608672583,
-9.));
#42539=CARTESIAN_POINT('Ctrl Pts',(-44.9540999893991,-49.4864924366765,
-9.));
#42540=CARTESIAN_POINT('Ctrl Pts',(-44.847696747572,-49.4403157932029,-9.));
#42541=CARTESIAN_POINT('Ctrl Pts',(-44.7436925895056,-49.3893796291663,
-9.));
#42542=CARTESIAN_POINT('Ctrl Pts',(-44.6397899691822,-49.338493193364,-9.));
#42543=CARTESIAN_POINT('Ctrl Pts',(-44.538281011366,-49.2828559183071,-9.));
#42544=CARTESIAN_POINT('Ctrl Pts',(-44.4395357151276,-49.2226729043818,
-9.));
#42545=CARTESIAN_POINT('Ctrl Pts',(-44.3421823782594,-49.1633382580584,
-9.));
#42546=CARTESIAN_POINT('Ctrl Pts',(-44.2475147356571,-49.0995845005203,
-9.));
#42547=CARTESIAN_POINT('Ctrl Pts',(-44.1559255117573,-49.0315757708794,
-9.));
#42548=CARTESIAN_POINT('Ctrl Pts',(-44.1056634674231,-48.9942541555324,
-9.));
#42549=CARTESIAN_POINT('Ctrl Pts',(-44.0563292320097,-48.9556506133514,
-9.));
#42550=CARTESIAN_POINT('Ctrl Pts',(-44.0079936818957,-48.9157890410837,
-9.));
#42551=CARTESIAN_POINT('Ctrl Pts',(-43.9809707187663,-48.8935036259983,
-9.));
#42552=CARTESIAN_POINT('Ctrl Pts',(-43.9542599849663,-48.8708249647296,
-9.));
#42553=CARTESIAN_POINT('Ctrl Pts',(-43.9278745179484,-48.8477569807897,
-9.));
#42554=CARTESIAN_POINT('Ctrl Pts',(-43.9114578068069,-48.833404366576,-9.));
#42555=CARTESIAN_POINT('Ctrl Pts',(-43.8951635188026,-48.8188977346138,
-9.));
#42556=CARTESIAN_POINT('Ctrl Pts',(-43.8790167509615,-48.8042581930767,
-9.));
#42557=CARTESIAN_POINT('Ctrl Pts',(-43.7964009707645,-48.7293542149109,
-9.));
#42558=CARTESIAN_POINT('Ctrl Pts',(-43.7175410737808,-48.6508864608485,
-9.));
#42559=CARTESIAN_POINT('Ctrl Pts',(-43.6427713171281,-48.5690422853087,
-9.));
#42560=CARTESIAN_POINT('Ctrl Pts',(-43.5691131678398,-48.488414893029,-9.));
#42561=CARTESIAN_POINT('Ctrl Pts',(-43.4994239498864,-48.4045101397136,
-9.));
#42562=CARTESIAN_POINT('Ctrl Pts',(-43.4340655377993,-48.3174806252745,
-9.));
#42563=CARTESIAN_POINT('Ctrl Pts',(-43.3705929531023,-48.232962228178,-9.));
#42564=CARTESIAN_POINT('Ctrl Pts',(-43.3112045665986,-48.1454962597952,
-9.));
#42565=CARTESIAN_POINT('Ctrl Pts',(-43.256277583738,-48.0552054878722,-9.));
#42566=CARTESIAN_POINT('Ctrl Pts',(-43.2286235921166,-48.0097469514626,
-9.));
#42567=CARTESIAN_POINT('Ctrl Pts',(-43.2021012370726,-47.9635721597901,
-9.));
#42568=CARTESIAN_POINT('Ctrl Pts',(-43.1767635963711,-47.9166956970799,
-9.));
#42569=CARTESIAN_POINT('Ctrl Pts',(-43.1505634206932,-47.8682234824552,
-9.));
#42570=CARTESIAN_POINT('Ctrl Pts',(-43.1256300485181,-47.8190009337087,
-9.));
#42571=CARTESIAN_POINT('Ctrl Pts',(-43.1019720879322,-47.7690801693092,
-9.));
#42572=CARTESIAN_POINT('Origin',(-46.,-46.,2.76038497140452));
#42573=CARTESIAN_POINT('Ctrl Pts',(-50.0901578141997,-45.9981376217778,
-0.364615028595479));
#42574=CARTESIAN_POINT('Ctrl Pts',(-50.0908678443317,-45.8792552045722,
-0.370425837919348));
#42575=CARTESIAN_POINT('Ctrl Pts',(-50.0327404569368,-44.4253400287511,
-0.441524166511649));
#42576=CARTESIAN_POINT('Ctrl Pts',(-48.2991257101273,-41.7778216414365,
-0.577910014372381));
#42577=CARTESIAN_POINT('Ctrl Pts',(-43.7551462487284,-41.7491661756407,
-0.773772572177673));
#42578=CARTESIAN_POINT('Ctrl Pts',(-41.2169403724754,-45.5179447459126,
-0.969635129982968));
#42579=CARTESIAN_POINT('Ctrl Pts',(-42.9521741545416,-49.7176769546074,
-1.16549768778826));
#42580=CARTESIAN_POINT('Ctrl Pts',(-47.4105432027648,-50.5956823608512,
-1.36136024559355));
#42581=CARTESIAN_POINT('Ctrl Pts',(-49.8549768496287,-48.1283902680758,
-1.51106602586263));
#42582=CARTESIAN_POINT('Ctrl Pts',(-50.0859947420446,-46.3965852541406,
-1.59548428686327));
#42583=CARTESIAN_POINT('Ctrl Pts',(-50.0828677018166,-46.0033110698502,
-1.61461502859548));
#42584=CARTESIAN_POINT('Ctrl Pts',(-50.0805802565567,-46.0038346370175,
-0.260384971404518));
#42585=CARTESIAN_POINT('Ctrl Pts',(-50.0745370386142,-45.103146971309,-0.304165019473208));
#42586=CARTESIAN_POINT('Ctrl Pts',(-49.3426919586741,-42.8475836408644,
-0.413232586810328));
#42587=CARTESIAN_POINT('Ctrl Pts',(-45.6441921539078,-41.2067322013831,
-0.58758767341588));
#42588=CARTESIAN_POINT('Ctrl Pts',(-41.8104753331013,-43.6427683056469,
-0.783450231221174));
#42589=CARTESIAN_POINT('Ctrl Pts',(-41.7184180535194,-48.1865095079258,
-0.979312789026466));
#42590=CARTESIAN_POINT('Ctrl Pts',(-45.4525334082598,-50.7759013692154,
-1.17517534683176));
#42591=CARTESIAN_POINT('Ctrl Pts',(-49.2692582722498,-49.2599208265826,
-1.35219940762444));
#42592=CARTESIAN_POINT('Ctrl Pts',(-50.0753327932863,-46.9514405162048,
-1.4639359491487));
#42593=CARTESIAN_POINT('Ctrl Pts',(-50.0830240067876,-45.9966653604899,
-1.51038497140452));
#42594=CARTESIAN_POINT('Ctrl Pts',(-43.4267655729853,-43.7934484719077,
0.));
#42595=CARTESIAN_POINT('Ctrl Pts',(-42.7026396483563,-44.6379090408209,
-0.0652875192684312));
#42596=CARTESIAN_POINT('Ctrl Pts',(-42.1622118099361,-47.0815123730999,
-0.195862557805293));
#42597=CARTESIAN_POINT('Ctrl Pts',(-44.7804699456593,-49.8003252158879,
-0.391725115610587));
#42598=CARTESIAN_POINT('Ctrl Pts',(-48.4895469401944,-49.1160278933692,
-0.58758767341588));
#42599=CARTESIAN_POINT('Ctrl Pts',(-49.9737289311609,-45.6513995309775,
-0.783450231221174));
#42600=CARTESIAN_POINT('Ctrl Pts',(-47.9078240822286,-42.4964188271871,
-0.979312789026467));
#42601=CARTESIAN_POINT('Ctrl Pts',(-44.1372110150862,-42.4726404024181,
-1.17517534683176));
#42602=CARTESIAN_POINT('Ctrl Pts',(-42.0309972160583,-45.5999885440531,
-1.37103790463705));
#42603=CARTESIAN_POINT('Ctrl Pts',(-43.4709014297081,-49.0849438082939,
-1.56690046244235));
#42604=CARTESIAN_POINT('Ctrl Pts',(-47.1704746197239,-49.813516348273,-1.76276302024764));
#42605=CARTESIAN_POINT('Ctrl Pts',(-49.824265602867,-47.1349091719286,-1.95862557805294));
#42606=CARTESIAN_POINT('Ctrl Pts',(-49.0612259744186,-43.4422793602443,
-2.15448813585823));
#42607=CARTESIAN_POINT('Ctrl Pts',(-45.5630964920078,-42.0348869356059,
-2.35035069366352));
#42608=CARTESIAN_POINT('Ctrl Pts',(-42.4553244696169,-44.1701649184598,
-2.54621325146881));
#42609=CARTESIAN_POINT('Ctrl Pts',(-42.5145835375169,-47.9403332310127,
-2.74207580927411));
#42610=CARTESIAN_POINT('Ctrl Pts',(-45.6879286795441,-49.9768868435812,
-2.9379383670794));
#42611=CARTESIAN_POINT('Ctrl Pts',(-49.1400974595928,-48.4602453793828,
-3.13380092488469));
#42612=CARTESIAN_POINT('Ctrl Pts',(-49.7867097218029,-44.7454687457041,
-3.32966348268999));
#42613=CARTESIAN_POINT('Ctrl Pts',(-47.050042144684,-42.1515678088258,-3.52552604049528));
#42614=CARTESIAN_POINT('Ctrl Pts',(-43.3752022219567,-42.996093261025,-3.72138859830058));
#42615=CARTESIAN_POINT('Ctrl Pts',(-42.0455183750331,-46.5244941426766,
-3.91725115610587));
#42616=CARTESIAN_POINT('Ctrl Pts',(-44.2490121010238,-49.5842796169672,
-4.11311371391116));
#42617=CARTESIAN_POINT('Ctrl Pts',(-48.0169463150116,-49.4416488178989,
-4.30897627171646));
#42618=CARTESIAN_POINT('Ctrl Pts',(-49.9828164023805,-46.2240368762855,
-4.50483882952175));
#42619=CARTESIAN_POINT('Ctrl Pts',(-48.3901928829157,-42.8062565861503,
-4.70070138732704));
#42620=CARTESIAN_POINT('Ctrl Pts',(-44.6620237528019,-42.2419634675882,
-4.89656394513234));
#42621=CARTESIAN_POINT('Ctrl Pts',(-42.1292850495319,-45.0353317691525,
-5.09242650293763));
#42622=CARTESIAN_POINT('Ctrl Pts',(-43.0548816114063,-48.6905941113693,
-5.28828906074292));
#42623=CARTESIAN_POINT('Ctrl Pts',(-46.6118284191898,-49.9419138769607,
-5.48415161854822));
#42624=CARTESIAN_POINT('Ctrl Pts',(-49.6221300325651,-47.6712848647882,
-5.68001417635351));
#42625=CARTESIAN_POINT('Ctrl Pts',(-49.3961974327852,-43.9074269825829,
-5.87587673415881));
#42626=CARTESIAN_POINT('Ctrl Pts',(-46.1358928380674,-42.0132027488516,
-6.0717392919641));
#42627=CARTESIAN_POINT('Ctrl Pts',(-42.7541730553862,-43.6810289290001,
-6.26760184976939));
#42628=CARTESIAN_POINT('Ctrl Pts',(-42.2724753932177,-47.4207666175459,
-6.46346440757469));
#42629=CARTESIAN_POINT('Ctrl Pts',(-45.121177278434,-49.8911041605667,-6.65932696537998));
#42630=CARTESIAN_POINT('Ctrl Pts',(-48.7550748399576,-48.8848888483899,
-6.85518952318527));
#42631=CARTESIAN_POINT('Ctrl Pts',(-49.9274161038516,-45.3011373268432,
-7.05105208099057));
#42632=CARTESIAN_POINT('Ctrl Pts',(-47.5907672407131,-42.3417902023858,
-7.24691463879586));
#42633=CARTESIAN_POINT('Ctrl Pts',(-43.8328177801406,-42.6509184160841,
-7.44277719660115));
#42634=CARTESIAN_POINT('Ctrl Pts',(-42.0111851884223,-45.9523117110681,
-7.63863975440645));
#42635=CARTESIAN_POINT('Ctrl Pts',(-43.753359094242,-49.2963347098191,-7.83450231221174));
#42636=CARTESIAN_POINT('Ctrl Pts',(-47.5029153976546,-49.6951640790793,
-8.03036487001703));
#42637=CARTESIAN_POINT('Ctrl Pts',(-49.9094803345903,-46.7925982881772,
-8.22622742782233));
#42638=CARTESIAN_POINT('Ctrl Pts',(-48.8234714875911,-43.1816880013063,
-8.42208998562762));
#42639=CARTESIAN_POINT('Ctrl Pts',(-45.2139879040286,-42.0892163329667,
-8.61795254343291));
#42640=CARTESIAN_POINT('Ctrl Pts',(-42.3084348061939,-44.4900926453702,
-8.81381510123821));
#42641=CARTESIAN_POINT('Ctrl Pts',(-42.6977478369022,-48.2416190468656,
-9.0096776590435));
#42642=CARTESIAN_POINT('Ctrl Pts',(-46.0445080898354,-49.9870172102589,
-9.2055402168488));
#42643=CARTESIAN_POINT('Ctrl Pts',(-48.2365749371353,-48.7794980878294,
-9.33611525538566));
#42644=CARTESIAN_POINT('Ctrl Pts',(-48.8425893907247,-47.8466430673628,
-9.40140277465409));
#42645=CARTESIAN_POINT('Ctrl Pts',(-43.2508390065835,-43.6425912356409,
0.133800924884696));
#42646=CARTESIAN_POINT('Ctrl Pts',(-42.4772061321698,-44.5447857781054,
0.0685134056162645));
#42647=CARTESIAN_POINT('Ctrl Pts',(-41.8998303915285,-47.155453074469,-0.0620616329205977));
#42648=CARTESIAN_POINT('Ctrl Pts',(-44.6970932688856,-50.0601453704073,
-0.257924190725891));
#42649=CARTESIAN_POINT('Ctrl Pts',(-48.659751971064,-49.329064094944,-0.453786748531184));
#42650=CARTESIAN_POINT('Ctrl Pts',(-50.2454043289916,-45.6275664581267,
-0.649649306336479));
#42651=CARTESIAN_POINT('Ctrl Pts',(-48.0382579581949,-42.2568864319368,
-0.845511864141771));
#42652=CARTESIAN_POINT('Ctrl Pts',(-44.0098560929669,-42.2314823268256,
-1.04137442194707));
#42653=CARTESIAN_POINT('Ctrl Pts',(-41.759644934864,-45.5726406113396,-1.23723697975236));
#42654=CARTESIAN_POINT('Ctrl Pts',(-43.2979923379859,-49.2958548570651,
-1.43309953755765));
#42655=CARTESIAN_POINT('Ctrl Pts',(-47.2504974807376,-50.0742383524657,
-1.62896209536295));
#42656=CARTESIAN_POINT('Ctrl Pts',(-50.0857225107405,-47.212500498898,-1.82482465316824));
#42657=CARTESIAN_POINT('Ctrl Pts',(-49.2705154853181,-43.267413438491,-2.02068721097353));
#42658=CARTESIAN_POINT('Ctrl Pts',(-45.5332263281381,-41.7638005862665,
-2.21654976877883));
#42659=CARTESIAN_POINT('Ctrl Pts',(-42.2129825405171,-44.0450629846456,
-2.41241232658412));
#42660=CARTESIAN_POINT('Ctrl Pts',(-42.2762930248891,-48.0729896883583,
-2.60827488438941));
#42661=CARTESIAN_POINT('Ctrl Pts',(-45.6665930269102,-50.2487781411695,
-2.80413744219471));
#42662=CARTESIAN_POINT('Ctrl Pts',(-49.3547792462321,-48.6284471248425,
-3.));
#42663=CARTESIAN_POINT('Ctrl Pts',(-50.0455990139418,-44.6596991113113,
-3.19586255780529));
#42664=CARTESIAN_POINT('Ctrl Pts',(-47.1218312934503,-41.8884586826942,
-3.39172511561059));
#42665=CARTESIAN_POINT('Ctrl Pts',(-43.1957503788823,-42.790722544377,-3.58758767341588));
#42666=CARTESIAN_POINT('Ctrl Pts',(-41.775158874602,-46.5603526919989,-3.78345023122118));
#42667=CARTESIAN_POINT('Ctrl Pts',(-44.1293007814315,-49.8293291932581,
-3.97931278902646));
#42668=CARTESIAN_POINT('Ctrl Pts',(-48.1548406460106,-49.6769470297281,
-4.17517534683177));
#42669=CARTESIAN_POINT('Ctrl Pts',(-50.2551130912961,-46.2393538011558,
-4.37103790463705));
#42670=CARTESIAN_POINT('Ctrl Pts',(-48.5536052881419,-42.5879071396839,
-4.56690046244235));
#42671=CARTESIAN_POINT('Ctrl Pts',(-44.5705491616704,-41.9850345004413,
-4.76276302024764));
#42672=CARTESIAN_POINT('Ctrl Pts',(-41.8646524985264,-44.9693794533479,
-4.95862557805293));
#42673=CARTESIAN_POINT('Ctrl Pts',(-42.8535301292744,-48.8745443098529,
-5.15448813585823));
#42674=CARTESIAN_POINT('Ctrl Pts',(-46.6536578273016,-50.2114141471829,
-5.35035069366352));
#42675=CARTESIAN_POINT('Ctrl Pts',(-49.8697673612905,-47.7855470574026,
-5.54621325146882));
#42676=CARTESIAN_POINT('Ctrl Pts',(-49.6283882300557,-43.7643622147427,
-5.74207580927411));
#42677=CARTESIAN_POINT('Ctrl Pts',(-46.1451835424621,-41.7406338977701,
-5.9379383670794));
#42678=CARTESIAN_POINT('Ctrl Pts',(-42.5322627686646,-43.5224858076182,
-6.1338009248847));
#42679=CARTESIAN_POINT('Ctrl Pts',(-42.0176324615496,-47.5179014102639,
-6.32966348268999));
#42680=CARTESIAN_POINT('Ctrl Pts',(-45.0610940375688,-50.1571306785139,
-6.52552604049528));
#42681=CARTESIAN_POINT('Ctrl Pts',(-48.9434334487518,-49.0821225649218,
-6.72138859830058));
#42682=CARTESIAN_POINT('Ctrl Pts',(-50.1959251921524,-45.2533575718454,
-6.91725115610588));
#42683=CARTESIAN_POINT('Ctrl Pts',(-47.6995246145712,-42.0916861768389,
-7.11311371391116));
#42684=CARTESIAN_POINT('Ctrl Pts',(-43.6846521397682,-42.4219488292201,
-7.30897627171646));
#42685=CARTESIAN_POINT('Ctrl Pts',(-41.7384784010241,-45.9490513641516,
-7.50483882952175));
#42686=CARTESIAN_POINT('Ctrl Pts',(-43.5997610324648,-49.521698105055,-7.70070138732705));
#42687=CARTESIAN_POINT('Ctrl Pts',(-47.6056665277988,-49.9477945902752,
-7.89656394513234));
#42688=CARTESIAN_POINT('Ctrl Pts',(-50.1767631924828,-46.8467865478674,
-8.09242650293763));
#42689=CARTESIAN_POINT('Ctrl Pts',(-49.0165062297547,-42.9890060024281,
-8.28828906074293));
#42690=CARTESIAN_POINT('Ctrl Pts',(-45.1602499282955,-41.8218443690062,
-8.48415161854821));
#42691=CARTESIAN_POINT('Ctrl Pts',(-42.0560503431317,-44.3868634899944,
-8.68001417635352));
#42692=CARTESIAN_POINT('Ctrl Pts',(-42.4719798779679,-48.3948737748281,
-8.8758767341588));
#42693=CARTESIAN_POINT('Ctrl Pts',(-46.0475510133015,-50.2596010994772,
-9.0717392919641));
#42694=CARTESIAN_POINT('Ctrl Pts',(-48.3894848100407,-48.9695264621503,
-9.20231433050096));
#42695=CARTESIAN_POINT('Ctrl Pts',(-49.036931183276,-47.9728941274296,-9.2676018497694));
#42696=CARTESIAN_POINT('Ctrl Pts',(-43.0749124401816,-43.4917339993741,
0.267601849769391));
#42697=CARTESIAN_POINT('Ctrl Pts',(-42.2517726159832,-44.45166251539,0.20231433050096));
#42698=CARTESIAN_POINT('Ctrl Pts',(-41.6374489731208,-47.2293937758381,
0.0717392919640981));
#42699=CARTESIAN_POINT('Ctrl Pts',(-44.613716592112,-50.3199655249267,-0.124123265841196));
#42700=CARTESIAN_POINT('Ctrl Pts',(-48.8299570019335,-49.5421002965189,
-0.319985823646488));
#42701=CARTESIAN_POINT('Ctrl Pts',(-50.5170797268223,-45.603733385276,-0.515848381451784));
#42702=CARTESIAN_POINT('Ctrl Pts',(-48.1686918341611,-42.0173540366867,
-0.711710939257075));
#42703=CARTESIAN_POINT('Ctrl Pts',(-43.8825011708477,-41.9903242512331,
-0.907573497062371));
#42704=CARTESIAN_POINT('Ctrl Pts',(-41.4882926536697,-45.545292678626,-1.10343605486766));
#42705=CARTESIAN_POINT('Ctrl Pts',(-43.1250832462638,-49.5067659058363,
-1.29929861267296));
#42706=CARTESIAN_POINT('Ctrl Pts',(-47.3305203417512,-50.3349603566584,
-1.49516117047825));
#42707=CARTESIAN_POINT('Ctrl Pts',(-50.3471794186141,-47.2900918258674,
-1.69102372828354));
#42708=CARTESIAN_POINT('Ctrl Pts',(-49.4798049962175,-43.0925475167376,
-1.88688628608884));
#42709=CARTESIAN_POINT('Ctrl Pts',(-45.5033561642685,-41.4927142369271,
-2.08274884389413));
#42710=CARTESIAN_POINT('Ctrl Pts',(-41.9706406114172,-43.9199610508312,
-2.27861140169943));
#42711=CARTESIAN_POINT('Ctrl Pts',(-42.0380025122611,-48.2056461457039,
-2.47447395950472));
#42712=CARTESIAN_POINT('Ctrl Pts',(-45.6452573742764,-50.5206694387578,
-2.67033651731001));
#42713=CARTESIAN_POINT('Ctrl Pts',(-49.5694610328715,-48.7966488703022,
-2.8661990751153));
#42714=CARTESIAN_POINT('Ctrl Pts',(-50.3044883060807,-44.5739294769185,
-3.0620616329206));
#42715=CARTESIAN_POINT('Ctrl Pts',(-47.1936204422165,-41.6253495565626,
-3.25792419072589));
#42716=CARTESIAN_POINT('Ctrl Pts',(-43.0162985358079,-42.585351827729,-3.45378674853118));
#42717=CARTESIAN_POINT('Ctrl Pts',(-41.5047993741709,-46.5962112413212,
-3.64964930633648));
#42718=CARTESIAN_POINT('Ctrl Pts',(-44.0095894618394,-50.074378769549,-3.84551186414177));
#42719=CARTESIAN_POINT('Ctrl Pts',(-48.2927349770096,-49.9122452415573,
-4.04137442194707));
#42720=CARTESIAN_POINT('Ctrl Pts',(-50.5274097802118,-46.2546707260261,
-4.23723697975236));
#42721=CARTESIAN_POINT('Ctrl Pts',(-48.7170176933682,-42.3695576932174,
-4.43309953755765));
#42722=CARTESIAN_POINT('Ctrl Pts',(-44.4790745705388,-41.7281055332943,
-4.62896209536295));
#42723=CARTESIAN_POINT('Ctrl Pts',(-41.6000199475209,-44.9034271375432,
-4.82482465316824));
#42724=CARTESIAN_POINT('Ctrl Pts',(-42.6521786471426,-49.0584945083365,
-5.02068721097354));
#42725=CARTESIAN_POINT('Ctrl Pts',(-46.6954872354135,-50.480914417405,-5.21654976877883));
#42726=CARTESIAN_POINT('Ctrl Pts',(-50.1174046900159,-47.8998092500169,
-5.41241232658412));
#42727=CARTESIAN_POINT('Ctrl Pts',(-49.8605790273263,-43.6212974469025,
-5.60827488438941));
#42728=CARTESIAN_POINT('Ctrl Pts',(-46.1544742468569,-41.4680650466885,
-5.80413744219471));
#42729=CARTESIAN_POINT('Ctrl Pts',(-42.3103524819431,-43.3639426862363,
-6.));
#42730=CARTESIAN_POINT('Ctrl Pts',(-41.7627895298816,-47.6150362029821,
-6.1958625578053));
#42731=CARTESIAN_POINT('Ctrl Pts',(-45.0010107967036,-50.423157196461,-6.39172511561059));
#42732=CARTESIAN_POINT('Ctrl Pts',(-49.131792057546,-49.2793562814538,-6.58758767341588));
#42733=CARTESIAN_POINT('Ctrl Pts',(-50.4644342804531,-45.2055778168475,
-6.78345023122118));
#42734=CARTESIAN_POINT('Ctrl Pts',(-47.8082819884292,-41.8415821512922,
-6.97931278902647));
#42735=CARTESIAN_POINT('Ctrl Pts',(-43.5364864993957,-42.1929792423559,
-7.17517534683176));
#42736=CARTESIAN_POINT('Ctrl Pts',(-41.4657716136258,-45.9457910172352,
-7.37103790463706));
#42737=CARTESIAN_POINT('Ctrl Pts',(-43.4461629706875,-49.7470615002908,
-7.56690046244235));
#42738=CARTESIAN_POINT('Ctrl Pts',(-47.7084176579431,-50.2004251014713,
-7.76276302024765));
#42739=CARTESIAN_POINT('Ctrl Pts',(-50.4440460503753,-46.9009748075577,
-7.95862557805293));
#42740=CARTESIAN_POINT('Ctrl Pts',(-49.2095409719184,-42.79632400355,-8.15448813585823));
#42741=CARTESIAN_POINT('Ctrl Pts',(-45.1065119525624,-41.5544724050458,
-8.35035069366352));
#42742=CARTESIAN_POINT('Ctrl Pts',(-41.8036658800697,-44.2836343346184,
-8.54621325146882));
#42743=CARTESIAN_POINT('Ctrl Pts',(-42.2462119190335,-48.5481285027907,
-8.74207580927411));
#42744=CARTESIAN_POINT('Ctrl Pts',(-46.0505939367677,-50.5321849886954,
-8.93793836707941));
#42745=CARTESIAN_POINT('Ctrl Pts',(-48.5423946829461,-49.1595548364713,
-9.06851340561627));
#42746=CARTESIAN_POINT('Ctrl Pts',(-49.2312729758272,-48.0991451874963,
-9.1338009248847));
#42747=CARTESIAN_POINT('Ctrl Pts',(-42.8989858737798,-43.3408767631073,
0.401402774654087));
#42748=CARTESIAN_POINT('Ctrl Pts',(-42.0263390997967,-44.3585392526745,
0.336115255385656));
#42749=CARTESIAN_POINT('Ctrl Pts',(-41.3750675547132,-47.3033344772072,
0.205540216848794));
#42750=CARTESIAN_POINT('Ctrl Pts',(-44.5303399153384,-50.5797856794461,
0.00967765904350008));
#42751=CARTESIAN_POINT('Ctrl Pts',(-49.0001620328031,-49.7551364980937,
-0.186184898761793));
#42752=CARTESIAN_POINT('Ctrl Pts',(-50.7887551246529,-45.5799003124252,
-0.382047456567087));
#42753=CARTESIAN_POINT('Ctrl Pts',(-48.2991257101273,-41.7778216414365,
-0.577910014372381));
#42754=CARTESIAN_POINT('Ctrl Pts',(-43.7551462487284,-41.7491661756407,
-0.773772572177673));
#42755=CARTESIAN_POINT('Ctrl Pts',(-41.2169403724754,-45.5179447459126,
-0.969635129982968));
#42756=CARTESIAN_POINT('Ctrl Pts',(-42.9521741545416,-49.7176769546074,
-1.16549768778826));
#42757=CARTESIAN_POINT('Ctrl Pts',(-47.4105432027648,-50.5956823608512,
-1.36136024559355));
#42758=CARTESIAN_POINT('Ctrl Pts',(-50.6086363264877,-47.3676831528367,
-1.55722280339885));
#42759=CARTESIAN_POINT('Ctrl Pts',(-49.6890945071171,-42.9176815949843,
-1.75308536120414));
#42760=CARTESIAN_POINT('Ctrl Pts',(-45.4734860003987,-41.2216278875877,
-1.94894791900943));
#42761=CARTESIAN_POINT('Ctrl Pts',(-41.7282986823175,-43.794859117017,-2.14481047681473));
#42762=CARTESIAN_POINT('Ctrl Pts',(-41.7997119996332,-48.3383026030494,
-2.34067303462002));
#42763=CARTESIAN_POINT('Ctrl Pts',(-45.6239217216425,-50.7925607363461,
-2.53653559242531));
#42764=CARTESIAN_POINT('Ctrl Pts',(-49.7841428195107,-48.9648506157619,
-2.73239815023061));
#42765=CARTESIAN_POINT('Ctrl Pts',(-50.5633775982196,-44.4881598425256,
-2.9282607080359));
#42766=CARTESIAN_POINT('Ctrl Pts',(-47.2654095909828,-41.362240430431,-3.1241232658412));
#42767=CARTESIAN_POINT('Ctrl Pts',(-42.8368466927335,-42.379981111081,-3.31998582364649));
#42768=CARTESIAN_POINT('Ctrl Pts',(-41.2344398737399,-46.6320697906436,
-3.51584838145178));
#42769=CARTESIAN_POINT('Ctrl Pts',(-43.8898781422471,-50.3194283458399,
-3.71171093925708));
#42770=CARTESIAN_POINT('Ctrl Pts',(-48.4306293080085,-50.1475434533866,
-3.90757349706237));
#42771=CARTESIAN_POINT('Ctrl Pts',(-50.7997064691274,-46.2699876508964,
-4.10343605486766));
#42772=CARTESIAN_POINT('Ctrl Pts',(-48.8804300985944,-42.151208246751,-4.29929861267296));
#42773=CARTESIAN_POINT('Ctrl Pts',(-44.3875999794073,-41.4711765661473,
-4.49516117047825));
#42774=CARTESIAN_POINT('Ctrl Pts',(-41.3353873965154,-44.8374748217385,
-4.69102372828354));
#42775=CARTESIAN_POINT('Ctrl Pts',(-42.4508271650107,-49.2424447068201,
-4.88688628608884));
#42776=CARTESIAN_POINT('Ctrl Pts',(-46.7373166435254,-50.7504146876272,
-5.08274884389413));
#42777=CARTESIAN_POINT('Ctrl Pts',(-50.3650420187413,-48.0140714426314,
-5.27861140169942));
#42778=CARTESIAN_POINT('Ctrl Pts',(-50.0927698245969,-43.4782326790622,
-5.47447395950472));
#42779=CARTESIAN_POINT('Ctrl Pts',(-46.1637649512516,-41.195496195607,-5.67033651731001));
#42780=CARTESIAN_POINT('Ctrl Pts',(-42.0884421952216,-43.2053995648544,
-5.86619907511531));
#42781=CARTESIAN_POINT('Ctrl Pts',(-41.5079465982135,-47.7121709957002,
-6.0620616329206));
#42782=CARTESIAN_POINT('Ctrl Pts',(-44.9409275558383,-50.6891837144081,
-6.25792419072589));
#42783=CARTESIAN_POINT('Ctrl Pts',(-49.3201506663402,-49.4765899979858,
-6.45378674853118));
#42784=CARTESIAN_POINT('Ctrl Pts',(-50.7329433687539,-45.1577980618496,
-6.64964930633648));
#42785=CARTESIAN_POINT('Ctrl Pts',(-47.9170393622873,-41.5914781257455,
-6.84551186414177));
#42786=CARTESIAN_POINT('Ctrl Pts',(-43.3883208590233,-41.9640096554919,
-7.04137442194707));
#42787=CARTESIAN_POINT('Ctrl Pts',(-41.1930648262276,-45.9425306703187,
-7.23723697975236));
#42788=CARTESIAN_POINT('Ctrl Pts',(-43.2925649089103,-49.9724248955266,
-7.43309953755766));
#42789=CARTESIAN_POINT('Ctrl Pts',(-47.8111687880873,-50.4530556126673,
-7.62896209536294));
#42790=CARTESIAN_POINT('Ctrl Pts',(-50.7113289082679,-46.9551630672479,
-7.82482465316824));
#42791=CARTESIAN_POINT('Ctrl Pts',(-49.4025757140821,-42.6036420046718,
-8.02068721097354));
#42792=CARTESIAN_POINT('Ctrl Pts',(-45.0527739768292,-41.2871004410853,
-8.21654976877883));
#42793=CARTESIAN_POINT('Ctrl Pts',(-41.5512814170077,-44.1804051792425,
-8.41241232658412));
#42794=CARTESIAN_POINT('Ctrl Pts',(-42.020443960099,-48.7013832307533,-8.60827488438941));
#42795=CARTESIAN_POINT('Ctrl Pts',(-46.0536368602338,-50.8047688779136,
-8.80413744219471));
#42796=CARTESIAN_POINT('Ctrl Pts',(-48.6953045558515,-49.3495832107922,
-8.93471248073157));
#42797=CARTESIAN_POINT('Ctrl Pts',(-49.4256147683784,-48.2253962475631,
-9.));
#42798=CARTESIAN_POINT('Ctrl Pts',(-43.4267655729853,-43.7934484719077,
0.));
#42799=CARTESIAN_POINT('Ctrl Pts',(-43.3501276807105,-43.8663850881657,
-7.04753096378064E-18));
#42800=CARTESIAN_POINT('Ctrl Pts',(-43.2774225625484,-43.9429578412532,
2.53724992624095E-17));
#42801=CARTESIAN_POINT('Ctrl Pts',(-43.2086477236659,-44.0227511556538,
-4.5102810375397E-17));
#42802=CARTESIAN_POINT('Ctrl Pts',(-43.1381557104546,-44.104536754345,-1.17337751798334E-16));
#42803=CARTESIAN_POINT('Ctrl Pts',(-43.0717922910936,-44.1897061536963,
3.43486518888929E-16));
#42804=CARTESIAN_POINT('Ctrl Pts',(-43.0095809299478,-44.2778601735959,
2.84494650060196E-16));
#42805=CARTESIAN_POINT('Ctrl Pts',(-42.946054054693,-44.3678782880081,2.24255346127592E-16));
#42806=CARTESIAN_POINT('Ctrl Pts',(-42.8868562438295,-44.461009120855,7.85372393156655E-16));
#42807=CARTESIAN_POINT('Ctrl Pts',(-42.8320459022356,-44.5568700617774,
9.78384040450919E-16));
#42808=CARTESIAN_POINT('Ctrl Pts',(-42.7793850615827,-44.648971617578,1.16382633668118E-15));
#42809=CARTESIAN_POINT('Ctrl Pts',(-42.7307742307634,-44.7435941668825,
3.30656683784562E-17));
#42810=CARTESIAN_POINT('Ctrl Pts',(-42.6862990500763,-44.8404265045392,
1.11022302462516E-16));
#42811=CARTESIAN_POINT('Ctrl Pts',(-42.679886056326,-44.8543890150141,1.22263075393663E-16));
#42812=CARTESIAN_POINT('Ctrl Pts',(-42.6735591098059,-44.8683975079843,
-7.82688482717754E-16));
#42813=CARTESIAN_POINT('Ctrl Pts',(-42.6673185299068,-44.8824510861312,
-7.91033905045424E-16));
#42814=CARTESIAN_POINT('Ctrl Pts',(-42.6607681147427,-44.8972024029786,
-7.99793664851382E-16));
#42815=CARTESIAN_POINT('Ctrl Pts',(-42.6543164169337,-44.9119954067526,
-1.21324678104633E-16));
#42816=CARTESIAN_POINT('Ctrl Pts',(-42.6479647673033,-44.9268258764304,
-1.2490009027033E-16));
#42817=CARTESIAN_POINT('Ctrl Pts',(-42.6031073987511,-45.0315633671385,
-1.50150787424036E-16));
#42818=CARTESIAN_POINT('Ctrl Pts',(-42.5632161545331,-45.1382135540035,
-3.07907070874353E-16));
#42819=CARTESIAN_POINT('Ctrl Pts',(-42.528320163891,-45.2463469640437,-2.08166817117217E-16));
#42820=CARTESIAN_POINT('Ctrl Pts',(-42.4929026061891,-45.3560965719249,
-1.06935812418896E-16));
#42821=CARTESIAN_POINT('Ctrl Pts',(-42.4626302928821,-45.4673747834446,
-2.85605705579807E-16));
#42822=CARTESIAN_POINT('Ctrl Pts',(-42.4375733579101,-45.5797690551028,
-4.9960036108132E-16));
#42823=CARTESIAN_POINT('Ctrl Pts',(-42.4112968134939,-45.6976339525716,
-7.24010891595492E-16));
#42824=CARTESIAN_POINT('Ctrl Pts',(-42.3907548535477,-45.8167269609219,
-4.47609461766868E-17));
#42825=CARTESIAN_POINT('Ctrl Pts',(-42.376082068452,-45.9366009615454,-5.55111512312578E-17));
#42826=CARTESIAN_POINT('Ctrl Pts',(-42.3650774796302,-46.0265064620131,
-6.35738050221861E-17));
#42827=CARTESIAN_POINT('Ctrl Pts',(-42.357375378577,-46.1168519806525,6.6117506257439E-16));
#42828=CARTESIAN_POINT('Ctrl Pts',(-42.3530552551646,-46.2074543300699,
7.21644966006352E-16));
#42829=CARTESIAN_POINT('Ctrl Pts',(-42.3521018391375,-46.2274495301548,
7.3499018084909E-16));
#42830=CARTESIAN_POINT('Ctrl Pts',(-42.3513132407974,-46.2474596005774,
-3.23104951562236E-16));
#42831=CARTESIAN_POINT('Ctrl Pts',(-42.3506909145217,-46.2674588278385,
-3.05311331771918E-16));
#42832=CARTESIAN_POINT('Ctrl Pts',(-42.3470030310376,-46.3859735407681,
-1.99866970652492E-16));
#42833=CARTESIAN_POINT('Ctrl Pts',(-42.3491403257791,-46.5042833521836,
-9.63231096175936E-16));
#42834=CARTESIAN_POINT('Ctrl Pts',(-42.3571688004525,-46.621960666869,-8.60422844084496E-16));
#42835=CARTESIAN_POINT('Ctrl Pts',(-42.3651713582012,-46.7392581044026,
-7.57946469943304E-16));
#42836=CARTESIAN_POINT('Ctrl Pts',(-42.3790267977734,-46.8559280062375,
-2.07758591149402E-16));
#42837=CARTESIAN_POINT('Ctrl Pts',(-42.3988487192012,-46.9715644449789,
-2.4980018054066E-16));
#42838=CARTESIAN_POINT('Ctrl Pts',(-42.4014018331404,-46.9864587126565,
-2.55215244276644E-16));
#42839=CARTESIAN_POINT('Ctrl Pts',(-42.4040540013104,-47.0013358483328,
-4.57968684642233E-16));
#42840=CARTESIAN_POINT('Ctrl Pts',(-42.406805529256,-47.0161949940318,-4.71844785465692E-16));
#42841=CARTESIAN_POINT('Ctrl Pts',(-42.4276985069981,-47.1290238682075,
-5.79779039420077E-16));
#42842=CARTESIAN_POINT('Ctrl Pts',(-42.4543158977961,-47.2408157327732,
-3.25103491011084E-16));
#42843=CARTESIAN_POINT('Ctrl Pts',(-42.486359445728,-47.3513087526731,-4.16333634234434E-16));
#42844=CARTESIAN_POINT('Ctrl Pts',(-42.5065690808814,-47.4209959054168,
-4.73871829238813E-16));
#42845=CARTESIAN_POINT('Ctrl Pts',(-42.5289381902425,-47.4901664003336,
-2.57699975902937E-16));
#42846=CARTESIAN_POINT('Ctrl Pts',(-42.5534023261536,-47.5587530205468,
-3.33066907387547E-16));
#42847=CARTESIAN_POINT('Ctrl Pts',(-42.5620444221668,-47.5829816366427,
-3.59690707242276E-16));
#42848=CARTESIAN_POINT('Ctrl Pts',(-42.5709480252132,-47.607137374388,-1.17515466282303E-15));
#42849=CARTESIAN_POINT('Ctrl Pts',(-42.5801105172574,-47.631217207197,-1.22124532708767E-15));
#42850=CARTESIAN_POINT('Ctrl Pts',(-42.5859847085885,-47.6466550972885,
-1.25079464392915E-15));
#42851=CARTESIAN_POINT('Ctrl Pts',(-42.5919639441197,-47.6620580726081,
-1.28683390958385E-16));
#42852=CARTESIAN_POINT('Ctrl Pts',(-42.598043751014,-47.6774164867468,-1.38777878078145E-16));
#42853=CARTESIAN_POINT('Ctrl Pts',(-42.6409188983819,-47.7857249052508,
-2.09964780949104E-16));
#42854=CARTESIAN_POINT('Ctrl Pts',(-42.6888409885308,-47.8919483371788,
-6.43124410407582E-16));
#42855=CARTESIAN_POINT('Ctrl Pts',(-42.741455861339,-47.9958307028328,-5.55111512312578E-16));
#42856=CARTESIAN_POINT('Ctrl Pts',(-42.7959148678593,-48.1033541106933,
-4.64013791546623E-16));
#42857=CARTESIAN_POINT('Ctrl Pts',(-42.8554014994299,-48.2083701489123,
3.64463956063111E-16));
#42858=CARTESIAN_POINT('Ctrl Pts',(-42.9195789519365,-48.3105914458752,
3.88578058618805E-16));
#42859=CARTESIAN_POINT('Ctrl Pts',(-42.98445195249,-48.4139206058127,4.12953507118863E-16));
#42860=CARTESIAN_POINT('Ctrl Pts',(-43.054118381845,-48.5143948787197,-3.61504930637615E-16));
#42861=CARTESIAN_POINT('Ctrl Pts',(-43.1282823985727,-48.61170300331,-3.33066907387547E-16));
#42862=CARTESIAN_POINT('Ctrl Pts',(-43.1809810456532,-48.6808471346839,
-3.1285973122524E-16));
#42863=CARTESIAN_POINT('Ctrl Pts',(-43.2359516673225,-48.7483923767087,
-1.30566376976968E-16));
#42864=CARTESIAN_POINT('Ctrl Pts',(-43.2931021569972,-48.8142194330436,
-5.55111512312578E-17));
#42865=CARTESIAN_POINT('Ctrl Pts',(-43.3103693212538,-48.8341080919287,
-3.28343392102748E-17));
#42866=CARTESIAN_POINT('Ctrl Pts',(-43.3278355504843,-48.8538398517485,
-4.86517584915369E-16));
#42867=CARTESIAN_POINT('Ctrl Pts',(-43.345498492003,-48.873411273902,-4.9960036108132E-16));
#42868=CARTESIAN_POINT('Ctrl Pts',(-43.3628813133451,-48.8926723088969,
-5.124756548431E-16));
#42869=CARTESIAN_POINT('Ctrl Pts',(-43.3804583525997,-48.9117818491587,
-2.10886016998155E-16));
#42870=CARTESIAN_POINT('Ctrl Pts',(-43.3982056633207,-48.9307137415863,
-2.22044604925031E-16));
#42871=CARTESIAN_POINT('Ctrl Pts',(-43.4838655638276,-49.0220911929223,
-2.75903104764051E-16));
#42872=CARTESIAN_POINT('Ctrl Pts',(-43.5735673629197,-49.1094227285799,
1.55779886598745E-16));
#42873=CARTESIAN_POINT('Ctrl Pts',(-43.6669817278709,-49.1923921170496,
-5.55111512312578E-17));
#42874=CARTESIAN_POINT('Ctrl Pts',(-43.7477796843816,-49.2641557804304,
-2.38265528404594E-16));
#42875=CARTESIAN_POINT('Ctrl Pts',(-43.8313561093309,-49.3326560699961,
-5.06042579863952E-16));
#42876=CARTESIAN_POINT('Ctrl Pts',(-43.9175245994745,-49.3976724621237,
-7.21644966006352E-16));
#42877=CARTESIAN_POINT('Ctrl Pts',(-43.9569256379766,-49.4274015819587,
-8.20230399073553E-16));
#42878=CARTESIAN_POINT('Ctrl Pts',(-43.9968689485439,-49.4564020376285,
-5.36268313194471E-16));
#42879=CARTESIAN_POINT('Ctrl Pts',(-44.0373382028386,-49.4846513724122,
-5.55111512312578E-16));
#42880=CARTESIAN_POINT('Ctrl Pts',(-44.0558574998406,-49.4975786632676,
-5.63734423878843E-16));
#42881=CARTESIAN_POINT('Ctrl Pts',(-44.0744888929508,-49.5103499540868,
3.11047644558593E-16));
#42882=CARTESIAN_POINT('Ctrl Pts',(-44.093224584765,-49.5229588001047,2.77555756156289E-16));
#42883=CARTESIAN_POINT('Ctrl Pts',(-44.1981798849433,-49.5935921789969,
8.99378536162834E-17));
#42884=CARTESIAN_POINT('Ctrl Pts',(-44.3062422017772,-49.6590224223094,
-6.83717929618714E-16));
#42885=CARTESIAN_POINT('Ctrl Pts',(-44.4171004727898,-49.7189173286392,
-4.9960036108132E-16));
#42886=CARTESIAN_POINT('Ctrl Pts',(-44.5269320414255,-49.7782575245074,
-3.17187978305053E-16));
#42887=CARTESIAN_POINT('Ctrl Pts',(-44.6395085962919,-49.8321651371395,
-3.46914076603539E-16));
#42888=CARTESIAN_POINT('Ctrl Pts',(-44.7545630653622,-49.880281181818,-2.77555756156289E-16));
#42889=CARTESIAN_POINT('Ctrl Pts',(-44.8154787832058,-49.9057562757025,
-2.40833915513258E-16));
#42890=CARTESIAN_POINT('Ctrl Pts',(-44.8770896512138,-49.9296072179812,
-2.58827617428343E-16));
#42891=CARTESIAN_POINT('Ctrl Pts',(-44.9393355849193,-49.9518501705994,
-2.77555756156289E-16));
#42892=CARTESIAN_POINT('Ctrl Pts',(-49.3879806100937,-46.0027475395409,
-2.01601780324957));
#42893=CARTESIAN_POINT('Ctrl Pts',(-49.3905754410883,-46.3290880943019,
-1.99688706151736));
#42894=CARTESIAN_POINT('Ctrl Pts',(-49.3471327586953,-46.6547522859376,
-1.97775631978515));
#42895=CARTESIAN_POINT('Ctrl Pts',(-49.2547938342684,-46.965905399372,-1.95862557805294));
#42896=CARTESIAN_POINT('Ctrl Pts',(-48.9396686084859,-48.0277782307101,
-1.8933380587845));
#42897=CARTESIAN_POINT('Ctrl Pts',(-48.0550716141049,-48.9206472894915,
-1.82805053951607));
#42898=CARTESIAN_POINT('Ctrl Pts',(-46.9961775852451,-49.2456530622191,
-1.76276302024764));
#42899=CARTESIAN_POINT('Ctrl Pts',(-45.9372835563853,-49.5706588349466,
-1.69747550097921));
#42900=CARTESIAN_POINT('Ctrl Pts',(-44.7040924930467,-49.3278013216202,
-1.63218798171078));
#42901=CARTESIAN_POINT('Ctrl Pts',(-43.8475129257691,-48.6255466875836,
-1.56690046244235));
#42902=CARTESIAN_POINT('Ctrl Pts',(-42.9909333584915,-47.923292053547,-1.50161294317392));
#42903=CARTESIAN_POINT('Ctrl Pts',(-42.5109652872749,-46.7616402988001,
-1.43632542390549));
#42904=CARTESIAN_POINT('Ctrl Pts',(-42.6220168848379,-45.6595897311541,
-1.37103790463705));
#42905=CARTESIAN_POINT('Ctrl Pts',(-42.733068482401,-44.5575391635081,-1.30575038536862));
#42906=CARTESIAN_POINT('Ctrl Pts',(-43.4351397487436,-43.5150897829631,
-1.24046286610019));
#42907=CARTESIAN_POINT('Ctrl Pts',(-44.4146108931053,-42.9978281634854,
-1.17517534683176));
#42908=CARTESIAN_POINT('Ctrl Pts',(-45.394082037467,-42.4805665440078,-1.10988782756333));
#42909=CARTESIAN_POINT('Ctrl Pts',(-46.6509530598478,-42.4884926855974,
-1.0446003082949));
#42910=CARTESIAN_POINT('Ctrl Pts',(-47.6237060458603,-43.0182858736907,
-0.979312789026467));
#42911=CARTESIAN_POINT('Ctrl Pts',(-48.5964590318727,-43.5480790617839,
-0.914025269758036));
#42912=CARTESIAN_POINT('Ctrl Pts',(-49.2850939815168,-44.5997392963807,
-0.848737750489605));
#42913=CARTESIAN_POINT('Ctrl Pts',(-49.3820477911778,-45.7030074740777,
-0.783450231221174));
#42914=CARTESIAN_POINT('Ctrl Pts',(-49.3906770071057,-45.8012020614281,
-0.777639421897305));
#42915=CARTESIAN_POINT('Ctrl Pts',(-49.3946191616459,-45.8998054662665,
-0.771828612573436));
#42916=CARTESIAN_POINT('Ctrl Pts',(-49.3940299756876,-45.9984545908008,
-0.766017803249567));
#42917=CARTESIAN_POINT('Ctrl Pts',(-47.0579044229729,-49.9456385074984,
5.55111512312578E-16));
#42918=CARTESIAN_POINT('Ctrl Pts',(-48.3527480267224,-49.5984650974504,
-0.0652875192684306));
#42919=CARTESIAN_POINT('Ctrl Pts',(-50.5530323995854,-47.5357692714295,
-0.195862557805293));
#42920=CARTESIAN_POINT('Ctrl Pts',(-49.798918270059,-43.0499899242987,-0.391725115610586));
#42921=CARTESIAN_POINT('Ctrl Pts',(-45.6441921539078,-41.2067322013831,
-0.58758767341588));
#42922=CARTESIAN_POINT('Ctrl Pts',(-41.8104753331013,-43.6427683056469,
-0.783450231221174));
#42923=CARTESIAN_POINT('Ctrl Pts',(-41.7184180535194,-48.1865095079258,
-0.979312789026466));
#42924=CARTESIAN_POINT('Ctrl Pts',(-45.4525334082598,-50.7759013692154,
-1.17517534683176));
#42925=CARTESIAN_POINT('Ctrl Pts',(-49.6754254318228,-49.098593633004,-1.37103790463705));
#42926=CARTESIAN_POINT('Ctrl Pts',(-50.6146438233287,-44.6526230577962,
-1.56690046244235));
#42927=CARTESIAN_POINT('Ctrl Pts',(-47.4307680051951,-41.41057421285,-1.76276302024764));
#42928=CARTESIAN_POINT('Ctrl Pts',(-42.9685984702712,-42.2689561020525,
-1.95862557805293));
#42929=CARTESIAN_POINT('Ctrl Pts',(-41.2148490309835,-46.4609045794214,
-2.15448813585823));
#42930=CARTESIAN_POINT('Ctrl Pts',(-43.7364585340961,-50.2410417148001,
-2.35035069366352));
#42931=CARTESIAN_POINT('Ctrl Pts',(-48.2804504821097,-50.2319761154881,
-2.54621325146882));
#42932=CARTESIAN_POINT('Ctrl Pts',(-50.7869498812151,-46.4417996865353,
-2.74207580927411));
#42933=CARTESIAN_POINT('Ctrl Pts',(-49.0164920780277,-42.2568934559197,
-2.9379383670794));
#42934=CARTESIAN_POINT('Ctrl Pts',(-44.5509149516467,-41.4163086543115,
-3.1338009248847));
#42935=CARTESIAN_POINT('Ctrl Pts',(-41.3800394184348,-44.6710764629181,
-3.32966348268999));
#42936=CARTESIAN_POINT('Ctrl Pts',(-42.3369215031958,-49.1131863035692,
-3.52552604049529));
#42937=CARTESIAN_POINT('Ctrl Pts',(-46.5666235775808,-50.7737837298756,
-3.72138859830058));
#42938=CARTESIAN_POINT('Ctrl Pts',(-50.2900692643348,-48.1691885628536,
-3.91725115610587));
#42939=CARTESIAN_POINT('Ctrl Pts',(-50.180502688043,-43.6265066797266,-4.11311371391116));
#42940=CARTESIAN_POINT('Ctrl Pts',(-46.3358174043579,-41.204449981662,-4.30897627171646));
#42941=CARTESIAN_POINT('Ctrl Pts',(-42.1910921533903,-43.0670331890375,
-4.50483882952175));
#42942=CARTESIAN_POINT('Ctrl Pts',(-41.4494798905217,-47.5501096808741,
-4.70070138732705));
#42943=CARTESIAN_POINT('Ctrl Pts',(-44.7735827067234,-50.6482226625802,
-4.89656394513233));
#42944=CARTESIAN_POINT('Ctrl Pts',(-49.1934423111539,-49.5933270812414,
-5.09242650293764));
#42945=CARTESIAN_POINT('Ctrl Pts',(-50.7600837602575,-45.3279316541825,
-5.28828906074292));
#42946=CARTESIAN_POINT('Ctrl Pts',(-48.0737730601331,-41.6630035036824,
-5.48415161854822));
#42947=CARTESIAN_POINT('Ctrl Pts',(-43.5346256929101,-41.8730152769562,
-5.68001417635351));
#42948=CARTESIAN_POINT('Ctrl Pts',(-41.1981957029014,-45.7703295255252,
-5.87587673415881));
#42949=CARTESIAN_POINT('Ctrl Pts',(-43.1519934739611,-49.8728455133488,
-6.0717392919641));
#42950=CARTESIAN_POINT('Ctrl Pts',(-47.6503759783394,-50.5151226960096,
-6.26760184976939));
#42951=CARTESIAN_POINT('Ctrl Pts',(-50.6742104721782,-47.1233109626991,
-6.46346440757469));
#42952=CARTESIAN_POINT('Ctrl Pts',(-49.5218181321677,-42.7278641268702,
-6.65932696537998));
#42953=CARTESIAN_POINT('Ctrl Pts',(-45.2228147324014,-41.2559448461001,
-6.85518952318528));
#42954=CARTESIAN_POINT('Ctrl Pts',(-41.6182000513892,-44.022657337512,-7.05105208099056));
#42955=CARTESIAN_POINT('Ctrl Pts',(-41.9285482915987,-48.5560484764118,
-7.24691463879586));
#42956=CARTESIAN_POINT('Ctrl Pts',(-45.8765970410433,-50.8057107187776,
-7.44277719660115));
#42957=CARTESIAN_POINT('Ctrl Pts',(-49.9348716345255,-48.761650115466,-7.63863975440645));
#42958=CARTESIAN_POINT('Ctrl Pts',(-50.4775506806467,-44.2501708246775,
-7.83450231221174));
#42959=CARTESIAN_POINT('Ctrl Pts',(-47.0195848331003,-41.3020769083036,
-8.03036487001704));
#42960=CARTESIAN_POINT('Ctrl Pts',(-42.6509149775089,-42.5514375357737,
-8.22622742782233));
#42961=CARTESIAN_POINT('Ctrl Pts',(-41.2740009567628,-46.8818734807212,
-8.42208998562762));
#42962=CARTESIAN_POINT('Ctrl Pts',(-44.1206550171574,-50.4245588063534,
-8.61795254343291));
#42963=CARTESIAN_POINT('Ctrl Pts',(-48.6442455574373,-50.0137240618373,
-8.81381510123821));
#42964=CARTESIAN_POINT('Ctrl Pts',(-50.8097851438853,-46.0175025423462,
-9.0096776590435));
#42965=CARTESIAN_POINT('Ctrl Pts',(-48.6687263145852,-42.0041782891898,
-9.2055402168488));
#42966=CARTESIAN_POINT('Ctrl Pts',(-45.6668068080595,-41.7135846407913,
-9.33611525538566));
#42967=CARTESIAN_POINT('Ctrl Pts',(-44.4292895827202,-42.2290460377978,
-9.40140277465409));
#42968=CARTESIAN_POINT('Ctrl Pts',(-46.9978874462229,-49.7217947561856,
0.133800924884696));
#42969=CARTESIAN_POINT('Ctrl Pts',(-48.219272052379,-49.3943171693393,0.0685134056162651));
#42970=CARTESIAN_POINT('Ctrl Pts',(-50.2947300106983,-47.4486420918325,
-0.0620616329205972));
#42971=CARTESIAN_POINT('Ctrl Pts',(-49.5833982433549,-43.2173497370389,
-0.257924190725891));
#42972=CARTESIAN_POINT('Ctrl Pts',(-45.6643778254701,-41.4786636119901,
-0.453786748531184));
#42973=CARTESIAN_POINT('Ctrl Pts',(-42.0481552208745,-43.7764986471809,
-0.649649306336477));
#42974=CARTESIAN_POINT('Ctrl Pts',(-41.9613205299201,-48.0624645682778,
-0.845511864141771));
#42975=CARTESIAN_POINT('Ctrl Pts',(-45.4835922534583,-50.504955189946,-1.04137442194706));
#42976=CARTESIAN_POINT('Ctrl Pts',(-49.4669113941667,-48.922804385893,-1.23723697975236));
#42977=CARTESIAN_POINT('Ctrl Pts',(-50.352846098468,-44.7290623739175,-1.43309953755765));
#42978=CARTESIAN_POINT('Ctrl Pts',(-47.3495977517792,-41.6709412694405,
-1.62896209536294));
#42979=CARTESIAN_POINT('Ctrl Pts',(-43.140575778598,-42.4806254835333,-1.82482465316824));
#42980=CARTESIAN_POINT('Ctrl Pts',(-41.4863199580507,-46.434756565644,-2.02068721097353));
#42981=CARTESIAN_POINT('Ctrl Pts',(-43.8648736466354,-50.0004391646398,
-2.21654976877883));
#42982=CARTESIAN_POINT('Ctrl Pts',(-48.1510760881736,-49.9918878744197,
-2.41241232658412));
#42983=CARTESIAN_POINT('Ctrl Pts',(-50.5153768983579,-46.4167355305122,
-2.60827488438941));
#42984=CARTESIAN_POINT('Ctrl Pts',(-48.845360611912,-42.4692471747913,-2.80413744219471));
#42985=CARTESIAN_POINT('Ctrl Pts',(-44.6331243665686,-41.6763503848778,
-3.));
#42986=CARTESIAN_POINT('Ctrl Pts',(-41.6421387733376,-44.7464688814539,
-3.19586255780529));
#42987=CARTESIAN_POINT('Ctrl Pts',(-42.5447350751993,-48.9365691858576,
-3.39172511561059));
#42988=CARTESIAN_POINT('Ctrl Pts',(-46.5344779192933,-50.5029576884072,
-3.58758767341588));
#42989=CARTESIAN_POINT('Ctrl Pts',(-50.0466852858747,-48.0461262741287,
-3.78345023122117));
#42990=CARTESIAN_POINT('Ctrl Pts',(-49.9433346346883,-43.7611595749465,
-3.97931278902647));
#42991=CARTESIAN_POINT('Ctrl Pts',(-46.3167658294595,-41.4765108670353,
-4.17517534683176));
#42992=CARTESIAN_POINT('Ctrl Pts',(-42.4071789082133,-43.2334261042004,
-4.37103790463705));
#42993=CARTESIAN_POINT('Ctrl Pts',(-41.7076397523018,-47.4621689419408,
-4.56690046244235));
#42994=CARTESIAN_POINT('Ctrl Pts',(-44.8431597465561,-50.3845199448194,
-4.76276302024764));
#42995=CARTESIAN_POINT('Ctrl Pts',(-49.0122721139422,-49.3894706427891,
-4.95862557805293));
#42996=CARTESIAN_POINT('Ctrl Pts',(-50.4900349447276,-45.3660593993828,
-5.15448813585823));
#42997=CARTESIAN_POINT('Ctrl Pts',(-47.95612387857,-41.9090497553401,-5.35035069366352));
#42998=CARTESIAN_POINT('Ctrl Pts',(-43.6744911753258,-42.1071471520028,
-5.54621325146882));
#42999=CARTESIAN_POINT('Ctrl Pts',(-41.4706114056805,-45.7833591785141,
-5.7420758092741));
#43000=CARTESIAN_POINT('Ctrl Pts',(-43.3135664268153,-49.6531314502598,
-5.93793836707941));
#43001=CARTESIAN_POINT('Ctrl Pts',(-47.5567469372182,-50.2589709983841,
-6.13380092488469));
#43002=CARTESIAN_POINT('Ctrl Pts',(-50.4090334154029,-47.0595833456598,
-6.32966348269));
#43003=CARTESIAN_POINT('Ctrl Pts',(-49.3220185355631,-42.9134987630019,
-6.52552604049528));
#43004=CARTESIAN_POINT('Ctrl Pts',(-45.2669059651471,-41.5250843275974,
-6.72138859830058));
#43005=CARTESIAN_POINT('Ctrl Pts',(-41.8667880900894,-44.1348358349494,
-6.91725115610587));
#43006=CARTESIAN_POINT('Ctrl Pts',(-42.1595296706494,-48.4110388719054,
-7.11311371391116));
#43007=CARTESIAN_POINT('Ctrl Pts',(-45.8835979310649,-50.5330733970942,
-7.30897627171647));
#43008=CARTESIAN_POINT('Ctrl Pts',(-49.7116387088703,-48.6049763298456,
-7.50483882952174));
#43009=CARTESIAN_POINT('Ctrl Pts',(-50.2235305165733,-44.3494420392139,
-7.70070138732705));
#43010=CARTESIAN_POINT('Ctrl Pts',(-46.9617418012592,-41.5685992281323,
-7.89656394513233));
#43011=CARTESIAN_POINT('Ctrl Pts',(-42.840915088638,-42.7470811957699,-8.09242650293763));
#43012=CARTESIAN_POINT('Ctrl Pts',(-41.5421160799624,-46.8318430819068,
-8.28828906074292));
#43013=CARTESIAN_POINT('Ctrl Pts',(-44.2272739155108,-50.1735449744385,
-8.48415161854822));
#43014=CARTESIAN_POINT('Ctrl Pts',(-48.4942323608801,-49.7860176845225,
-8.68001417635351));
#43015=CARTESIAN_POINT('Ctrl Pts',(-50.5369166721361,-46.0165095890564,
-8.8758767341588));
#43016=CARTESIAN_POINT('Ctrl Pts',(-48.5173242770319,-42.2308690312902,
-9.0717392919641));
#43017=CARTESIAN_POINT('Ctrl Pts',(-45.6857095062803,-41.9567613261026,
-9.20231433050096));
#43018=CARTESIAN_POINT('Ctrl Pts',(-44.5183990415218,-42.4429795948946,
-9.26760184976939));
#43019=CARTESIAN_POINT('Ctrl Pts',(-46.9378704694728,-49.4979510048728,
0.267601849769392));
#43020=CARTESIAN_POINT('Ctrl Pts',(-48.0857960780355,-49.1901692412281,
0.202314330500961));
#43021=CARTESIAN_POINT('Ctrl Pts',(-50.0364276218112,-47.3615149122355,
0.0717392919640985));
#43022=CARTESIAN_POINT('Ctrl Pts',(-49.3678782166508,-43.3847095497791,
-0.124123265841195));
#43023=CARTESIAN_POINT('Ctrl Pts',(-45.6845634970324,-41.750595022597,-0.319985823646488));
#43024=CARTESIAN_POINT('Ctrl Pts',(-42.2858351086478,-43.9102289887149,
-0.515848381451782));
#43025=CARTESIAN_POINT('Ctrl Pts',(-42.2042230063208,-47.9384196286299,
-0.711710939257077));
#43026=CARTESIAN_POINT('Ctrl Pts',(-45.5146510986568,-50.2340090106765,
-0.907573497062368));
#43027=CARTESIAN_POINT('Ctrl Pts',(-49.2583973565106,-48.7470151387819,
-1.10343605486766));
#43028=CARTESIAN_POINT('Ctrl Pts',(-50.0910483736072,-44.8055016900389,
-1.29929861267296));
#43029=CARTESIAN_POINT('Ctrl Pts',(-47.2684274983633,-41.9313083260309,
-1.49516117047825));
#43030=CARTESIAN_POINT('Ctrl Pts',(-43.3125530869246,-42.6922948650142,
-1.69102372828354));
#43031=CARTESIAN_POINT('Ctrl Pts',(-41.757790885118,-46.4086085518666,-1.88688628608884));
#43032=CARTESIAN_POINT('Ctrl Pts',(-43.9932887591747,-49.7598366144794,
-2.08274884389413));
#43033=CARTESIAN_POINT('Ctrl Pts',(-48.0217016942375,-49.7517996333514,
-2.27861140169942));
#43034=CARTESIAN_POINT('Ctrl Pts',(-50.2438039155007,-46.391671374489,-2.47447395950472));
#43035=CARTESIAN_POINT('Ctrl Pts',(-48.6742291457962,-42.681600893663,-2.67033651731001));
#43036=CARTESIAN_POINT('Ctrl Pts',(-44.7153337814905,-41.936392115444,-2.8661990751153));
#43037=CARTESIAN_POINT('Ctrl Pts',(-41.9042381282403,-44.8218612999897,
-3.0620616329206));
#43038=CARTESIAN_POINT('Ctrl Pts',(-42.7525486472029,-48.7599520681459,
-3.25792419072589));
#43039=CARTESIAN_POINT('Ctrl Pts',(-46.5023322610058,-50.2321316469387,
-3.45378674853119));
#43040=CARTESIAN_POINT('Ctrl Pts',(-49.8033013074145,-47.9230639854038,
-3.64964930633647));
#43041=CARTESIAN_POINT('Ctrl Pts',(-49.7061665813336,-43.8958124701664,
-3.84551186414177));
#43042=CARTESIAN_POINT('Ctrl Pts',(-46.2977142545611,-41.7485717524086,
-4.04137442194706));
#43043=CARTESIAN_POINT('Ctrl Pts',(-42.6232656630362,-43.3998190193633,
-4.23723697975236));
#43044=CARTESIAN_POINT('Ctrl Pts',(-41.9657996140819,-47.3742282030075,
-4.43309953755765));
#43045=CARTESIAN_POINT('Ctrl Pts',(-44.9127367863888,-50.1208172270585,
-4.62896209536295));
#43046=CARTESIAN_POINT('Ctrl Pts',(-48.8311019167305,-49.1856142043368,
-4.82482465316824));
#43047=CARTESIAN_POINT('Ctrl Pts',(-50.2199861291977,-45.4041871445831,
-5.02068721097353));
#43048=CARTESIAN_POINT('Ctrl Pts',(-47.8384746970067,-42.1550960069977,
-5.21654976877883));
#43049=CARTESIAN_POINT('Ctrl Pts',(-43.8143566577415,-42.3412790270494,
-5.41241232658412));
#43050=CARTESIAN_POINT('Ctrl Pts',(-41.7430271084595,-45.7963888315029,
-5.60827488438941));
#43051=CARTESIAN_POINT('Ctrl Pts',(-43.4751393796696,-49.4334173871708,
-5.80413744219471));
#43052=CARTESIAN_POINT('Ctrl Pts',(-47.463117896097,-50.0028193007586,-6.));
#43053=CARTESIAN_POINT('Ctrl Pts',(-50.1438563586276,-46.9958557286205,
-6.19586255780529));
#43054=CARTESIAN_POINT('Ctrl Pts',(-49.1222189389585,-43.0991333991335,
-6.39172511561059));
#43055=CARTESIAN_POINT('Ctrl Pts',(-45.3109971978927,-41.7942238090946,
-6.58758767341588));
#43056=CARTESIAN_POINT('Ctrl Pts',(-42.1153761287897,-44.2470143323867,
-6.78345023122118));
#43057=CARTESIAN_POINT('Ctrl Pts',(-42.3905110497,-48.266029267399,-6.97931278902647));
#43058=CARTESIAN_POINT('Ctrl Pts',(-45.8905988210865,-50.2604360754108,
-7.17517534683176));
#43059=CARTESIAN_POINT('Ctrl Pts',(-49.4884057832152,-48.4483025442253,
-7.37103790463705));
#43060=CARTESIAN_POINT('Ctrl Pts',(-49.9695103524998,-44.4487132537502,
-7.56690046244235));
#43061=CARTESIAN_POINT('Ctrl Pts',(-46.9038987694181,-41.8351215479612,
-7.76276302024765));
#43062=CARTESIAN_POINT('Ctrl Pts',(-43.030915199767,-42.942724855766,-7.95862557805293));
#43063=CARTESIAN_POINT('Ctrl Pts',(-41.8102312031619,-46.7818126830923,
-8.15448813585824));
#43064=CARTESIAN_POINT('Ctrl Pts',(-44.3338928138642,-49.9225311425236,
-8.35035069366352));
#43065=CARTESIAN_POINT('Ctrl Pts',(-48.3442191643229,-49.5583113072078,
-8.54621325146882));
#43066=CARTESIAN_POINT('Ctrl Pts',(-50.2640482003868,-46.0155166357666,
-8.74207580927411));
#43067=CARTESIAN_POINT('Ctrl Pts',(-48.3659222394787,-42.4575597733907,
-8.93793836707941));
#43068=CARTESIAN_POINT('Ctrl Pts',(-45.7046122045012,-42.1999380114139,
-9.06851340561627));
#43069=CARTESIAN_POINT('Ctrl Pts',(-44.6075085003234,-42.6569131519913,
-9.1338009248847));
#43070=CARTESIAN_POINT('Ctrl Pts',(-46.8778534927228,-49.27410725356,0.401402774654088));
#43071=CARTESIAN_POINT('Ctrl Pts',(-47.9523201036921,-48.9860213131169,
0.336115255385657));
#43072=CARTESIAN_POINT('Ctrl Pts',(-49.7781252329241,-47.2743877326385,
0.205540216848794));
#43073=CARTESIAN_POINT('Ctrl Pts',(-49.1523581899468,-43.5520693625194,
0.00967765904350067));
#43074=CARTESIAN_POINT('Ctrl Pts',(-45.7047491685946,-42.0225264332039,
-0.186184898761793));
#43075=CARTESIAN_POINT('Ctrl Pts',(-42.5235149964211,-44.0439593302489,
-0.382047456567086));
#43076=CARTESIAN_POINT('Ctrl Pts',(-42.4471254827216,-47.814374688982,-0.57791001437238));
#43077=CARTESIAN_POINT('Ctrl Pts',(-45.5457099438552,-49.963062831407,-0.773772572177673));
#43078=CARTESIAN_POINT('Ctrl Pts',(-49.0498833188546,-48.5712258916709,
-0.969635129982967));
#43079=CARTESIAN_POINT('Ctrl Pts',(-49.8292506487463,-44.8819410061602,
-1.16549768778826));
#43080=CARTESIAN_POINT('Ctrl Pts',(-47.1872572449474,-42.1916753826214,
-1.36136024559355));
#43081=CARTESIAN_POINT('Ctrl Pts',(-43.4845303952514,-42.9039642464951,
-1.55722280339885));
#43082=CARTESIAN_POINT('Ctrl Pts',(-42.0292618121851,-46.3824605380891,
-1.75308536120414));
#43083=CARTESIAN_POINT('Ctrl Pts',(-44.1217038717141,-49.5192340643191,
-1.94894791900943));
#43084=CARTESIAN_POINT('Ctrl Pts',(-47.8923273003014,-49.5117113922829,
-2.14481047681473));
#43085=CARTESIAN_POINT('Ctrl Pts',(-49.9722309326436,-46.3666072184659,
-2.34067303462002));
#43086=CARTESIAN_POINT('Ctrl Pts',(-48.5030976796804,-42.8939546125346,
-2.53653559242531));
#43087=CARTESIAN_POINT('Ctrl Pts',(-44.7975431964124,-42.1964338460104,
-2.73239815023061));
#43088=CARTESIAN_POINT('Ctrl Pts',(-42.166337483143,-44.8972537185255,-2.9282607080359));
#43089=CARTESIAN_POINT('Ctrl Pts',(-42.9603622192064,-48.5833349504342,
-3.1241232658412));
#43090=CARTESIAN_POINT('Ctrl Pts',(-46.4701866027183,-49.9613056054703,
-3.31998582364649));
#43091=CARTESIAN_POINT('Ctrl Pts',(-49.5599173289544,-47.8000016966788,
-3.51584838145178));
#43092=CARTESIAN_POINT('Ctrl Pts',(-49.4689985279789,-44.0304653653864,
-3.71171093925708));
#43093=CARTESIAN_POINT('Ctrl Pts',(-46.2786626796627,-42.0206326377818,
-3.90757349706237));
#43094=CARTESIAN_POINT('Ctrl Pts',(-42.8393524178592,-43.5662119345263,
-4.10343605486766));
#43095=CARTESIAN_POINT('Ctrl Pts',(-42.2239594758619,-47.2862874640742,
-4.29929861267296));
#43096=CARTESIAN_POINT('Ctrl Pts',(-44.9823138262216,-49.8571145092977,
-4.49516117047825));
#43097=CARTESIAN_POINT('Ctrl Pts',(-48.6499317195187,-48.9817577658845,
-4.69102372828354));
#43098=CARTESIAN_POINT('Ctrl Pts',(-49.9499373136678,-45.4423148897834,
-4.88688628608884));
#43099=CARTESIAN_POINT('Ctrl Pts',(-47.7208255154434,-42.4011422586555,
-5.08274884389413));
#43100=CARTESIAN_POINT('Ctrl Pts',(-43.9542221401571,-42.575410902096,-5.27861140169943));
#43101=CARTESIAN_POINT('Ctrl Pts',(-42.0154428112387,-45.8094184844919,
-5.47447395950472));
#43102=CARTESIAN_POINT('Ctrl Pts',(-43.6367123325237,-49.2137033240818,
-5.67033651731001));
#43103=CARTESIAN_POINT('Ctrl Pts',(-47.3694888549758,-49.7466676031331,
-5.86619907511531));
#43104=CARTESIAN_POINT('Ctrl Pts',(-49.8786793018522,-46.9321281115812,
-6.0620616329206));
#43105=CARTESIAN_POINT('Ctrl Pts',(-48.9224193423538,-43.2847680352652,
-6.25792419072589));
#43106=CARTESIAN_POINT('Ctrl Pts',(-45.3550884306384,-42.0633632905919,
-6.45378674853118));
#43107=CARTESIAN_POINT('Ctrl Pts',(-42.3639641674899,-44.3591928298241,
-6.64964930633648));
#43108=CARTESIAN_POINT('Ctrl Pts',(-42.6214924287507,-48.1210196628927,
-6.84551186414177));
#43109=CARTESIAN_POINT('Ctrl Pts',(-45.8975997111081,-49.9877987537274,
-7.04137442194707));
#43110=CARTESIAN_POINT('Ctrl Pts',(-49.2651728575601,-48.2916287586049,
-7.23723697975236));
#43111=CARTESIAN_POINT('Ctrl Pts',(-49.7154901884265,-44.5479844682866,
-7.43309953755765));
#43112=CARTESIAN_POINT('Ctrl Pts',(-46.8460557375769,-42.1016438677899,
-7.62896209536295));
#43113=CARTESIAN_POINT('Ctrl Pts',(-43.2209153108962,-43.1383685157623,
-7.82482465316823));
#43114=CARTESIAN_POINT('Ctrl Pts',(-42.0783463263615,-46.7317822842778,
-8.02068721097354));
#43115=CARTESIAN_POINT('Ctrl Pts',(-44.4405117122176,-49.6715173106087,
-8.21654976877882));
#43116=CARTESIAN_POINT('Ctrl Pts',(-48.1942059677658,-49.330604929893,-8.41241232658413));
#43117=CARTESIAN_POINT('Ctrl Pts',(-49.9911797286376,-46.0145236824768,
-8.60827488438941));
#43118=CARTESIAN_POINT('Ctrl Pts',(-48.2145202019254,-42.6842505154911,
-8.80413744219471));
#43119=CARTESIAN_POINT('Ctrl Pts',(-45.723514902722,-42.4431146967252,-8.93471248073157));
#43120=CARTESIAN_POINT('Ctrl Pts',(-44.696617959125,-42.8708467090881,-9.));
#43121=CARTESIAN_POINT('Ctrl Pts',(-49.3881103126091,-45.9972329022571,
-1.10898219675043));
#43122=CARTESIAN_POINT('Ctrl Pts',(-49.3906987648108,-45.6759065142304,
-1.12782069376304));
#43123=CARTESIAN_POINT('Ctrl Pts',(-49.348599621807,-45.3552439043751,-1.14665919077565));
#43124=CARTESIAN_POINT('Ctrl Pts',(-49.2590238597979,-45.0484442164888,
-1.16549768778826));
#43125=CARTESIAN_POINT('Ctrl Pts',(-48.9485861808133,-43.9851857983139,
-1.23078520705669));
#43126=CARTESIAN_POINT('Ctrl Pts',(-48.0679217128803,-43.0884305904677,
-1.29607272632512));
#43127=CARTESIAN_POINT('Ctrl Pts',(-47.0104683372979,-42.7587677971901,
-1.36136024559355));
#43128=CARTESIAN_POINT('Ctrl Pts',(-45.9530149617154,-42.4291050039126,
-1.42664776486198));
#43129=CARTESIAN_POINT('Ctrl Pts',(-44.7187726784834,-42.6665346252038,
-1.49193528413041));
#43130=CARTESIAN_POINT('Ctrl Pts',(-43.859106773023,-43.3649988177818,-1.55722280339884));
#43131=CARTESIAN_POINT('Ctrl Pts',(-42.9994408675627,-44.0634630103597,
-1.62251032266727));
#43132=CARTESIAN_POINT('Ctrl Pts',(-42.5143513398739,-45.2229617742244,
-1.6877978419357));
#43133=CARTESIAN_POINT('Ctrl Pts',(-42.6205469192844,-46.3255067438617,
-1.75308536120414));
#43134=CARTESIAN_POINT('Ctrl Pts',(-42.7267424986948,-47.4280517134991,
-1.81837288047257));
#43135=CARTESIAN_POINT('Ctrl Pts',(-43.4242231852045,-48.4736428889091,
-1.883660399741));
#43136=CARTESIAN_POINT('Ctrl Pts',(-44.4014007665572,-48.9951846979414,
-1.94894791900943));
#43137=CARTESIAN_POINT('Ctrl Pts',(-45.3785783479099,-49.5167265069737,
-2.01423543827786));
#43138=CARTESIAN_POINT('Ctrl Pts',(-46.6354528241056,-49.5142189496283,
-2.07952295754629));
#43139=CARTESIAN_POINT('Ctrl Pts',(-47.6105406675939,-48.9887811419861,
-2.14481047681472));
#43140=CARTESIAN_POINT('Ctrl Pts',(-48.5856285110821,-48.4633433343439,
-2.21009799608315));
#43141=CARTESIAN_POINT('Ctrl Pts',(-49.2789297218628,-47.4149752764049,
-2.27538551535158));
#43142=CARTESIAN_POINT('Ctrl Pts',(-49.3807247850927,-46.3120158131135,
-2.34067303462002));
#43143=CARTESIAN_POINT('Ctrl Pts',(-49.3902405513404,-46.2089115553985,
-2.34677608866349));
#43144=CARTESIAN_POINT('Ctrl Pts',(-49.3945874743613,-46.105330253756,-2.35287914270696));
#43145=CARTESIAN_POINT('Ctrl Pts',(-49.393944259473,-46.0016943208402,-2.35898219675043));
#43146=CARTESIAN_POINT('Ctrl Pts',(-47.0579044229729,-49.9456385074984,
5.55111512312578E-16));
#43147=CARTESIAN_POINT('Ctrl Pts',(-47.1733693372504,-49.9039985328978,
5.66013349383169E-16));
#43148=CARTESIAN_POINT('Ctrl Pts',(-47.2864786532175,-49.8568504145239,
5.21146057028503E-16));
#43149=CARTESIAN_POINT('Ctrl Pts',(-47.3970077281708,-49.804548304315,4.47558656802016E-16));
#43150=CARTESIAN_POINT('Ctrl Pts',(-47.5098934841488,-49.7511310179344,
3.72402239284464E-16));
#43151=CARTESIAN_POINT('Ctrl Pts',(-47.620088418098,-49.6923370616094,4.47268168963809E-16));
#43152=CARTESIAN_POINT('Ctrl Pts',(-47.7273259226398,-49.6284969725913,
5.48172618408671E-16));
#43153=CARTESIAN_POINT('Ctrl Pts',(-47.8392942950329,-49.561840527243,6.53528547939391E-16));
#43154=CARTESIAN_POINT('Ctrl Pts',(-47.9480394609077,-49.4896823744086,
7.20663869194476E-16));
#43155=CARTESIAN_POINT('Ctrl Pts',(-48.0532163752826,-49.4123564527643,
7.42461647718073E-16));
#43156=CARTESIAN_POINT('Ctrl Pts',(-48.1452461753606,-49.3446962713255,
7.61534703926221E-16));
#43157=CARTESIAN_POINT('Ctrl Pts',(-48.2345436748161,-49.2730785145345,
1.00926389872883E-15));
#43158=CARTESIAN_POINT('Ctrl Pts',(-48.3208451029165,-49.1977075112963,
1.01307850997046E-15));
#43159=CARTESIAN_POINT('Ctrl Pts',(-48.3378049250329,-49.1828957192345,
1.01382815142513E-15));
#43160=CARTESIAN_POINT('Ctrl Pts',(-48.3546489363343,-49.1679389353915,
5.86365414716671E-16));
#43161=CARTESIAN_POINT('Ctrl Pts',(-48.3713749781207,-49.1528386522715,
5.82867087928207E-16));
#43162=CARTESIAN_POINT('Ctrl Pts',(-48.3839971030697,-49.1414433883627,
5.80227113784865E-16));
#43163=CARTESIAN_POINT('Ctrl Pts',(-48.3965520031907,-49.1299663623313,
3.88578058618805E-16));
#43164=CARTESIAN_POINT('Ctrl Pts',(-48.4090283192252,-49.1184180896672,
3.88578058618805E-16));
#43165=CARTESIAN_POINT('Ctrl Pts',(-48.4995034915464,-49.034672859391,3.88578058618805E-16));
#43166=CARTESIAN_POINT('Ctrl Pts',(-48.585990505988,-48.9470573638322,2.49245464307548E-16));
#43167=CARTESIAN_POINT('Ctrl Pts',(-48.6682317367018,-48.8558860449089,
3.05311331771918E-16));
#43168=CARTESIAN_POINT('Ctrl Pts',(-48.7501471507582,-48.7650759211444,
3.61155082016356E-16));
#43169=CARTESIAN_POINT('Ctrl Pts',(-48.8278508314432,-48.6707373593851,
2.40491596001199E-16));
#43170=CARTESIAN_POINT('Ctrl Pts',(-48.9010457239218,-48.573152188254,4.16333634234434E-17));
#43171=CARTESIAN_POINT('Ctrl Pts',(-48.9731614105922,-48.4770058399686,
-1.54292848184616E-16));
#43172=CARTESIAN_POINT('Ctrl Pts',(-49.0409006391222,-48.3777072181801,
1.86597674064836E-16));
#43173=CARTESIAN_POINT('Ctrl Pts',(-49.1039319851986,-48.2755084011431,
8.32667268468867E-17));
#43174=CARTESIAN_POINT('Ctrl Pts',(-49.1554910626096,-48.191910682755,-1.25706390486376E-18));
#43175=CARTESIAN_POINT('Ctrl Pts',(-49.2038992954219,-48.1063719477112,
5.41938973494124E-16));
#43176=CARTESIAN_POINT('Ctrl Pts',(-49.2489486618552,-48.0190260212161,
5.55111512312578E-16));
#43177=CARTESIAN_POINT('Ctrl Pts',(-49.2595828404022,-47.998407480907,5.58220970686877E-16));
#43178=CARTESIAN_POINT('Ctrl Pts',(-49.270029742428,-47.9776882326517,9.06864741724049E-16));
#43179=CARTESIAN_POINT('Ctrl Pts',(-49.2802864197024,-47.9568700298176,
9.15933995315754E-16));
#43180=CARTESIAN_POINT('Ctrl Pts',(-49.287528246751,-47.9421711346146,9.2233743028929E-16));
#43181=CARTESIAN_POINT('Ctrl Pts',(-49.2946745182361,-47.9274242550742,
-3.81840268582438E-17));
#43182=CARTESIAN_POINT('Ctrl Pts',(-49.3017191206196,-47.9126411190135,
-2.77555756156289E-17));
#43183=CARTESIAN_POINT('Ctrl Pts',(-49.3523583097563,-47.8063745077476,
4.72079618742721E-17));
#43184=CARTESIAN_POINT('Ctrl Pts',(-49.3978249076527,-47.6980808260915,
-4.96970061520271E-16));
#43185=CARTESIAN_POINT('Ctrl Pts',(-49.4378477716308,-47.5880161091457,
-4.9960036108132E-16));
#43186=CARTESIAN_POINT('Ctrl Pts',(-49.4770644924164,-47.4801683230611,
-5.02177680973382E-16));
#43187=CARTESIAN_POINT('Ctrl Pts',(-49.5110547933194,-47.3706194935391,
4.57968148600611E-17));
#43188=CARTESIAN_POINT('Ctrl Pts',(-49.5395146923287,-47.2595997093103,
2.77555756156289E-17));
#43189=CARTESIAN_POINT('Ctrl Pts',(-49.544975138073,-47.2382989482596,2.42941013489102E-17));
#43190=CARTESIAN_POINT('Ctrl Pts',(-49.5502318456946,-47.2169440218678,
-4.52064932513013E-16));
#43191=CARTESIAN_POINT('Ctrl Pts',(-49.5552824461283,-47.1955365379506,
-4.71844785465692E-16));
#43192=CARTESIAN_POINT('Ctrl Pts',(-49.5824903881121,-47.0802129070123,
-6.35243347783829E-16));
#43193=CARTESIAN_POINT('Ctrl Pts',(-49.6037211273402,-46.9633633041741,
-3.31089260042331E-16));
#43194=CARTESIAN_POINT('Ctrl Pts',(-49.6190592501821,-46.8454242871399,
-4.16333634234434E-16));
#43195=CARTESIAN_POINT('Ctrl Pts',(-49.6275696309687,-46.7799856441651,
-4.63631604903081E-16));
#43196=CARTESIAN_POINT('Ctrl Pts',(-49.634264983748,-46.7142117486677,-2.27956851258612E-16));
#43197=CARTESIAN_POINT('Ctrl Pts',(-49.6391531642022,-46.6481791918392,
-2.22044604925031E-16));
#43198=CARTESIAN_POINT('Ctrl Pts',(-49.6410794249398,-46.6221580735902,
-2.1971479568619E-16));
#43199=CARTESIAN_POINT('Ctrl Pts',(-49.6427250054364,-46.596096810251,4.98233321211434E-16));
#43200=CARTESIAN_POINT('Ctrl Pts',(-49.6440901965306,-46.5700001834423,
5.27355936696949E-16));
#43201=CARTESIAN_POINT('Ctrl Pts',(-49.6449645924009,-46.553285466503,5.46008779378254E-16));
#43202=CARTESIAN_POINT('Ctrl Pts',(-49.6457239151094,-46.5365557747368,
6.58486149275759E-16));
#43203=CARTESIAN_POINT('Ctrl Pts',(-49.646367818249,-46.5198278005682,6.66133814775094E-16));
#43204=CARTESIAN_POINT('Ctrl Pts',(-49.6509450937801,-46.4009146564497,
7.20498314655799E-16));
#43205=CARTESIAN_POINT('Ctrl Pts',(-49.6497056526231,-46.2818992441625,
-3.44821266031896E-16));
#43206=CARTESIAN_POINT('Ctrl Pts',(-49.6428026243385,-46.1632168328176,
-3.88578058618805E-16));
#43207=CARTESIAN_POINT('Ctrl Pts',(-49.6360414897975,-46.0469739727774,
-4.31435417673498E-16));
#43208=CARTESIAN_POINT('Ctrl Pts',(-49.6238466714416,-45.9310496539742,
5.18747692508596E-16));
#43209=CARTESIAN_POINT('Ctrl Pts',(-49.6063097059683,-45.8158627002793,
5.55111512312578E-16));
#43210=CARTESIAN_POINT('Ctrl Pts',(-49.5889759985516,-45.7020107937674,
5.91053865851183E-16));
#43211=CARTESIAN_POINT('Ctrl Pts',(-49.56642285937,-45.5888784455779,2.91334207310992E-16));
#43212=CARTESIAN_POINT('Ctrl Pts',(-49.5386937754477,-45.4768924893138,
4.44089209850063E-16));
#43213=CARTESIAN_POINT('Ctrl Pts',(-49.5206040613618,-45.4038358410619,
5.43742495507627E-16));
#43214=CARTESIAN_POINT('Ctrl Pts',(-49.5003106142802,-45.3312675708399,
3.37381644489328E-17));
#43215=CARTESIAN_POINT('Ctrl Pts',(-49.4778162055683,-45.2593138849385,
5.55111512312578E-17));
#43216=CARTESIAN_POINT('Ctrl Pts',(-49.4685898053458,-45.2298010619024,
6.44416500351063E-17));
#43217=CARTESIAN_POINT('Ctrl Pts',(-49.4589930454642,-45.2003917152151,
5.1904603637396E-16));
#43218=CARTESIAN_POINT('Ctrl Pts',(-49.4490257849573,-45.171094919731,5.55111512312578E-16));
#43219=CARTESIAN_POINT('Ctrl Pts',(-49.4429390810481,-45.1532042546404,
5.77135605415197E-16));
#43220=CARTESIAN_POINT('Ctrl Pts',(-49.4367169044357,-45.1353635641357,
-3.8949053638378E-16));
#43221=CARTESIAN_POINT('Ctrl Pts',(-49.430361091836,-45.1175789294473,-3.33066907387547E-16));
#43222=CARTESIAN_POINT('Ctrl Pts',(-49.3921806745662,-45.0107436880449,
5.87916208435275E-18));
#43223=CARTESIAN_POINT('Ctrl Pts',(-49.3491645674419,-44.9058795780642,
7.07363767081224E-16));
#43224=CARTESIAN_POINT('Ctrl Pts',(-49.3013720780751,-44.8033974788009,
3.88578058618805E-16));
#43225=CARTESIAN_POINT('Ctrl Pts',(-49.2629804005143,-44.7210736709641,
1.3249769343093E-16));
#43226=CARTESIAN_POINT('Ctrl Pts',(-49.2215056579415,-44.6402872554315,
-1.03620088217595E-16));
#43227=CARTESIAN_POINT('Ctrl Pts',(-49.1769599094038,-44.5612680076514,
-2.22044604925031E-16));
#43228=CARTESIAN_POINT('Ctrl Pts',(-49.1548834013714,-44.5221067158202,
-2.80734825207282E-16));
#43229=CARTESIAN_POINT('Ctrl Pts',(-49.1320523745914,-44.4833797210652,
-9.37977106089326E-17));
#43230=CARTESIAN_POINT('Ctrl Pts',(-49.1084669149778,-44.4451166907322,
-1.66533453693773E-16));
#43231=CARTESIAN_POINT('Ctrl Pts',(-49.0950715621271,-44.4233852171529,
-2.07843691418425E-16));
#43232=CARTESIAN_POINT('Ctrl Pts',(-49.0814310539731,-44.4018008856244,
5.69071523681598E-16));
#43233=CARTESIAN_POINT('Ctrl Pts',(-49.0675590494629,-44.3803899179501,
5.55111512312578E-16));
#43234=CARTESIAN_POINT('Ctrl Pts',(-49.0090087392671,-44.2900195033499,
4.96189746868475E-16));
#43235=CARTESIAN_POINT('Ctrl Pts',(-48.9462914113485,-44.2026580989667,
1.12926594395583E-15));
#43236=CARTESIAN_POINT('Ctrl Pts',(-48.8794389832423,-44.1186868190207,
1.0547118733939E-15));
#43237=CARTESIAN_POINT('Ctrl Pts',(-48.8212020338695,-44.0455371770777,
9.89765815997824E-16));
#43238=CARTESIAN_POINT('Ctrl Pts',(-48.7598264591088,-43.9749604010674,
8.04362549974418E-16));
#43239=CARTESIAN_POINT('Ctrl Pts',(-48.6953138444556,-43.9072342030353,
9.99200722162641E-16));
#43240=CARTESIAN_POINT('Ctrl Pts',(-48.6572944668562,-43.8673209564524,
1.05974870095357E-15));
#43241=CARTESIAN_POINT('Ctrl Pts',(-48.6181851531445,-43.8283982895143,
2.13352833165291E-16));
#43242=CARTESIAN_POINT('Ctrl Pts',(-48.5780349767684,-43.7904875157198,
2.77555756156289E-16));
#43243=CARTESIAN_POINT('Origin',(-46.,-46.,-5.));
#43244=CARTESIAN_POINT('Origin',(0.,0.,0.));
#43245=CARTESIAN_POINT('',(-40.,-4.89858719658941E-15,4.));
#43246=CARTESIAN_POINT('Origin',(0.,0.,4.));
#43247=CARTESIAN_POINT('',(-40.,-4.89858719658941E-15,0.));
#43248=CARTESIAN_POINT('',(-40.,-4.89858719658941E-15,0.));
#43249=CARTESIAN_POINT('Origin',(0.,0.,0.));
#43250=CARTESIAN_POINT('Origin',(0.,0.,4.));
#43251=CARTESIAN_POINT('',(-20.,-2.44929359829471E-15,4.));
#43252=CARTESIAN_POINT('Origin',(0.,0.,4.));
#43253=CARTESIAN_POINT('Origin',(0.,0.,-10.));
#43254=CARTESIAN_POINT('',(-20.,-2.44929359829471E-15,-10.));
#43255=CARTESIAN_POINT('',(-20.,-2.44929359829471E-15,-10.));
#43256=CARTESIAN_POINT('Origin',(0.,0.,-10.));
#43257=CARTESIAN_POINT('Origin',(0.,0.,-10.));
#43258=CARTESIAN_POINT('',(-110.,1.34711147906209E-14,0.));
#43259=CARTESIAN_POINT('Origin',(0.,0.,0.));
#43260=CARTESIAN_POINT('',(-110.,1.34711147906209E-14,-10.));
#43261=CARTESIAN_POINT('',(-110.,-1.34711147906209E-14,-10.));
#43262=CARTESIAN_POINT('Origin',(0.,0.,-10.));
#43263=CARTESIAN_POINT('Origin',(0.,0.,0.));
#43264=CARTESIAN_POINT('Origin',(0.,0.,-10.));
#69468=UNCERTAINTY_MEASURE_WITH_UNIT(LENGTH_MEASURE(0.01),#69492,
'DISTANCE_ACCURACY_VALUE',
'Maximum model space distance between geometric entities at asserted c
onnectivities');
#69478=UNCERTAINTY_MEASURE_WITH_UNIT(LENGTH_MEASURE(0.01),#69492,
'DISTANCE_ACCURACY_VALUE',
'Maximum model space distance between geometric entities at asserted c
onnectivities');
#69481=(
GEOMETRIC_REPRESENTATION_CONTEXT(3)
GLOBAL_UNCERTAINTY_ASSIGNED_CONTEXT((#69468))
GLOBAL_UNIT_ASSIGNED_CONTEXT((#69492,#69494,#69495))
REPRESENTATION_CONTEXT('','3D')
);
#69491=(
GEOMETRIC_REPRESENTATION_CONTEXT(3)
GLOBAL_UNCERTAINTY_ASSIGNED_CONTEXT((#69478))
GLOBAL_UNIT_ASSIGNED_CONTEXT((#69492,#69494,#69495))
REPRESENTATION_CONTEXT('','3D')
);
#69492=(
LENGTH_UNIT()
NAMED_UNIT(*)
SI_UNIT(.MILLI.,.METRE.)
);
#69494=(
NAMED_UNIT(*)
PLANE_ANGLE_UNIT()
SI_UNIT($,.RADIAN.)
);
#69495=(
NAMED_UNIT(*)
SI_UNIT($,.STERADIAN.)
SOLID_ANGLE_UNIT()
);
#69498=SHAPE_DEFINITION_REPRESENTATION(#69510,#69572);
#69510=PRODUCT_DEFINITION_SHAPE('',$,#69585);
#69572=SHAPE_REPRESENTATION('',(#15193),#69481);
#69582=PRODUCT_DEFINITION_CONTEXT('part definition',#69620,'design');
#69585=PRODUCT_DEFINITION('Backplate','Backplate',#69597,#69582);
#69597=PRODUCT_DEFINITION_FORMATION('',$,#69624);
#69620=APPLICATION_CONTEXT(
'Core Data for Automotive Mechanical Design Process');
#69621=PRODUCT_CONTEXT('part definition',#69620,'mechanical');
#69624=PRODUCT('Backplate','Backplate',$,(#69621));
#69636=PRESENTATION_STYLE_ASSIGNMENT((#69646));
#69646=SURFACE_STYLE_USAGE(.BOTH.,#69656);
#69656=SURFACE_SIDE_STYLE('',(#69666));
#69666=SURFACE_STYLE_FILL_AREA(#69676);
#69676=FILL_AREA_STYLE('Gray',(#69686));
#69686=FILL_AREA_STYLE_COLOUR('Gray',#69696);
#69696=COLOUR_RGB('Gray',0.407843137254902,0.447058823529412,0.498039215686275);
ENDSEC;
END-ISO-10303-21;
